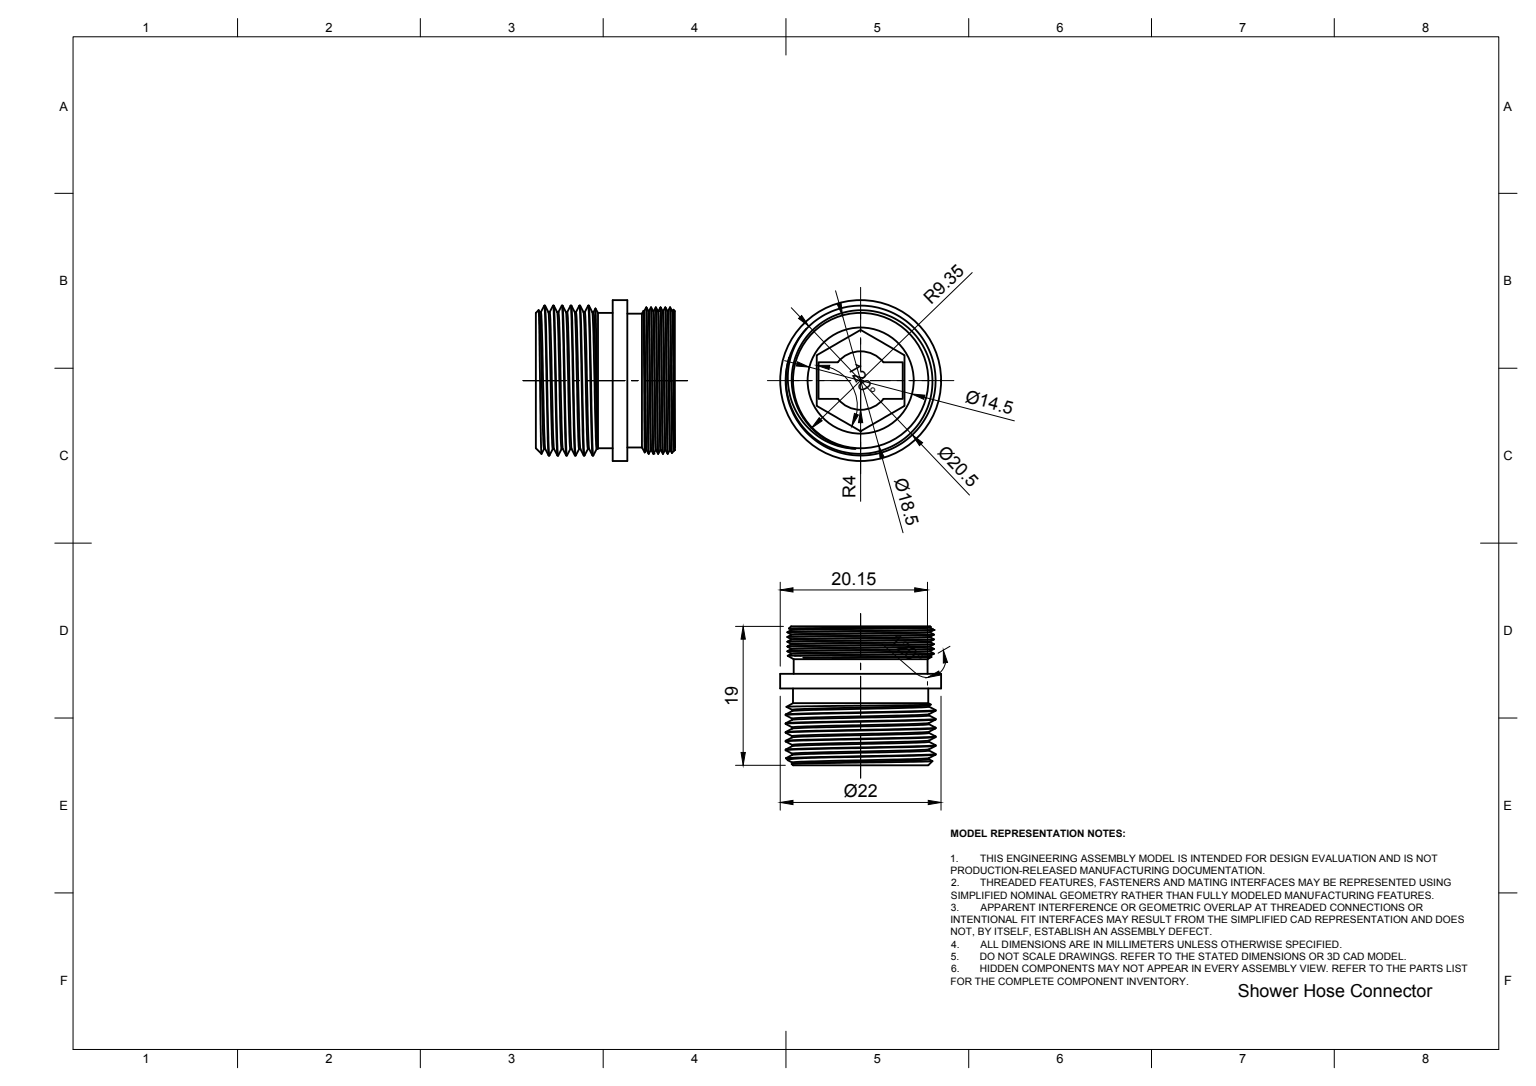
ISO-10303-21;
HEADER;
/* Generated by software containing ST-Developer
 * from STEP Tools, Inc. (www.steptools.com) 
 */

FILE_DESCRIPTION(
/* description */ ('STEP AP214'),
/* implementation_level */ '2;1');

FILE_NAME(
/* name */ 'Shower Hose Connector.step',
/* time_stamp */ '2026-10-05T23:18:41-07:00',
/* author */ (''),
/* organization */ (''),
/* preprocessor_version */ 'ST-DEVELOPER v20.2',
/* originating_system */ 'Autodesk Translation Framework v15.15.0.0',
/* authorisation */ '');

FILE_SCHEMA (('AUTOMOTIVE_DESIGN { 1 0 10303 214 3 1 1 }'));
ENDSEC;

DATA;
#10=MECHANICAL_DESIGN_GEOMETRIC_PRESENTATION_REPRESENTATION('',(#102),#221662);
#64=MANIFOLD_SOLID_BREP('Body1',#79324);
#76=SHAPE_REPRESENTATION_RELATIONSHIP('SRR','None',#221711,#89);
#89=ADVANCED_BREP_SHAPE_REPRESENTATION('',(#64),#221651);
#102=STYLED_ITEM('',(#221783),#64);
#179=B_SPLINE_SURFACE_WITH_KNOTS('',1,3,((#174040,#174041,#174042,#174043,
#174044,#174045,#174046,#174047,#174048,#174049,#174050,#174051,#174052,
#174053,#174054,#174055,#174056,#174057,#174058,#174059,#174060,#174061,
#174062,#174063,#174064,#174065,#174066,#174067,#174068,#174069,#174070,
#174071,#174072,#174073,#174074,#174075,#174076,#174077,#174078,#174079,
#174080,#174081,#174082,#174083,#174084,#174085,#174086,#174087,#174088,
#174089,#174090,#174091,#174092,#174093,#174094,#174095,#174096,#174097,
#174098,#174099,#174100,#174101,#174102,#174103,#174104,#174105,#174106),
(#174107,#174108,#174109,#174110,#174111,#174112,#174113,#174114,#174115,
#174116,#174117,#174118,#174119,#174120,#174121,#174122,#174123,#174124,
#174125,#174126,#174127,#174128,#174129,#174130,#174131,#174132,#174133,
#174134,#174135,#174136,#174137,#174138,#174139,#174140,#174141,#174142,
#174143,#174144,#174145,#174146,#174147,#174148,#174149,#174150,#174151,
#174152,#174153,#174154,#174155,#174156,#174157,#174158,#174159,#174160,
#174161,#174162,#174163,#174164,#174165,#174166,#174167,#174168,#174169,
#174170,#174171,#174172,#174173)),.UNSPECIFIED.,.F.,.F.,.F.,(2,2),(4,1,
1,1,1,1,1,1,1,1,1,1,1,1,1,1,1,1,1,1,1,1,1,1,1,1,1,1,1,1,1,1,1,1,1,1,1,1,
1,1,1,1,1,1,1,1,1,1,1,1,1,1,1,1,1,1,1,1,1,1,1,1,1,1,4),(0.,1.),(0.,0.0157026587679609,
0.0314053175359218,0.0471079763038827,0.0628106350718436,0.0785132938398045,
0.0942159526077654,0.109918611375726,0.125621270143687,0.141323928911648,
0.157026587679609,0.17272924644757,0.188431905215531,0.204134563983492,
0.219837222751453,0.235539881519413,0.251242540287374,0.266945199055335,
0.282647857823296,0.298350516591257,0.314053175359218,0.329755834127179,
0.34545849289514,0.361161151663101,0.376863810431061,0.392566469199022,
0.408269127966983,0.423971786734944,0.439674445502905,0.455377104270866,
0.471079763038827,0.486782421806788,0.502485080574749,0.518187739342709,
0.53389039811067,0.549593056878631,0.565295715646592,0.580998374414553,
0.596701033182514,0.612403691950475,0.628106350718436,0.643809009486397,
0.659511668254358,0.675214327022318,0.690916985790279,0.70661964455824,
0.722322303326201,0.738024962094162,0.753727620862123,0.769430279630084,
0.785132938398045,0.800835597166006,0.816538255933966,0.832240914701927,
0.847943573469888,0.863646232237849,0.87934889100581,0.895051549773771,
0.910754208541732,0.926456867309693,0.942159526077654,0.957862184845615,
0.973564843613575,0.989267502381536,1.),.UNSPECIFIED.);
#180=B_SPLINE_SURFACE_WITH_KNOTS('',1,3,((#174174,#174175,#174176,#174177,
#174178,#174179,#174180,#174181,#174182,#174183,#174184,#174185,#174186,
#174187,#174188,#174189,#174190,#174191,#174192,#174193,#174194,#174195,
#174196,#174197,#174198,#174199,#174200,#174201,#174202,#174203,#174204,
#174205,#174206,#174207,#174208,#174209,#174210,#174211,#174212,#174213,
#174214,#174215,#174216,#174217,#174218,#174219,#174220,#174221,#174222,
#174223,#174224,#174225,#174226,#174227,#174228,#174229,#174230,#174231,
#174232,#174233,#174234,#174235,#174236,#174237,#174238,#174239,#174240),
(#174241,#174242,#174243,#174244,#174245,#174246,#174247,#174248,#174249,
#174250,#174251,#174252,#174253,#174254,#174255,#174256,#174257,#174258,
#174259,#174260,#174261,#174262,#174263,#174264,#174265,#174266,#174267,
#174268,#174269,#174270,#174271,#174272,#174273,#174274,#174275,#174276,
#174277,#174278,#174279,#174280,#174281,#174282,#174283,#174284,#174285,
#174286,#174287,#174288,#174289,#174290,#174291,#174292,#174293,#174294,
#174295,#174296,#174297,#174298,#174299,#174300,#174301,#174302,#174303,
#174304,#174305,#174306,#174307)),.UNSPECIFIED.,.F.,.F.,.F.,(2,2),(4,1,
1,1,1,1,1,1,1,1,1,1,1,1,1,1,1,1,1,1,1,1,1,1,1,1,1,1,1,1,1,1,1,1,1,1,1,1,
1,1,1,1,1,1,1,1,1,1,1,1,1,1,1,1,1,1,1,1,1,1,1,1,1,1,4),(0.,1.),(0.,0.0157026587679609,
0.0314053175359218,0.0471079763038827,0.0628106350718436,0.0785132938398045,
0.0942159526077654,0.109918611375726,0.125621270143687,0.141323928911648,
0.157026587679609,0.17272924644757,0.188431905215531,0.204134563983492,
0.219837222751453,0.235539881519413,0.251242540287374,0.266945199055335,
0.282647857823296,0.298350516591257,0.314053175359218,0.329755834127179,
0.34545849289514,0.361161151663101,0.376863810431061,0.392566469199022,
0.408269127966983,0.423971786734944,0.439674445502905,0.455377104270866,
0.471079763038827,0.486782421806788,0.502485080574749,0.518187739342709,
0.53389039811067,0.549593056878631,0.565295715646592,0.580998374414553,
0.596701033182514,0.612403691950475,0.628106350718436,0.643809009486397,
0.659511668254358,0.675214327022318,0.690916985790279,0.70661964455824,
0.722322303326201,0.738024962094162,0.753727620862123,0.769430279630084,
0.785132938398045,0.800835597166006,0.816538255933966,0.832240914701927,
0.847943573469888,0.863646232237849,0.87934889100581,0.895051549773771,
0.910754208541732,0.926456867309693,0.942159526077654,0.957862184845615,
0.973564843613575,0.989267502381536,1.),.UNSPECIFIED.);
#181=B_SPLINE_SURFACE_WITH_KNOTS('',1,3,((#174308,#174309,#174310,#174311,
#174312,#174313,#174314,#174315,#174316,#174317,#174318,#174319,#174320,
#174321,#174322,#174323,#174324,#174325,#174326,#174327,#174328,#174329,
#174330,#174331,#174332,#174333,#174334,#174335,#174336,#174337,#174338,
#174339,#174340,#174341,#174342,#174343,#174344,#174345,#174346,#174347,
#174348,#174349,#174350,#174351,#174352,#174353,#174354,#174355,#174356,
#174357,#174358,#174359,#174360,#174361,#174362,#174363,#174364,#174365,
#174366,#174367,#174368,#174369,#174370,#174371,#174372,#174373,#174374,
#174375,#174376,#174377,#174378,#174379,#174380,#174381,#174382,#174383,
#174384),(#174385,#174386,#174387,#174388,#174389,#174390,#174391,#174392,
#174393,#174394,#174395,#174396,#174397,#174398,#174399,#174400,#174401,
#174402,#174403,#174404,#174405,#174406,#174407,#174408,#174409,#174410,
#174411,#174412,#174413,#174414,#174415,#174416,#174417,#174418,#174419,
#174420,#174421,#174422,#174423,#174424,#174425,#174426,#174427,#174428,
#174429,#174430,#174431,#174432,#174433,#174434,#174435,#174436,#174437,
#174438,#174439,#174440,#174441,#174442,#174443,#174444,#174445,#174446,
#174447,#174448,#174449,#174450,#174451,#174452,#174453,#174454,#174455,
#174456,#174457,#174458,#174459,#174460,#174461)),.UNSPECIFIED.,.F.,.F.,
 .F.,(2,2),(4,1,1,1,1,1,1,1,1,1,1,1,1,1,1,1,1,1,1,1,1,1,1,1,1,1,1,1,1,1,
1,1,1,1,1,1,1,1,1,1,1,1,1,1,1,1,1,1,1,1,1,1,1,1,1,1,1,1,1,1,1,1,1,1,1,1,
1,1,1,1,1,1,1,1,4),(0.,1.),(0.,0.0135337770704249,0.0270675541408498,0.0406013312112747,
0.0541351082816996,0.0676688853521246,0.0812026624225494,0.0947364394929744,
0.108270216563399,0.121803993633824,0.135337770704249,0.148871547774674,
0.162405324845099,0.175939101915524,0.189472878985949,0.203006656056374,
0.216540433126799,0.230074210197223,0.243607987267648,0.257141764338073,
0.270675541408498,0.284209318478923,0.297743095549348,0.311276872619773,
0.324810649690198,0.338344426760623,0.351878203831048,0.365411980901473,
0.378945757971897,0.392479535042322,0.406013312112747,0.419547089183172,
0.433080866253597,0.446614643324022,0.460148420394447,0.473682197464872,
0.487215974535297,0.500749751605722,0.514283528676147,0.527817305746571,
0.541351082816996,0.554884859887421,0.568418636957846,0.581952414028271,
0.595486191098696,0.609019968169121,0.622553745239546,0.636087522309971,
0.649621299380396,0.663155076450821,0.676688853521245,0.69022263059167,
0.703756407662095,0.71729018473252,0.730823961802945,0.74435773887337,0.757891515943795,
0.77142529301422,0.784959070084645,0.79849284715507,0.812026624225495,0.825560401295919,
0.839094178366344,0.852627955436769,0.866161732507194,0.879695509577619,
0.893229286648044,0.906763063718469,0.920296840788894,0.933830617859319,
0.947364394929744,0.960898172000169,0.974431949070593,0.987965726141018,
1.),.UNSPECIFIED.);
#182=B_SPLINE_SURFACE_WITH_KNOTS('',1,3,((#174462,#174463,#174464,#174465,
#174466,#174467,#174468,#174469,#174470,#174471,#174472,#174473,#174474,
#174475,#174476,#174477,#174478,#174479,#174480,#174481,#174482,#174483,
#174484,#174485,#174486,#174487,#174488,#174489,#174490,#174491,#174492,
#174493,#174494,#174495,#174496,#174497,#174498,#174499,#174500,#174501,
#174502,#174503,#174504,#174505,#174506,#174507,#174508,#174509,#174510,
#174511,#174512,#174513,#174514,#174515,#174516,#174517,#174518,#174519,
#174520,#174521,#174522,#174523,#174524,#174525,#174526,#174527,#174528,
#174529,#174530,#174531,#174532,#174533,#174534,#174535,#174536,#174537,
#174538),(#174539,#174540,#174541,#174542,#174543,#174544,#174545,#174546,
#174547,#174548,#174549,#174550,#174551,#174552,#174553,#174554,#174555,
#174556,#174557,#174558,#174559,#174560,#174561,#174562,#174563,#174564,
#174565,#174566,#174567,#174568,#174569,#174570,#174571,#174572,#174573,
#174574,#174575,#174576,#174577,#174578,#174579,#174580,#174581,#174582,
#174583,#174584,#174585,#174586,#174587,#174588,#174589,#174590,#174591,
#174592,#174593,#174594,#174595,#174596,#174597,#174598,#174599,#174600,
#174601,#174602,#174603,#174604,#174605,#174606,#174607,#174608,#174609,
#174610,#174611,#174612,#174613,#174614,#174615)),.UNSPECIFIED.,.F.,.F.,
 .F.,(2,2),(4,1,1,1,1,1,1,1,1,1,1,1,1,1,1,1,1,1,1,1,1,1,1,1,1,1,1,1,1,1,
1,1,1,1,1,1,1,1,1,1,1,1,1,1,1,1,1,1,1,1,1,1,1,1,1,1,1,1,1,1,1,1,1,1,1,1,
1,1,1,1,1,1,1,1,4),(0.,1.),(0.,0.0135337770704249,0.0270675541408498,0.0406013312112747,
0.0541351082816996,0.0676688853521246,0.0812026624225494,0.0947364394929744,
0.108270216563399,0.121803993633824,0.135337770704249,0.148871547774674,
0.162405324845099,0.175939101915524,0.189472878985949,0.203006656056374,
0.216540433126799,0.230074210197223,0.243607987267648,0.257141764338073,
0.270675541408498,0.284209318478923,0.297743095549348,0.311276872619773,
0.324810649690198,0.338344426760623,0.351878203831048,0.365411980901473,
0.378945757971897,0.392479535042322,0.406013312112747,0.419547089183172,
0.433080866253597,0.446614643324022,0.460148420394447,0.473682197464872,
0.487215974535297,0.500749751605722,0.514283528676147,0.527817305746571,
0.541351082816996,0.554884859887421,0.568418636957846,0.581952414028271,
0.595486191098696,0.609019968169121,0.622553745239546,0.636087522309971,
0.649621299380396,0.663155076450821,0.676688853521245,0.69022263059167,
0.703756407662095,0.71729018473252,0.730823961802945,0.74435773887337,0.757891515943795,
0.77142529301422,0.784959070084645,0.79849284715507,0.812026624225495,0.825560401295919,
0.839094178366344,0.852627955436769,0.866161732507194,0.879695509577619,
0.893229286648044,0.906763063718469,0.920296840788894,0.933830617859319,
0.947364394929744,0.960898172000169,0.974431949070593,0.987965726141018,
1.),.UNSPECIFIED.);
#275=FACE_BOUND('',#24701,.T.);
#276=FACE_BOUND('',#24703,.T.);
#277=FACE_BOUND('',#24705,.T.);
#278=FACE_BOUND('',#24713,.T.);
#279=FACE_BOUND('',#24715,.T.);
#280=FACE_BOUND('',#24717,.T.);
#281=FACE_BOUND('',#24719,.T.);
#1770=(
BOUNDED_CURVE()
B_SPLINE_CURVE(2,(#173205,#173206,#173207),.UNSPECIFIED.,.F.,.F.)
B_SPLINE_CURVE_WITH_KNOTS((3,3),(-1.84750056124993,-0.734340623816359),
 .UNSPECIFIED.)
CURVE()
GEOMETRIC_REPRESENTATION_ITEM()
RATIONAL_B_SPLINE_CURVE((1.51230430780121,1.74625859842863,1.51230430780121))
REPRESENTATION_ITEM('')
);
#1771=(
BOUNDED_CURVE()
B_SPLINE_CURVE(2,(#173209,#173210,#173211),.UNSPECIFIED.,.F.,.F.)
B_SPLINE_CURVE_WITH_KNOTS((3,3),(-1.84750056124992,-0.734340623816352),
 .UNSPECIFIED.)
CURVE()
GEOMETRIC_REPRESENTATION_ITEM()
RATIONAL_B_SPLINE_CURVE((1.51230430780122,1.74625859842863,1.51230430780121))
REPRESENTATION_ITEM('')
);
#1772=(
BOUNDED_CURVE()
B_SPLINE_CURVE(2,(#173213,#173214,#173215),.UNSPECIFIED.,.F.,.F.)
B_SPLINE_CURVE_WITH_KNOTS((3,3),(-1.84750056124992,-0.734340623816351),
 .UNSPECIFIED.)
CURVE()
GEOMETRIC_REPRESENTATION_ITEM()
RATIONAL_B_SPLINE_CURVE((1.51230430780122,1.74625859842864,1.51230430780121))
REPRESENTATION_ITEM('')
);
#1773=(
BOUNDED_CURVE()
B_SPLINE_CURVE(2,(#173220,#173221,#173222),.UNSPECIFIED.,.F.,.F.)
B_SPLINE_CURVE_WITH_KNOTS((3,3),(0.734340623816355,1.8475005612499),
 .UNSPECIFIED.)
CURVE()
GEOMETRIC_REPRESENTATION_ITEM()
RATIONAL_B_SPLINE_CURVE((1.5123043078012,1.7462585984286,1.5123043078012))
REPRESENTATION_ITEM('')
);
#1774=(
BOUNDED_CURVE()
B_SPLINE_CURVE(2,(#173224,#173225,#173226),.UNSPECIFIED.,.F.,.F.)
B_SPLINE_CURVE_WITH_KNOTS((3,3),(0.734340623816354,1.84750056124992),
 .UNSPECIFIED.)
CURVE()
GEOMETRIC_REPRESENTATION_ITEM()
RATIONAL_B_SPLINE_CURVE((1.51230430780121,1.74625859842862,1.51230430780121))
REPRESENTATION_ITEM('')
);
#1775=(
BOUNDED_CURVE()
B_SPLINE_CURVE(2,(#173227,#173228,#173229),.UNSPECIFIED.,.F.,.F.)
B_SPLINE_CURVE_WITH_KNOTS((3,3),(0.734340623816358,1.84750056124993),
 .UNSPECIFIED.)
CURVE()
GEOMETRIC_REPRESENTATION_ITEM()
RATIONAL_B_SPLINE_CURVE((1.51230430780122,1.74625859842864,1.51230430780122))
REPRESENTATION_ITEM('')
);
#1886=TOROIDAL_SURFACE('',#80583,6.75,0.25);
#1887=TOROIDAL_SURFACE('',#80586,8.25,0.5);
#1933=CONICAL_SURFACE('',#80540,9.49999999999999,0.7853981625);
#1934=CONICAL_SURFACE('',#80555,7.25,1.04719755);
#1935=CONICAL_SURFACE('',#80571,10.25,1.04719755);
#1936=CONICAL_SURFACE('',#80573,9.99999999999999,1.04719755);
#1937=CONICAL_SURFACE('',#80592,9.49999999999999,0.7853981625);
#1938=CONICAL_SURFACE('',#80594,10.25,0.7853981625);
#2170=CYLINDRICAL_SURFACE('',#80523,9.35);
#2171=CYLINDRICAL_SURFACE('',#80525,9.35);
#2172=CYLINDRICAL_SURFACE('',#80526,9.35);
#2173=CYLINDRICAL_SURFACE('',#80527,9.35);
#2174=CYLINDRICAL_SURFACE('',#80528,9.35);
#2175=CYLINDRICAL_SURFACE('',#80529,9.35);
#2176=CYLINDRICAL_SURFACE('',#80530,9.35);
#2177=CYLINDRICAL_SURFACE('',#80532,9.50000000000001);
#2178=CYLINDRICAL_SURFACE('',#80534,9.50000000000001);
#2179=CYLINDRICAL_SURFACE('',#80535,9.50000000000001);
#2180=CYLINDRICAL_SURFACE('',#80536,9.50000000000001);
#2181=CYLINDRICAL_SURFACE('',#80537,9.50000000000001);
#2182=CYLINDRICAL_SURFACE('',#80538,9.50000000000001);
#2183=CYLINDRICAL_SURFACE('',#80539,9.50000000000001);
#2184=CYLINDRICAL_SURFACE('',#80542,10.);
#2185=CYLINDRICAL_SURFACE('',#80544,10.);
#2186=CYLINDRICAL_SURFACE('',#80545,10.);
#2187=CYLINDRICAL_SURFACE('',#80546,10.);
#2188=CYLINDRICAL_SURFACE('',#80547,10.);
#2189=CYLINDRICAL_SURFACE('',#80548,10.25);
#2190=CYLINDRICAL_SURFACE('',#80550,10.25);
#2191=CYLINDRICAL_SURFACE('',#80551,10.25);
#2192=CYLINDRICAL_SURFACE('',#80552,10.25);
#2193=CYLINDRICAL_SURFACE('',#80553,10.25);
#2194=CYLINDRICAL_SURFACE('',#80554,10.25);
#2195=CYLINDRICAL_SURFACE('',#80557,10.25);
#2196=CYLINDRICAL_SURFACE('',#80559,9.25);
#2197=CYLINDRICAL_SURFACE('',#80563,11.);
#2198=CYLINDRICAL_SURFACE('',#80566,9.15);
#2199=CYLINDRICAL_SURFACE('',#80569,10.);
#2200=CYLINDRICAL_SURFACE('',#80576,7.75);
#2201=CYLINDRICAL_SURFACE('',#80580,6.5);
#2202=CYLINDRICAL_SURFACE('',#80589,4.);
#2203=CYLINDRICAL_SURFACE('',#80596,9.50000000000001);
#2204=CYLINDRICAL_SURFACE('',#80597,9.35);
#2205=CYLINDRICAL_SURFACE('',#80601,4.);
#3041=LINE('',#161941,#10108);
#3042=LINE('',#162330,#10109);
#3043=LINE('',#162956,#10110);
#3044=LINE('',#163166,#10111);
#3045=LINE('',#163572,#10112);
#3046=LINE('',#163993,#10113);
#3047=LINE('',#164421,#10114);
#3048=LINE('',#164833,#10115);
#3049=LINE('',#165106,#10116);
#3050=LINE('',#165636,#10117);
#3051=LINE('',#166150,#10118);
#3052=LINE('',#166686,#10119);
#3053=LINE('',#167210,#10120);
#3054=LINE('',#167730,#10121);
#3055=LINE('',#168256,#10122);
#3056=LINE('',#168283,#10123);
#3057=LINE('',#168630,#10124);
#3058=LINE('',#169158,#10125);
#3059=LINE('',#169674,#10126);
#3060=LINE('',#170192,#10127);
#3061=LINE('',#170718,#10128);
#3062=LINE('',#171017,#10129);
#3063=LINE('',#171447,#10130);
#3064=LINE('',#171891,#10131);
#3065=LINE('',#172549,#10132);
#3066=LINE('',#172769,#10133);
#3067=LINE('',#173217,#10134);
#3068=LINE('',#173296,#10135);
#3069=LINE('',#173304,#10136);
#3070=LINE('',#173310,#10137);
#3071=LINE('',#173726,#10138);
#3072=LINE('',#173793,#10139);
#3073=LINE('',#173799,#10140);
#3074=LINE('',#173806,#10141);
#3075=LINE('',#173821,#10142);
#3076=LINE('',#173824,#10143);
#3077=LINE('',#173948,#10144);
#3078=LINE('',#174618,#10145);
#3079=LINE('',#174620,#10146);
#3080=LINE('',#174621,#10147);
#3081=LINE('',#174624,#10148);
#3082=LINE('',#174626,#10149);
#3083=LINE('',#174627,#10150);
#3084=LINE('',#174630,#10151);
#3085=LINE('',#174632,#10152);
#3086=LINE('',#174633,#10153);
#3087=LINE('',#174638,#10154);
#3088=LINE('',#174642,#10155);
#3089=LINE('',#174644,#10156);
#3090=LINE('',#174645,#10157);
#3091=LINE('',#174648,#10158);
#3092=LINE('',#174650,#10159);
#3093=LINE('',#174651,#10160);
#3094=LINE('',#174653,#10161);
#3095=LINE('',#174654,#10162);
#3096=LINE('',#174660,#10163);
#3097=LINE('',#174662,#10164);
#3098=LINE('',#174664,#10165);
#3099=LINE('',#174666,#10166);
#3100=LINE('',#174668,#10167);
#3101=LINE('',#174669,#10168);
#3102=LINE('',#174671,#10169);
#3103=LINE('',#174672,#10170);
#3104=LINE('',#174674,#10171);
#3105=LINE('',#174676,#10172);
#3106=LINE('',#174678,#10173);
#3107=LINE('',#174680,#10174);
#10108=VECTOR('',#88588,9.35000000000001);
#10109=VECTOR('',#88593,9.35000000000001);
#10110=VECTOR('',#88596,9.35000000000001);
#10111=VECTOR('',#88599,9.35000000000001);
#10112=VECTOR('',#88602,9.35000000000001);
#10113=VECTOR('',#88605,9.35000000000001);
#10114=VECTOR('',#88608,9.35000000000001);
#10115=VECTOR('',#88613,9.50000000000001);
#10116=VECTOR('',#88618,9.50000000000001);
#10117=VECTOR('',#88621,9.50000000000001);
#10118=VECTOR('',#88624,9.50000000000001);
#10119=VECTOR('',#88627,9.50000000000001);
#10120=VECTOR('',#88630,9.50000000000001);
#10121=VECTOR('',#88633,9.50000000000001);
#10122=VECTOR('',#88636,9.5);
#10123=VECTOR('',#88641,10.);
#10124=VECTOR('',#88646,10.);
#10125=VECTOR('',#88649,10.);
#10126=VECTOR('',#88652,10.);
#10127=VECTOR('',#88655,10.);
#10128=VECTOR('',#88658,10.25);
#10129=VECTOR('',#88663,10.25);
#10130=VECTOR('',#88666,10.25);
#10131=VECTOR('',#88669,10.25);
#10132=VECTOR('',#88672,10.25);
#10133=VECTOR('',#88675,10.25);
#10134=VECTOR('',#88678,7.25);
#10135=VECTOR('',#88689,9.25000000000001);
#10136=VECTOR('',#88698,11.);
#10137=VECTOR('',#88705,9.15);
#10138=VECTOR('',#88716,10.25);
#10139=VECTOR('',#88723,9.99999999999999);
#10140=VECTOR('',#88728,7.75);
#10141=VECTOR('',#88737,6.5);
#10142=VECTOR('',#88756,1000.);
#10143=VECTOR('',#88759,1000.);
#10144=VECTOR('',#88766,10.25);
#10145=VECTOR('',#88775,1000.);
#10146=VECTOR('',#88776,1000.);
#10147=VECTOR('',#88777,1000.);
#10148=VECTOR('',#88780,1000.);
#10149=VECTOR('',#88781,1000.);
#10150=VECTOR('',#88782,1000.);
#10151=VECTOR('',#88785,1000.);
#10152=VECTOR('',#88786,1000.);
#10153=VECTOR('',#88787,1000.);
#10154=VECTOR('',#88792,1000.);
#10155=VECTOR('',#88797,1000.);
#10156=VECTOR('',#88798,1000.);
#10157=VECTOR('',#88799,1000.);
#10158=VECTOR('',#88802,1000.);
#10159=VECTOR('',#88803,1000.);
#10160=VECTOR('',#88804,1000.);
#10161=VECTOR('',#88807,1000.);
#10162=VECTOR('',#88808,1000.);
#10163=VECTOR('',#88815,1000.);
#10164=VECTOR('',#88816,1000.);
#10165=VECTOR('',#88817,1000.);
#10166=VECTOR('',#88818,1000.);
#10167=VECTOR('',#88819,1000.);
#10168=VECTOR('',#88820,1000.);
#10169=VECTOR('',#88823,1000.);
#10170=VECTOR('',#88824,1000.);
#10171=VECTOR('',#88827,1000.);
#10172=VECTOR('',#88830,1000.);
#10173=VECTOR('',#88833,1000.);
#10174=VECTOR('',#88836,1000.);
#16943=PLANE('',#80598);
#16944=PLANE('',#80599);
#16945=PLANE('',#80600);
#16946=PLANE('',#80604);
#16947=PLANE('',#80605);
#16948=PLANE('',#80606);
#16949=PLANE('',#80607);
#16950=PLANE('',#80608);
#16951=PLANE('',#80609);
#16952=PLANE('',#80610);
#16953=PLANE('',#80611);
#16954=PLANE('',#80612);
#16955=PLANE('',#80613);
#16956=PLANE('',#80614);
#16957=PLANE('',#80615);
#16958=PLANE('',#80616);
#16959=PLANE('',#80617);
#16960=PLANE('',#80618);
#16961=PLANE('',#80619);
#20601=FACE_OUTER_BOUND('',#24646,.T.);
#20602=FACE_OUTER_BOUND('',#24647,.T.);
#20603=FACE_OUTER_BOUND('',#24648,.T.);
#20604=FACE_OUTER_BOUND('',#24649,.T.);
#20605=FACE_OUTER_BOUND('',#24650,.T.);
#20606=FACE_OUTER_BOUND('',#24651,.T.);
#20607=FACE_OUTER_BOUND('',#24652,.T.);
#20608=FACE_OUTER_BOUND('',#24653,.T.);
#20609=FACE_OUTER_BOUND('',#24654,.T.);
#20610=FACE_OUTER_BOUND('',#24655,.T.);
#20611=FACE_OUTER_BOUND('',#24656,.T.);
#20612=FACE_OUTER_BOUND('',#24657,.T.);
#20613=FACE_OUTER_BOUND('',#24658,.T.);
#20614=FACE_OUTER_BOUND('',#24659,.T.);
#20615=FACE_OUTER_BOUND('',#24660,.T.);
#20616=FACE_OUTER_BOUND('',#24661,.T.);
#20617=FACE_OUTER_BOUND('',#24662,.T.);
#20618=FACE_OUTER_BOUND('',#24663,.T.);
#20619=FACE_OUTER_BOUND('',#24664,.T.);
#20620=FACE_OUTER_BOUND('',#24665,.T.);
#20621=FACE_OUTER_BOUND('',#24666,.T.);
#20622=FACE_OUTER_BOUND('',#24667,.T.);
#20623=FACE_OUTER_BOUND('',#24668,.T.);
#20624=FACE_OUTER_BOUND('',#24669,.T.);
#20625=FACE_OUTER_BOUND('',#24670,.T.);
#20626=FACE_OUTER_BOUND('',#24671,.T.);
#20627=FACE_OUTER_BOUND('',#24672,.T.);
#20628=FACE_OUTER_BOUND('',#24673,.T.);
#20629=FACE_OUTER_BOUND('',#24674,.T.);
#20630=FACE_OUTER_BOUND('',#24675,.T.);
#20631=FACE_OUTER_BOUND('',#24676,.T.);
#20632=FACE_OUTER_BOUND('',#24677,.T.);
#20633=FACE_OUTER_BOUND('',#24678,.T.);
#20634=FACE_OUTER_BOUND('',#24679,.T.);
#20635=FACE_OUTER_BOUND('',#24680,.T.);
#20636=FACE_OUTER_BOUND('',#24681,.T.);
#20637=FACE_OUTER_BOUND('',#24682,.T.);
#20638=FACE_OUTER_BOUND('',#24683,.T.);
#20639=FACE_OUTER_BOUND('',#24684,.T.);
#20640=FACE_OUTER_BOUND('',#24685,.T.);
#20641=FACE_OUTER_BOUND('',#24686,.T.);
#20642=FACE_OUTER_BOUND('',#24687,.T.);
#20643=FACE_OUTER_BOUND('',#24688,.T.);
#20644=FACE_OUTER_BOUND('',#24689,.T.);
#20645=FACE_OUTER_BOUND('',#24690,.T.);
#20646=FACE_OUTER_BOUND('',#24691,.T.);
#20647=FACE_OUTER_BOUND('',#24692,.T.);
#20648=FACE_OUTER_BOUND('',#24693,.T.);
#20649=FACE_OUTER_BOUND('',#24694,.T.);
#20650=FACE_OUTER_BOUND('',#24695,.T.);
#20651=FACE_OUTER_BOUND('',#24696,.T.);
#20652=FACE_OUTER_BOUND('',#24697,.T.);
#20653=FACE_OUTER_BOUND('',#24698,.T.);
#20654=FACE_OUTER_BOUND('',#24699,.T.);
#20655=FACE_OUTER_BOUND('',#24700,.T.);
#20656=FACE_OUTER_BOUND('',#24702,.T.);
#20657=FACE_OUTER_BOUND('',#24704,.T.);
#20658=FACE_OUTER_BOUND('',#24706,.T.);
#20659=FACE_OUTER_BOUND('',#24707,.T.);
#20660=FACE_OUTER_BOUND('',#24708,.T.);
#20661=FACE_OUTER_BOUND('',#24709,.T.);
#20662=FACE_OUTER_BOUND('',#24710,.T.);
#20663=FACE_OUTER_BOUND('',#24711,.T.);
#20664=FACE_OUTER_BOUND('',#24712,.T.);
#20665=FACE_OUTER_BOUND('',#24714,.T.);
#20666=FACE_OUTER_BOUND('',#24716,.T.);
#20667=FACE_OUTER_BOUND('',#24718,.T.);
#24646=EDGE_LOOP('',(#55947,#55948,#55949,#55950));
#24647=EDGE_LOOP('',(#55951,#55952,#55953,#55954));
#24648=EDGE_LOOP('',(#55955,#55956,#55957,#55958));
#24649=EDGE_LOOP('',(#55959,#55960,#55961,#55962));
#24650=EDGE_LOOP('',(#55963,#55964,#55965,#55966,#55967));
#24651=EDGE_LOOP('',(#55968,#55969,#55970,#55971));
#24652=EDGE_LOOP('',(#55972,#55973,#55974,#55975,#55976));
#24653=EDGE_LOOP('',(#55977,#55978,#55979,#55980));
#24654=EDGE_LOOP('',(#55981,#55982,#55983,#55984));
#24655=EDGE_LOOP('',(#55985,#55986,#55987,#55988));
#24656=EDGE_LOOP('',(#55989,#55990,#55991,#55992,#55993,#55994));
#24657=EDGE_LOOP('',(#55995,#55996,#55997,#55998));
#24658=EDGE_LOOP('',(#55999,#56000,#56001,#56002));
#24659=EDGE_LOOP('',(#56003,#56004,#56005,#56006));
#24660=EDGE_LOOP('',(#56007,#56008,#56009));
#24661=EDGE_LOOP('',(#56010,#56011,#56012,#56013));
#24662=EDGE_LOOP('',(#56014,#56015,#56016,#56017));
#24663=EDGE_LOOP('',(#56018,#56019,#56020,#56021));
#24664=EDGE_LOOP('',(#56022,#56023,#56024,#56025));
#24665=EDGE_LOOP('',(#56026,#56027,#56028,#56029));
#24666=EDGE_LOOP('',(#56030,#56031,#56032,#56033));
#24667=EDGE_LOOP('',(#56034,#56035,#56036,#56037));
#24668=EDGE_LOOP('',(#56038,#56039,#56040,#56041));
#24669=EDGE_LOOP('',(#56042,#56043,#56044,#56045));
#24670=EDGE_LOOP('',(#56046,#56047,#56048,#56049));
#24671=EDGE_LOOP('',(#56050,#56051,#56052,#56053));
#24672=EDGE_LOOP('',(#56054,#56055,#56056,#56057,#56058,#56059,#56060,#56061,
#56062));
#24673=EDGE_LOOP('',(#56063,#56064,#56065,#56066));
#24674=EDGE_LOOP('',(#56067,#56068,#56069,#56070,#56071));
#24675=EDGE_LOOP('',(#56072,#56073,#56074,#56075));
#24676=EDGE_LOOP('',(#56076,#56077,#56078,#56079));
#24677=EDGE_LOOP('',(#56080,#56081,#56082,#56083));
#24678=EDGE_LOOP('',(#56084,#56085,#56086,#56087,#56088,#56089,#56090,#56091,
#56092,#56093));
#24679=EDGE_LOOP('',(#56094,#56095,#56096,#56097,#56098,#56099,#56100,#56101));
#24680=EDGE_LOOP('',(#56102,#56103,#56104,#56105,#56106));
#24681=EDGE_LOOP('',(#56107,#56108,#56109,#56110));
#24682=EDGE_LOOP('',(#56111,#56112,#56113,#56114));
#24683=EDGE_LOOP('',(#56115,#56116,#56117,#56118,#56119));
#24684=EDGE_LOOP('',(#56120,#56121,#56122,#56123));
#24685=EDGE_LOOP('',(#56124,#56125,#56126,#56127,#56128));
#24686=EDGE_LOOP('',(#56129,#56130,#56131,#56132,#56133,#56134,#56135,#56136));
#24687=EDGE_LOOP('',(#56137,#56138,#56139,#56140));
#24688=EDGE_LOOP('',(#56141,#56142,#56143));
#24689=EDGE_LOOP('',(#56144,#56145,#56146,#56147,#56148,#56149,#56150,#56151,
#56152,#56153,#56154,#56155,#56156,#56157,#56158,#56159,#56160));
#24690=EDGE_LOOP('',(#56161,#56162,#56163,#56164,#56165,#56166,#56167,#56168,
#56169,#56170,#56171,#56172,#56173,#56174,#56175,#56176,#56177,#56178,#56179));
#24691=EDGE_LOOP('',(#56180,#56181,#56182,#56183,#56184,#56185,#56186,#56187,
#56188,#56189,#56190,#56191,#56192,#56193,#56194,#56195,#56196,#56197));
#24692=EDGE_LOOP('',(#56198,#56199,#56200,#56201,#56202,#56203,#56204,#56205,
#56206,#56207,#56208,#56209,#56210,#56211,#56212,#56213,#56214,#56215));
#24693=EDGE_LOOP('',(#56216,#56217,#56218,#56219));
#24694=EDGE_LOOP('',(#56220,#56221,#56222,#56223));
#24695=EDGE_LOOP('',(#56224,#56225,#56226,#56227));
#24696=EDGE_LOOP('',(#56228,#56229,#56230,#56231));
#24697=EDGE_LOOP('',(#56232,#56233,#56234,#56235));
#24698=EDGE_LOOP('',(#56236,#56237,#56238,#56239));
#24699=EDGE_LOOP('',(#56240,#56241,#56242,#56243));
#24700=EDGE_LOOP('',(#56244));
#24701=EDGE_LOOP('',(#56245,#56246,#56247,#56248,#56249,#56250,#56251,#56252));
#24702=EDGE_LOOP('',(#56253));
#24703=EDGE_LOOP('',(#56254));
#24704=EDGE_LOOP('',(#56255,#56256,#56257,#56258,#56259,#56260));
#24705=EDGE_LOOP('',(#56261,#56262,#56263,#56264,#56265,#56266,#56267,#56268));
#24706=EDGE_LOOP('',(#56269,#56270,#56271,#56272));
#24707=EDGE_LOOP('',(#56273,#56274,#56275,#56276));
#24708=EDGE_LOOP('',(#56277,#56278,#56279,#56280));
#24709=EDGE_LOOP('',(#56281,#56282,#56283,#56284));
#24710=EDGE_LOOP('',(#56285,#56286,#56287,#56288));
#24711=EDGE_LOOP('',(#56289,#56290,#56291,#56292));
#24712=EDGE_LOOP('',(#56293,#56294,#56295));
#24713=EDGE_LOOP('',(#56296));
#24714=EDGE_LOOP('',(#56297));
#24715=EDGE_LOOP('',(#56298));
#24716=EDGE_LOOP('',(#56299));
#24717=EDGE_LOOP('',(#56300));
#24718=EDGE_LOOP('',(#56301));
#24719=EDGE_LOOP('',(#56302));
#30123=B_SPLINE_CURVE_WITH_KNOTS('',3,(#161943,#161944,#161945,#161946,
#161947,#161948,#161949,#161950,#161951,#161952,#161953,#161954,#161955,
#161956,#161957,#161958,#161959,#161960,#161961,#161962,#161963,#161964,
#161965,#161966,#161967,#161968,#161969,#161970,#161971,#161972,#161973,
#161974,#161975,#161976,#161977,#161978,#161979,#161980,#161981,#161982,
#161983,#161984,#161985,#161986,#161987,#161988,#161989,#161990,#161991,
#161992,#161993,#161994,#161995,#161996,#161997,#161998,#161999,#162000,
#162001,#162002,#162003,#162004,#162005,#162006,#162007,#162008,#162009,
#162010,#162011,#162012,#162013,#162014,#162015,#162016,#162017,#162018,
#162019,#162020,#162021,#162022,#162023,#162024,#162025,#162026,#162027,
#162028,#162029,#162030,#162031,#162032,#162033,#162034,#162035,#162036,
#162037,#162038,#162039,#162040,#162041,#162042,#162043,#162044,#162045,
#162046,#162047,#162048,#162049,#162050,#162051,#162052,#162053,#162054,
#162055,#162056,#162057,#162058,#162059,#162060,#162061,#162062,#162063,
#162064,#162065,#162066,#162067,#162068,#162069,#162070,#162071,#162072,
#162073,#162074,#162075,#162076,#162077,#162078,#162079,#162080,#162081,
#162082,#162083,#162084,#162085,#162086,#162087,#162088,#162089,#162090,
#162091,#162092,#162093,#162094,#162095,#162096,#162097,#162098,#162099,
#162100,#162101,#162102,#162103,#162104,#162105,#162106,#162107,#162108,
#162109,#162110,#162111,#162112,#162113,#162114,#162115,#162116,#162117,
#162118,#162119,#162120,#162121,#162122,#162123,#162124,#162125,#162126,
#162127,#162128,#162129,#162130,#162131,#162132,#162133,#162134,#162135,
#162136,#162137,#162138,#162139,#162140,#162141,#162142,#162143,#162144),
 .UNSPECIFIED.,.F.,.F.,(4,2,2,2,2,2,2,2,2,2,2,2,2,2,2,2,2,2,2,2,2,2,2,2,
2,2,2,2,2,2,2,2,2,2,2,2,2,2,2,2,2,2,2,2,2,2,2,2,2,2,2,2,2,2,2,2,2,2,2,2,
2,2,2,2,2,2,2,2,2,2,2,2,2,2,2,2,2,2,2,2,2,2,2,2,2,2,2,2,2,2,2,2,2,2,2,2,
2,2,2,2,4),(-5.80673691874591,-5.80311558456603,-5.78521951548741,-5.74936542742757,
-5.69789658982925,-5.55469108508799,-5.47835921867039,-5.44224050505522,
-5.41337094993437,-5.37911111324198,-5.30769462254877,-5.19011243008685,
-5.1078364512622,-5.08324731886244,-5.06654399501397,-5.04601596685676,
-4.99854432371449,-4.91830532015885,-4.78499374848092,-4.74318259301805,
-4.71370033935409,-4.6823336174823,-4.6296968329514,-4.56208732768372,-4.47613359739696,
-4.38165464089175,-4.35365106186554,-4.33726741584425,-4.32077052078011,
-4.29220578521379,-4.19215569564271,-4.02482294360284,-3.9823839054569,
-3.9530819167607,-3.92201642443015,-3.8707363199192,-3.83543283172867,-3.71055225609258,
-3.63739932108507,-3.61332061828525,-3.59666780468482,-3.57581690019977,
-3.52601539924736,-3.4385685991293,-3.31662702727645,-3.27439545448113,
-3.24514210062318,-3.21398488565512,-3.16251724931886,-3.06903864772341,
-2.91054203146376,-2.88348211392876,-2.86728626244473,-2.85057629001149,
-2.82094837620054,-2.7817347539378,-2.67149231740343,-2.54909724995236,
-2.50941118672945,-2.48021170712932,-2.4480865615984,-2.39060713882964,
-2.31115601623141,-2.17122053541862,-2.14565849354444,-2.12883882530887,
-2.10884676183292,-2.06498560927209,-1.99486879103477,-1.8440265326523,
-1.80321525945184,-1.77387759557024,-1.74217324047111,-1.68763358136074,
-1.6163625826057,-1.51764607929113,-1.4347617200489,-1.4110028515639,-1.39555525777792,
-1.37784773159648,-1.34302416000173,-1.29369949695151,-1.19799736808929,
-1.07974823682673,-1.04009726750669,-1.01090298265717,-0.978763975383292,
-0.921197537526748,-0.841549942479151,-0.701890581981484,-0.676365628406667,
-0.659551239060342,-0.639541471368818,-0.595562919387754,-0.525133199857429,
-0.374882540968986,-0.334029316432046,-0.304686498507445,-0.272998728748237,
-0.218549124060644,-1.00000001435063E-6),.UNSPECIFIED.);
#30124=B_SPLINE_CURVE_WITH_KNOTS('',3,(#162147,#162148,#162149,#162150,
#162151,#162152,#162153,#162154,#162155,#162156,#162157,#162158,#162159,
#162160,#162161,#162162,#162163,#162164,#162165,#162166,#162167,#162168,
#162169,#162170,#162171,#162172,#162173,#162174,#162175,#162176,#162177,
#162178,#162179,#162180,#162181,#162182,#162183,#162184,#162185,#162186,
#162187,#162188,#162189,#162190,#162191,#162192,#162193,#162194,#162195,
#162196,#162197,#162198,#162199,#162200,#162201,#162202,#162203,#162204,
#162205,#162206,#162207,#162208,#162209,#162210,#162211,#162212,#162213,
#162214,#162215,#162216,#162217,#162218,#162219,#162220,#162221,#162222,
#162223,#162224,#162225,#162226,#162227,#162228,#162229,#162230,#162231,
#162232,#162233,#162234,#162235,#162236,#162237,#162238,#162239,#162240,
#162241,#162242,#162243,#162244,#162245,#162246,#162247,#162248,#162249,
#162250,#162251,#162252,#162253,#162254,#162255,#162256,#162257,#162258,
#162259,#162260,#162261,#162262,#162263,#162264,#162265,#162266,#162267,
#162268,#162269,#162270,#162271,#162272,#162273,#162274,#162275,#162276,
#162277,#162278,#162279,#162280,#162281,#162282,#162283,#162284,#162285,
#162286,#162287,#162288,#162289,#162290,#162291,#162292,#162293,#162294,
#162295,#162296,#162297,#162298,#162299,#162300,#162301,#162302,#162303,
#162304,#162305,#162306,#162307,#162308,#162309,#162310,#162311,#162312,
#162313,#162314,#162315,#162316,#162317,#162318,#162319,#162320,#162321,
#162322,#162323,#162324,#162325,#162326),.UNSPECIFIED.,.F.,.F.,(4,2,2,2,
2,2,2,2,2,2,2,2,2,2,2,2,2,2,2,2,2,2,2,2,2,2,2,2,2,2,2,2,2,2,2,2,2,2,2,2,
2,2,2,2,2,2,2,2,2,2,2,2,2,2,2,2,2,2,2,2,2,2,2,2,2,2,2,2,2,2,2,2,2,2,2,2,
2,2,2,2,2,2,2,2,2,2,2,2,2,4),(-28.462078608473,-28.3866548311619,-28.3415640456688,
-28.3139836013474,-28.2851402865027,-28.2498725241615,-28.1727391509134,
-28.0276202040923,-27.9762895199563,-27.9405029136976,-27.9226205962435,
-27.9070576963559,-27.8835404957315,-27.799784969196,-27.7010835025185,
-27.6300241283045,-27.5755935925949,-27.5439101464897,-27.5145673445461,
-27.4737074668686,-27.3235559695455,-27.2530676138123,-27.2090677021112,
-27.1890551445635,-27.1722423347026,-27.1467255074532,-27.0071246534371,
-26.9274530031814,-26.8698765206144,-26.8377367496269,-26.8085440961376,
-26.7688990369699,-26.6510052576259,-26.5570035453015,-26.5064981574161,
-26.4711052813981,-26.4532940091875,-26.4378833110121,-26.4143654381337,
-26.3306061123437,-26.2319014706414,-26.1608403040848,-26.1064082708122,
-26.0747238510428,-26.045380088863,-26.0045187746979,-25.85436419259,-25.7838726296274,
-25.7398709498093,-25.7198576946395,-25.7030443585834,-25.6775268190117,
-25.5379220805613,-25.4582473970294,-25.4006688534241,-25.3685280144069,
-25.3393344329808,-25.2996881799948,-25.1817954462825,-25.0878143825943,
-25.0372910199182,-25.0018891637963,-24.9840758916647,-24.9686651747599,
-24.9451497507252,-24.8613357356013,-24.7626277773463,-24.6915881953645,
-24.6371666422563,-24.6054833705243,-24.5761378290026,-24.535269208448,
-24.3851947435507,-24.3146549163278,-24.2706345365833,-24.2506179801848,
-24.2338047935297,-24.2082916912617,-24.0687112068533,-23.9890112592286,
-23.931420751605,-23.8992771939593,-23.8700831671917,-23.8304394951872,
-23.7127704669023,-23.6199974742871,-23.5686447890576,-23.5328466286805,
-23.5149611243724,-23.511361333244),.UNSPECIFIED.);
#30125=B_SPLINE_CURVE_WITH_KNOTS('',3,(#162331,#162332,#162333,#162334,
#162335,#162336,#162337,#162338,#162339,#162340,#162341,#162342,#162343,
#162344,#162345,#162346,#162347,#162348,#162349,#162350,#162351,#162352,
#162353,#162354,#162355,#162356,#162357,#162358,#162359,#162360,#162361,
#162362,#162363,#162364,#162365,#162366,#162367,#162368,#162369,#162370,
#162371,#162372,#162373,#162374,#162375,#162376,#162377,#162378,#162379,
#162380,#162381,#162382,#162383,#162384,#162385,#162386,#162387,#162388,
#162389,#162390,#162391,#162392,#162393,#162394,#162395,#162396,#162397,
#162398,#162399,#162400,#162401,#162402,#162403,#162404,#162405,#162406,
#162407,#162408,#162409,#162410,#162411,#162412,#162413,#162414,#162415,
#162416,#162417,#162418,#162419,#162420,#162421,#162422,#162423,#162424,
#162425,#162426,#162427,#162428,#162429,#162430,#162431,#162432,#162433,
#162434,#162435,#162436,#162437,#162438,#162439,#162440,#162441,#162442,
#162443,#162444,#162445,#162446,#162447,#162448,#162449,#162450,#162451,
#162452,#162453,#162454,#162455,#162456,#162457,#162458,#162459,#162460,
#162461,#162462,#162463,#162464,#162465,#162466,#162467,#162468,#162469,
#162470,#162471,#162472,#162473,#162474,#162475,#162476,#162477,#162478,
#162479,#162480,#162481,#162482,#162483,#162484,#162485,#162486,#162487,
#162488,#162489,#162490,#162491,#162492,#162493,#162494,#162495,#162496,
#162497,#162498,#162499,#162500,#162501,#162502,#162503,#162504,#162505,
#162506,#162507,#162508,#162509,#162510,#162511,#162512,#162513,#162514,
#162515,#162516,#162517,#162518,#162519,#162520,#162521,#162522,#162523,
#162524,#162525,#162526,#162527,#162528,#162529,#162530,#162531,#162532,
#162533,#162534,#162535,#162536,#162537,#162538),.UNSPECIFIED.,.F.,.F.,
(4,2,2,2,2,2,2,2,2,2,2,2,2,2,2,2,2,2,2,2,2,2,2,2,2,2,2,2,2,2,2,2,2,2,2,
2,2,2,2,2,2,2,2,2,2,2,2,2,2,2,2,2,2,2,2,2,2,2,2,2,2,2,2,2,2,2,2,2,2,2,2,
2,2,2,2,2,2,2,2,2,2,2,2,2,2,2,2,2,2,2,2,2,2,2,2,2,2,2,2,2,2,2,2,4),(-11.684044174322,
-11.6723367729996,-11.6578121804501,-11.6213110169713,-11.4659961518821,
-11.3949588913602,-11.3405391976892,-11.3088570747923,-11.2795126353998,
-11.2386456144045,-11.0885755866662,-11.0180390006996,-10.9740204899463,
-10.9540047134165,-10.9371921425277,-10.9116799180412,-10.772104244175,
-10.6924075600857,-10.6348193273248,-10.602676986944,-10.5734840389483,
-10.5338417896757,-10.416174179528,-10.3233755606539,-10.2720432235089,
-10.2362551585611,-10.2183719028399,-10.2028080433849,-10.1792891894372,
-10.0955321491061,-9.99682485798081,-9.92575976392989,-9.87132523251124,
-9.8396397759129,-9.81029529297017,-9.76943338184275,-9.61926762710395,
-9.54877801758719,-9.50477660009966,-9.48476302813906,-9.46794918087568,
-9.44243051234741,-9.30281954225911,-9.22314464713178,-9.16556541387518,
-9.13342385207994,-9.10422944144975,-9.064581790491,-8.94666604649448,-8.85258545643525,
-8.80212773470256,-8.76675706925275,-8.74894916912009,-8.73353607961527,
-8.71000687037493,-8.62634021065093,-8.52762996553284,-8.4565241472155,
-8.40206817624361,-8.37037821353963,-8.34103413103857,-8.30018054264639,
-8.14987483177597,-8.07945594751373,-8.03548056449599,-8.01547057214582,
-7.99865508565373,-7.9731272329097,-7.83346309061008,-7.75382343831422,
-7.69625920008055,-7.6641194132818,-7.6349232418721,-7.59526788858234,-7.47694539865929,
-7.36353796539349,-7.32380079443192,-7.29388946418653,-7.27712283294249,
-7.26097107435698,-7.23413817200323,-7.07433090077473,-6.98158545707883,
-6.93020696410078,-6.89906512256474,-6.86980261427119,-6.82751420994756,
-6.70813042045763,-6.61894713689106,-6.56861078422214,-6.54768760660895,
-6.53104358260768,-6.50707032200526,-6.42785900488293,-6.30717218959642,
-6.27246012230937,-6.2217530119573,-6.19078642066411,-6.16142784615645,
-6.11862909549268,-5.93063288332504,-5.84217227257886,-5.81867682705061,
-5.80673691874591),.UNSPECIFIED.);
#30126=B_SPLINE_CURVE_WITH_KNOTS('',3,(#162539,#162540,#162541,#162542,
#162543,#162544,#162545,#162546,#162547,#162548,#162549,#162550,#162551,
#162552,#162553,#162554,#162555,#162556,#162557,#162558,#162559,#162560,
#162561,#162562,#162563,#162564,#162565,#162566,#162567,#162568,#162569,
#162570,#162571,#162572,#162573,#162574,#162575,#162576,#162577,#162578,
#162579,#162580,#162581,#162582,#162583,#162584,#162585,#162586,#162587,
#162588,#162589,#162590,#162591,#162592,#162593,#162594,#162595,#162596,
#162597,#162598,#162599,#162600,#162601,#162602,#162603,#162604,#162605,
#162606,#162607,#162608,#162609,#162610,#162611,#162612,#162613,#162614,
#162615,#162616,#162617,#162618,#162619,#162620,#162621,#162622,#162623,
#162624,#162625,#162626,#162627,#162628,#162629,#162630,#162631,#162632,
#162633,#162634,#162635,#162636,#162637,#162638,#162639,#162640,#162641,
#162642,#162643,#162644,#162645,#162646,#162647,#162648,#162649,#162650,
#162651,#162652,#162653,#162654,#162655,#162656,#162657,#162658,#162659,
#162660,#162661,#162662,#162663,#162664,#162665,#162666,#162667,#162668,
#162669,#162670,#162671,#162672,#162673,#162674,#162675,#162676,#162677,
#162678,#162679,#162680,#162681,#162682,#162683,#162684,#162685,#162686,
#162687,#162688,#162689,#162690,#162691,#162692,#162693,#162694,#162695,
#162696,#162697,#162698,#162699,#162700,#162701,#162702,#162703,#162704,
#162705,#162706,#162707,#162708,#162709,#162710,#162711,#162712,#162713,
#162714,#162715,#162716,#162717,#162718,#162719,#162720,#162721,#162722,
#162723,#162724,#162725,#162726,#162727,#162728,#162729,#162730,#162731,
#162732,#162733,#162734,#162735,#162736,#162737,#162738,#162739,#162740,
#162741,#162742,#162743,#162744),.UNSPECIFIED.,.F.,.F.,(4,2,2,2,2,2,2,2,
2,2,2,2,2,2,2,2,2,2,2,2,2,2,2,2,2,2,2,2,2,2,2,2,2,2,2,2,2,2,2,2,2,2,2,2,
2,2,2,2,2,2,2,2,2,2,2,2,2,2,2,2,2,2,2,2,2,2,2,2,2,2,2,2,2,2,2,2,2,2,2,2,
2,2,2,2,2,2,2,2,2,2,2,2,2,2,2,2,2,2,2,2,2,2,4),(-23.511361333244,-23.4993972146998,
-23.4758809979245,-23.3920650137635,-23.2933538790571,-23.222311663882,
-23.1678881812097,-23.1362038578463,-23.1068573834604,-23.0659875336822,
-22.9159070008107,-22.8453655716136,-22.8013440258702,-22.7813268635726,
-22.7645131254748,-22.7389991251823,-22.5994137366634,-22.5197115478179,
-22.4621193305488,-22.4299747619663,-22.4007797880389,-22.3611347842271,
-22.2434587686312,-22.1506513293291,-22.0993169410328,-22.0635271110743,
-22.0456427443577,-22.0300777615743,-22.0065569877358,-21.9227978044795,
-21.8240836745711,-21.7530120351075,-21.6985728996921,-21.6668850982125,
-21.6375386358784,-21.5966742949601,-21.4464924060745,-21.3760009976888,
-21.3319976895833,-21.3119829078351,-21.2951678475892,-21.2696470548108,
-21.1300244121076,-21.0503455467186,-20.9927630125642,-20.9606193364621,
-20.9314228664848,-20.8917722001421,-20.7738322732462,-20.6796670929825,
-20.629259794319,-20.593912562184,-20.5761081420522,-20.5606923997099,-20.5371509363203,
-20.4535496666785,-20.3548327100082,-20.2836961859723,-20.2292232392401,
-20.1975287401617,-20.1681835203225,-20.1273335473972,-19.9769278678421,
-19.906552344578,-19.862592066368,-19.8425834801576,-19.8257660978533,-19.8002309315131,
-19.6605226063899,-19.5809037486191,-19.5233472487528,-19.4912071878676,
-19.46200841687,-19.4223458305632,-19.2344315517932,-19.1392170953403,-19.1154216534419,
-19.0998135406436,-19.0820475230388,-19.046913153152,-18.9069936528118,
-18.8239247364213,-18.7636645823629,-18.730965971671,-18.7019078955318,
-18.6640356065842,-18.5570298547274,-18.4687890467565,-18.4216257184478,
-18.3876755479274,-18.3693757380058,-18.3538804018095,-18.3259541867317,
-18.1495305957111,-18.0659447479598,-18.030177836169,-18.0013209655792,
-17.9667538391989,-17.8946472335103,-17.7511154568425,-17.6684221208536,
-17.6452400522391,-17.6336516764103),.UNSPECIFIED.);
#30127=B_SPLINE_CURVE_WITH_KNOTS('',3,(#162747,#162748,#162749,#162750,
#162751,#162752,#162753,#162754,#162755,#162756,#162757,#162758,#162759,
#162760,#162761,#162762,#162763,#162764,#162765,#162766,#162767,#162768,
#162769,#162770,#162771,#162772,#162773,#162774,#162775,#162776,#162777,
#162778,#162779,#162780,#162781,#162782,#162783,#162784,#162785,#162786,
#162787,#162788,#162789,#162790,#162791,#162792,#162793,#162794,#162795,
#162796,#162797,#162798,#162799,#162800,#162801,#162802,#162803,#162804,
#162805,#162806,#162807,#162808,#162809,#162810,#162811,#162812,#162813,
#162814,#162815,#162816,#162817,#162818,#162819,#162820,#162821,#162822,
#162823,#162824,#162825,#162826,#162827,#162828,#162829,#162830,#162831,
#162832,#162833,#162834,#162835,#162836,#162837,#162838,#162839,#162840,
#162841,#162842,#162843,#162844,#162845,#162846,#162847,#162848,#162849,
#162850,#162851,#162852,#162853,#162854,#162855,#162856,#162857,#162858,
#162859,#162860,#162861,#162862,#162863,#162864,#162865,#162866,#162867,
#162868,#162869,#162870,#162871,#162872,#162873,#162874,#162875,#162876,
#162877,#162878,#162879,#162880,#162881,#162882,#162883,#162884,#162885,
#162886,#162887,#162888,#162889,#162890,#162891,#162892,#162893,#162894,
#162895,#162896,#162897,#162898,#162899,#162900,#162901,#162902,#162903,
#162904,#162905,#162906,#162907,#162908,#162909,#162910,#162911,#162912,
#162913,#162914,#162915,#162916,#162917,#162918,#162919,#162920,#162921,
#162922,#162923,#162924,#162925,#162926,#162927,#162928,#162929,#162930,
#162931,#162932,#162933,#162934,#162935,#162936,#162937,#162938,#162939,
#162940,#162941,#162942,#162943,#162944,#162945,#162946,#162947,#162948,
#162949,#162950,#162951,#162952,#162953,#162954),.UNSPECIFIED.,.F.,.F.,
(4,2,2,2,2,2,2,2,2,2,2,2,2,2,2,2,2,2,2,2,2,2,2,2,2,2,2,2,2,2,2,2,2,2,2,
2,2,2,2,2,2,2,2,2,2,2,2,2,2,2,2,2,2,2,2,2,2,2,2,2,2,2,2,2,2,2,2,2,2,2,2,
2,2,2,2,2,2,2,2,2,2,2,2,2,2,2,2,2,2,2,2,2,2,2,2,2,2,2,2,2,2,2,2,4),(-17.6336516764103,
-17.6297243330596,-17.6116808244776,-17.5750059161433,-17.4367864941327,
-17.3541262239905,-17.2940543692883,-17.2613882223578,-17.2323243674471,
-17.1943943599489,-17.0846814014701,-16.9816201130654,-16.927367862535,
-16.9059448670352,-16.8893486613693,-16.8660531557983,-16.7953573344822,
-16.7864150354094,-16.6649414585775,-16.630115600003,-16.5792969587153,
-16.5483100156811,-16.5189610220922,-16.4762299426034,-16.3119485845575,
-16.2098416083641,-16.1810552057561,-16.1645128975227,-16.1481695117954,
-16.1203707252606,-15.9660810541342,-15.8691700519801,-15.8180199551347,
-15.7869176839933,-15.7576318254445,-15.7151968440132,-15.6025722476219,
-15.5087784758488,-15.4570725237245,-15.4359686611406,-15.419344216166,
-15.3956253670958,-15.3202983293306,-15.1964086399864,-15.1612416528181,
-15.1100918324008,-15.0790470775991,-15.0497297623631,-15.0072044449991,
-14.8406561679522,-14.7400623849715,-14.7114372462249,-14.6949272684309,
-14.6805627321891,-14.654893180657,-14.50694225317,-14.3855500321139,-14.3415261726698,
-14.3116722146673,-14.2809387669368,-14.2315816356588,-14.1688167976056,
-14.0691049340051,-13.9938446919914,-13.9701305813156,-13.9535065294856,
-13.9323991956418,-13.880665938317,-13.7867761558958,-13.6743063607204,
-13.631870689576,-13.6025846942315,-13.5714824819395,-13.5203332368778,
-13.4233565715843,-13.2691331244168,-13.2413190829432,-13.2249726282854,
-13.2084334966322,-13.1796632703288,-13.077707529614,-12.9132272038271,
-12.8705149485744,-12.8411688075139,-12.8101764854403,-12.7593277508794,
-12.7244708632311,-12.6027868669078,-12.5586556269274,-12.5149929475945,
-12.4950303927588,-12.4782009101954,-12.4525739862569,-12.4208646084837,
-12.3484411713795,-12.2017213702071,-12.1606457739916,-12.1312685777191,
-12.099653925335,-12.0456331388895,-11.8143378152777,-11.7775768940125,
-11.7595172858016,-11.7555598459133),.UNSPECIFIED.);
#30128=B_SPLINE_CURVE_WITH_KNOTS('',3,(#162957,#162958,#162959,#162960,
#162961,#162962,#162963,#162964,#162965,#162966,#162967,#162968,#162969,
#162970,#162971,#162972,#162973,#162974,#162975,#162976,#162977,#162978,
#162979,#162980,#162981,#162982,#162983,#162984,#162985,#162986,#162987,
#162988,#162989,#162990,#162991,#162992,#162993,#162994,#162995,#162996,
#162997,#162998,#162999,#163000,#163001,#163002,#163003,#163004,#163005,
#163006,#163007,#163008,#163009,#163010,#163011,#163012,#163013,#163014,
#163015,#163016,#163017,#163018,#163019,#163020,#163021,#163022,#163023,
#163024,#163025,#163026,#163027,#163028,#163029,#163030,#163031,#163032,
#163033,#163034,#163035,#163036,#163037,#163038,#163039,#163040,#163041,
#163042,#163043,#163044,#163045,#163046,#163047,#163048,#163049,#163050,
#163051,#163052,#163053,#163054,#163055,#163056,#163057,#163058,#163059,
#163060,#163061,#163062,#163063,#163064,#163065,#163066,#163067,#163068,
#163069,#163070,#163071,#163072,#163073,#163074,#163075,#163076,#163077,
#163078,#163079,#163080,#163081,#163082,#163083,#163084,#163085,#163086,
#163087,#163088,#163089,#163090,#163091,#163092,#163093,#163094,#163095,
#163096,#163097,#163098,#163099,#163100,#163101,#163102,#163103,#163104,
#163105,#163106,#163107,#163108,#163109,#163110,#163111,#163112,#163113,
#163114,#163115,#163116,#163117,#163118,#163119,#163120,#163121,#163122,
#163123,#163124,#163125,#163126,#163127,#163128,#163129,#163130,#163131,
#163132,#163133,#163134,#163135,#163136,#163137,#163138,#163139,#163140,
#163141,#163142,#163143,#163144,#163145,#163146,#163147,#163148,#163149,
#163150,#163151,#163152,#163153,#163154,#163155,#163156,#163157,#163158,
#163159,#163160,#163161,#163162),.UNSPECIFIED.,.F.,.F.,(4,2,2,2,2,2,2,2,
2,2,2,2,2,2,2,2,2,2,2,2,2,2,2,2,2,2,2,2,2,2,2,2,2,2,2,2,2,2,2,2,2,2,2,2,
2,2,2,2,2,2,2,2,2,2,2,2,2,2,2,2,2,2,2,2,2,2,2,2,2,2,2,2,2,2,2,2,2,2,2,2,
2,2,2,2,2,2,2,2,2,2,2,2,2,2,2,2,2,2,2,2,2,2,4),(-5.87747899666309,-5.87157346505971,
-5.85248314543527,-5.80954203483998,-5.7417957919028,-5.5608213270671,-5.5201349499391,
-5.49079992027863,-5.45907652088146,-5.40398214713538,-5.32972990832103,
-5.18388223059086,-5.15664816033201,-5.13974869721203,-5.12056346370538,
-5.08166576675479,-4.96471618283776,-4.84727000182852,-4.80935360609149,
-4.78029242579081,-4.74762140467953,-4.68751512230553,-4.60477716464133,
-4.46624328632409,-4.42985298043581,-4.4118607071297,-4.39633043336306,
-4.37304374410558,-4.28852092165992,-4.14412811602476,-4.0740255911769,
-4.03975577928991,-4.01116499979379,-3.97519554604315,-3.8897194987258,
-3.78910941156182,-3.70831001718957,-3.68410127974098,-3.66743607545008,
-3.64666970556103,-3.59749286246434,-3.51203828177267,-3.38728278927883,
-3.34503190946236,-3.31577494615111,-3.28462199156079,-3.23318206344992,
-3.14058837404119,-2.98069440326973,-2.95387314181897,-2.937723617619,-2.92095388779108,
-2.89102741751659,-2.85126289552927,-2.73768112991984,-2.61959869869359,
-2.5799480763157,-2.55075237876615,-2.51861023214061,-2.46103313057068,
-2.38136459778146,-2.24171758855171,-2.2161946518779,-2.19937971442438,
-2.17936694154875,-2.1353740560491,-2.06490903203982,-1.91470678954435,
-1.87384699542792,-1.84450183315419,-1.81281363412142,-1.75836912301625,
-1.68728513927099,-1.58856462092969,-1.50482238591236,-1.48129984342857,
-1.46573494246526,-1.44785213223697,-1.41206920115665,-1.36074929016381,
-1.26793889032233,-1.15027252609476,-1.11062990544292,-1.08143591754672,
-1.04929168040641,-0.99169818777239,-0.911991451022073,-0.772399803164502,
-0.746886891767463,-0.730073653166686,-0.710056749975434,-0.666034554412352,
-0.595490216808555,-0.445442481013401,-0.404573231916604,-0.375227423474463,
-0.343543965431134,-0.289122676732243,-0.21808301763149,-0.0627325530217655,
-0.02623614266319,-0.0117124008606042,-1.00000000102796E-6),
 .UNSPECIFIED.);
#30129=B_SPLINE_CURVE_WITH_KNOTS('',3,(#163167,#163168,#163169,#163170,
#163171,#163172,#163173,#163174,#163175,#163176,#163177,#163178,#163179,
#163180,#163181,#163182,#163183,#163184,#163185,#163186,#163187,#163188,
#163189,#163190,#163191,#163192,#163193,#163194,#163195,#163196,#163197,
#163198,#163199,#163200,#163201,#163202,#163203,#163204,#163205,#163206,
#163207,#163208,#163209,#163210,#163211,#163212,#163213,#163214,#163215,
#163216,#163217,#163218,#163219,#163220,#163221,#163222,#163223,#163224,
#163225,#163226,#163227,#163228,#163229,#163230,#163231,#163232,#163233,
#163234,#163235,#163236,#163237,#163238,#163239,#163240,#163241,#163242,
#163243,#163244,#163245,#163246,#163247,#163248,#163249,#163250,#163251,
#163252,#163253,#163254,#163255,#163256,#163257,#163258,#163259,#163260,
#163261,#163262,#163263,#163264,#163265,#163266,#163267,#163268,#163269,
#163270,#163271,#163272,#163273,#163274,#163275,#163276,#163277,#163278,
#163279,#163280,#163281,#163282,#163283,#163284,#163285,#163286,#163287,
#163288,#163289,#163290,#163291,#163292,#163293,#163294,#163295,#163296,
#163297,#163298,#163299,#163300,#163301,#163302,#163303,#163304,#163305,
#163306,#163307,#163308,#163309,#163310,#163311,#163312,#163313,#163314,
#163315,#163316,#163317,#163318,#163319,#163320,#163321,#163322,#163323,
#163324,#163325,#163326,#163327,#163328,#163329,#163330,#163331,#163332,
#163333,#163334,#163335,#163336,#163337,#163338,#163339,#163340,#163341,
#163342,#163343,#163344,#163345,#163346,#163347,#163348,#163349,#163350,
#163351,#163352,#163353,#163354,#163355,#163356,#163357,#163358,#163359,
#163360,#163361,#163362),.UNSPECIFIED.,.F.,.F.,(4,2,2,2,2,2,2,2,2,2,2,2,
2,2,2,2,2,2,2,2,2,2,2,2,2,2,2,2,2,2,2,2,2,2,2,2,2,2,2,2,2,2,2,2,2,2,2,2,
2,2,2,2,2,2,2,2,2,2,2,2,2,2,2,2,2,2,2,2,2,2,2,2,2,2,2,2,2,2,2,2,2,2,2,2,
2,2,2,2,2,2,2,2,2,2,2,2,2,4),(-11.7554193354896,-11.7397043632071,-11.7123004815342,
-11.6224226329561,-11.4373214846833,-11.3972516385993,-11.3680038502512,
-11.3360446056121,-11.2795437262896,-11.2022552555165,-11.0575886767294,
-11.0324815767214,-11.015720652302,-10.9954932470459,-10.950073918821,-10.8757255179483,
-10.7323508256304,-10.6911203504236,-10.6617252978838,-10.6301725220565,
-10.5764779266283,-10.3341276308243,-10.3038299096669,-10.2869872280702,
-10.2708941245356,-10.2443610789862,-10.1377258901351,-9.9739783796236,
-9.9312112972648,-9.90185904001811,-9.87088633993241,-9.82013679359398,
-9.78537996755567,-9.66438133917026,-9.58618606974665,-9.5619483554948,
-9.54528130209995,-9.52453598057058,-9.47550615798171,-9.39050927554147,
-9.26523325924768,-9.22293054516803,-9.19366725491827,-9.16253205978628,
-9.11118379427364,-8.86425618552492,-8.83412626996381,-8.81731620087078,
-8.80119737244526,-8.77453432150838,-8.66029891333827,-8.50548966811694,
-8.46221896920077,-8.43278589735234,-8.40194360743511,-8.35195177820095,
-8.28797649513853,-8.1881217207662,-8.11486396452449,-8.09140312005425,
-8.07479768206906,-8.0535049396504,-8.00030373832085,-7.90117681883251,
-7.78622750901807,-7.74828129370964,-7.71921680515702,-7.68656181833748,
-7.62654998195761,-7.54401711520464,-7.4063189996342,-7.36915394529351,
-7.3510242746613,-7.33553417289989,-7.31253040254177,-7.23269484403501,
-7.09052336097322,-7.01526138710406,-6.98024657890108,-6.9513993988035,
-6.91612418334169,-6.83681859754211,-6.68649309196766,-6.64000070015146,
-6.61881803077876,-6.60387345672411,-6.58153213344665,-6.51891702391052,
-6.37632972261265,-6.30508437756925,-6.27084803666434,-6.24197681600633,
-6.20582826182792,-6.12182666386515,-5.96475121216872,-5.90828696392928,
-5.88688495602323,-5.87747899666309),.UNSPECIFIED.);
#30130=B_SPLINE_CURVE_WITH_KNOTS('',3,(#163363,#163364,#163365,#163366,
#163367,#163368,#163369,#163370,#163371,#163372,#163373,#163374,#163375,
#163376,#163377,#163378,#163379,#163380,#163381,#163382,#163383,#163384,
#163385,#163386,#163387,#163388,#163389,#163390,#163391,#163392,#163393,
#163394,#163395,#163396,#163397,#163398,#163399,#163400,#163401,#163402,
#163403,#163404,#163405,#163406,#163407,#163408,#163409,#163410,#163411,
#163412,#163413,#163414,#163415,#163416,#163417,#163418,#163419,#163420,
#163421,#163422,#163423,#163424,#163425,#163426,#163427,#163428,#163429,
#163430,#163431,#163432,#163433,#163434,#163435,#163436,#163437,#163438,
#163439,#163440,#163441,#163442,#163443,#163444,#163445,#163446,#163447,
#163448,#163449,#163450,#163451,#163452,#163453,#163454,#163455,#163456,
#163457,#163458,#163459,#163460,#163461,#163462,#163463,#163464,#163465,
#163466,#163467,#163468,#163469,#163470,#163471,#163472,#163473,#163474,
#163475,#163476,#163477,#163478,#163479,#163480,#163481,#163482,#163483,
#163484,#163485,#163486,#163487,#163488,#163489,#163490,#163491,#163492,
#163493,#163494,#163495,#163496,#163497,#163498,#163499,#163500,#163501,
#163502,#163503,#163504,#163505,#163506,#163507,#163508,#163509,#163510,
#163511,#163512,#163513,#163514,#163515,#163516,#163517,#163518,#163519,
#163520,#163521,#163522,#163523,#163524,#163525,#163526,#163527,#163528,
#163529,#163530,#163531,#163532,#163533,#163534,#163535,#163536,#163537,
#163538,#163539,#163540,#163541,#163542,#163543,#163544,#163545,#163546,
#163547,#163548,#163549,#163550,#163551,#163552,#163553,#163554,#163555,
#163556,#163557,#163558,#163559,#163560,#163561,#163562,#163563,#163564,
#163565,#163566,#163567,#163568),.UNSPECIFIED.,.F.,.F.,(4,2,2,2,2,2,2,2,
2,2,2,2,2,2,2,2,2,2,2,2,2,2,2,2,2,2,2,2,2,2,2,2,2,2,2,2,2,2,2,2,2,2,2,2,
2,2,2,2,2,2,2,2,2,2,2,2,2,2,2,2,2,2,2,2,2,2,2,2,2,2,2,2,2,2,2,2,2,2,2,2,
2,2,2,2,2,2,2,2,2,2,2,2,2,2,2,2,2,2,2,2,2,2,4),(-11.7555598459133,-11.7440048067695,
-11.720851736883,-11.638659223459,-11.4953665694064,-11.4227083740445,-11.3880596555871,
-11.3592030410641,-11.3235236457627,-11.2407482262352,-11.0700802910848,
-11.0383780099431,-11.0205040090326,-11.0024721687282,-10.9699455702908,
-10.9256322936732,-10.7740119075505,-10.7099728002658,-10.6767884487821,
-10.6478103432566,-10.6101592509722,-10.5120284451198,-10.4250797153776,
-10.3301968685769,-10.3021758802065,-10.2857871637331,-10.2692906627363,
-10.2407356533069,-10.1407993755448,-9.97324266646984,-9.93081799300448,
-9.90151489474412,-9.87043899193725,-9.81911755145721,-9.78377384073625,
-9.65861981349754,-9.58575417153447,-9.56169656834753,-9.54504351230296,
-9.5241730780038,-9.47424208902618,-9.38638792719994,-9.26501304267273,
-9.22276472422519,-9.19350551792324,-9.16234684096919,-9.110888961732,-9.01770518171239,
-8.85868257304902,-8.8317053223883,-8.81552408718923,-8.79879050856922,
-8.76905203613641,-8.72963687788532,-8.61820280554415,-8.49733444467963,
-8.45764792686622,-8.42844487004975,-8.39631271403875,-8.3388109906517,
-8.25931711823037,-8.11940588144879,-8.09384484094786,-8.07702334324308,
-8.05702598803933,-8.01314304416159,-7.94297521434756,-7.79218740176557,
-7.75136442710309,-7.72202168256262,-7.69031479211883,-7.63577899031293,
-7.5645206967366,-7.46578969299074,-7.38269289579539,-7.35900554606823,
-7.34356717687921,-7.32582497937522,-7.29082160692587,-7.24112945306772,
-7.14593443646003,-7.02778013672203,-6.9881251327,-6.95892680798051,-6.92678233802362,
-6.86920288508827,-6.78953331989904,-6.64986690084062,-6.62434048946161,
-6.60752394225729,-6.58751010528971,-6.54351767881986,-6.4730578617152,
-6.32282194091014,-6.28196012859145,-6.25261265899417,-6.2209212087621,
-6.16646900481442,-6.09537301881674,-5.99664407705398,-5.91290865712216,
-5.88938277793605,-5.87740991053728),.UNSPECIFIED.);
#30131=B_SPLINE_CURVE_WITH_KNOTS('',3,(#163573,#163574,#163575,#163576,
#163577,#163578,#163579,#163580,#163581,#163582,#163583,#163584,#163585,
#163586,#163587,#163588,#163589,#163590,#163591,#163592,#163593,#163594,
#163595,#163596,#163597,#163598,#163599,#163600,#163601,#163602,#163603,
#163604,#163605,#163606,#163607,#163608,#163609,#163610,#163611,#163612,
#163613,#163614,#163615,#163616,#163617,#163618,#163619,#163620,#163621,
#163622,#163623,#163624,#163625,#163626,#163627,#163628,#163629,#163630,
#163631,#163632,#163633,#163634,#163635,#163636,#163637,#163638,#163639,
#163640,#163641,#163642,#163643,#163644,#163645,#163646,#163647,#163648,
#163649,#163650,#163651,#163652,#163653,#163654,#163655,#163656,#163657,
#163658,#163659,#163660,#163661,#163662,#163663,#163664,#163665,#163666,
#163667,#163668,#163669,#163670,#163671,#163672,#163673,#163674,#163675,
#163676,#163677,#163678,#163679,#163680,#163681,#163682,#163683,#163684,
#163685,#163686,#163687,#163688,#163689,#163690,#163691,#163692,#163693,
#163694,#163695,#163696,#163697,#163698,#163699,#163700,#163701,#163702,
#163703,#163704,#163705,#163706,#163707,#163708,#163709,#163710,#163711,
#163712,#163713,#163714,#163715,#163716,#163717,#163718,#163719,#163720,
#163721,#163722,#163723,#163724,#163725,#163726,#163727,#163728,#163729,
#163730,#163731,#163732,#163733,#163734,#163735,#163736,#163737,#163738,
#163739,#163740,#163741,#163742,#163743,#163744,#163745,#163746,#163747,
#163748,#163749,#163750,#163751,#163752,#163753,#163754,#163755,#163756,
#163757,#163758,#163759,#163760,#163761,#163762,#163763,#163764,#163765,
#163766,#163767,#163768,#163769,#163770,#163771,#163772),.UNSPECIFIED.,
 .F.,.F.,(4,2,2,2,2,2,2,2,2,2,2,2,2,2,2,2,2,2,2,2,2,2,2,2,2,2,2,2,2,2,2,
2,2,2,2,2,2,2,2,2,2,2,2,2,2,2,2,2,2,2,2,2,2,2,2,2,2,2,2,2,2,2,2,2,2,2,2,
2,2,2,2,2,2,2,2,2,2,2,2,2,2,2,2,2,2,2,2,2,2,2,2,2,2,2,2,2,2,2,2,4),(-17.6325413712744,
-17.6173187457267,-17.5904856539766,-17.4593952055629,-17.3626719016611,
-17.2965513353061,-17.2628975944784,-17.2339877545232,-17.1970562833595,
-17.1096153606531,-16.9866238803363,-16.9456921605042,-16.9149211009742,
-16.89722700416,-16.8790024480916,-16.8454419442937,-16.6774854446449,-16.5951359694173,
-16.5595115378792,-16.5306635546779,-16.4959833036162,-16.4230634716081,
-16.2799158071296,-16.1979903684606,-16.1748579249094,-16.159351597272,
-16.1412896347085,-16.1044983710977,-15.9664384603955,-15.8838265873493,
-15.8237812112649,-15.7911238400417,-15.762064995908,-15.7241374690325,
-15.6077611350589,-15.4903145511018,-15.4510846007422,-15.4318445322676,
-15.4149715433235,-15.387893779987,-15.2412814902409,-15.1673191911459,
-15.1123642372609,-15.0806678097385,-15.0513283384161,-15.0105871103192,
-14.8035043822286,-14.7516665127793,-14.7156392273614,-14.697713275884,
-14.6821643154854,-14.6587417864808,-14.5775135039217,-14.4344046562726,
-14.3622961518627,-14.3273191292728,-14.2984747582599,-14.2631678401768,
-14.1835735132702,-14.0317209167044,-13.9865811168811,-13.9656290196518,
-13.9489901467216,-13.925063527677,-13.8408484917158,-13.6623672802532,
-13.6250349005944,-13.5960376800389,-13.5630417581693,-13.5009852778125,
-13.4139140657653,-13.2642609992235,-13.2387213061367,-13.2243802532728,
-13.2078391596062,-13.1790510099162,-13.0769001636591,-12.9127536585608,
-12.8700218757182,-12.8406761560905,-12.8096957282282,-12.7588959517633,
-12.7240867360307,-12.6027175415787,-12.5250678189431,-12.5008241580527,
-12.484157186304,-12.4634173481096,-12.4144228007699,-12.3295333231515,
-12.2041551846857,-12.1618359118408,-12.1325711761753,-12.1014427265716,
-12.0501266293664,-11.9578768100303,-11.7971824674383,-11.770504412013,
-11.7559673807982,-11.7554193354896),.UNSPECIFIED.);
#30132=B_SPLINE_CURVE_WITH_KNOTS('',3,(#163774,#163775,#163776,#163777,
#163778,#163779,#163780,#163781,#163782,#163783,#163784,#163785,#163786,
#163787,#163788,#163789,#163790,#163791,#163792,#163793,#163794,#163795,
#163796,#163797,#163798,#163799,#163800,#163801,#163802,#163803,#163804,
#163805,#163806,#163807,#163808,#163809,#163810,#163811,#163812,#163813,
#163814,#163815,#163816,#163817,#163818,#163819,#163820,#163821,#163822,
#163823,#163824,#163825,#163826,#163827,#163828,#163829,#163830,#163831,
#163832,#163833,#163834,#163835,#163836,#163837,#163838,#163839,#163840,
#163841,#163842,#163843,#163844,#163845,#163846,#163847,#163848,#163849,
#163850,#163851,#163852,#163853,#163854,#163855,#163856,#163857,#163858,
#163859,#163860,#163861,#163862,#163863,#163864,#163865,#163866,#163867,
#163868,#163869,#163870,#163871,#163872,#163873,#163874,#163875,#163876,
#163877,#163878,#163879,#163880,#163881,#163882,#163883,#163884,#163885,
#163886,#163887,#163888,#163889,#163890,#163891,#163892,#163893,#163894,
#163895,#163896,#163897,#163898,#163899,#163900,#163901,#163902,#163903,
#163904,#163905,#163906,#163907,#163908,#163909,#163910,#163911,#163912,
#163913,#163914,#163915,#163916,#163917,#163918,#163919,#163920,#163921,
#163922,#163923,#163924,#163925,#163926,#163927,#163928,#163929,#163930,
#163931,#163932,#163933,#163934,#163935,#163936,#163937,#163938,#163939,
#163940,#163941,#163942,#163943,#163944,#163945,#163946,#163947,#163948,
#163949,#163950,#163951,#163952,#163953,#163954,#163955,#163956,#163957,
#163958,#163959,#163960,#163961,#163962,#163963,#163964,#163965,#163966,
#163967,#163968,#163969,#163970,#163971,#163972,#163973,#163974,#163975,
#163976,#163977,#163978,#163979,#163980,#163981,#163982,#163983,#163984,
#163985),.UNSPECIFIED.,.F.,.F.,(4,2,2,2,2,2,2,2,2,2,2,2,2,2,2,2,2,2,2,2,
2,2,2,2,2,2,2,2,2,2,2,2,2,2,2,2,2,2,2,2,2,2,2,2,2,2,2,2,2,2,2,2,2,2,2,2,
2,2,2,2,2,2,2,2,2,2,2,2,2,2,2,2,2,2,2,2,2,2,2,2,2,2,2,2,2,2,2,2,2,2,2,2,
2,2,2,2,2,2,2,2,2,2,2,2,2,4),(-5.87740991053728,-5.87381634389079,-5.85593259626545,
-5.82014988976725,-5.76883250195084,-5.67600323296091,-5.55832568302647,
-5.51867964714232,-5.4894831557696,-5.45733617317984,-5.39973779655696,
-5.32002434367809,-5.18042059592695,-5.1549054723282,-5.13809078986479,
-5.11807218524499,-5.07404630556962,-5.00349615672977,-4.8534351379586,
-4.812562417678,-4.78321409938624,-4.75152791616519,-4.69710190387738,-4.62605603914143,
-4.52732961968957,-4.44348970680189,-4.41997195299682,-4.4044070877698,
-4.38652049228867,-4.35072022791597,-4.29936522418603,-4.20660022685623,
-4.08893228353677,-4.04928748385735,-4.02009183715372,-3.98794572217029,
-3.93034870130074,-3.85063688066746,-3.71103790495148,-3.68552365771353,
-3.66870947346294,-3.64869136252443,-3.60466624131641,-3.53411678403665,
-3.38406246324267,-3.34319073573122,-3.31384322885109,-3.28215800891038,
-3.22773389296099,-3.15669072814478,-3.05796711401422,-2.97412817625273,
-2.95061115117794,-2.93519943267184,-2.91738499773655,-2.88198087389371,
-2.83145493570879,-2.73748120548732,-2.6195895690735,-2.57994205599912,
-2.55074675201768,-2.51860323799425,-2.46101795597002,-2.38133107091658,
-2.24170745971876,-2.21618866822998,-2.19937427274828,-2.17935940028968,
-2.13535287861461,-2.06485158880524,-1.91471635824081,-1.8738518013772,
-1.84450597083593,-1.81281948687812,-1.75838467887102,-1.68731964167472,
-1.58859899517801,-1.50481364012982,-1.48129449819807,-1.46573010873508,
-1.44784576290461,-1.41205434491034,-1.36071658586461,-1.26793430907094,
-1.15027077968689,-1.11062820157249,-1.08143421502927,-1.04928995090465,
-0.991696319260591,-0.911989278801862,-0.772397971886967,-0.746885124704753,
-0.730071892244856,-0.710054950998422,-0.666032522475088,-0.595487572620013,
-0.445440918675119,-0.404571584945724,-0.375225760690415,-0.343542325363129,
-0.289121185952612,-0.218081824129735,-0.0627285934085948,-0.0262342865270621,
-0.011711063373005,-1.00000000198032E-6),.UNSPECIFIED.);
#30133=B_SPLINE_CURVE_WITH_KNOTS('',3,(#163986,#163987,#163988,#163989),
 .UNSPECIFIED.,.F.,.F.,(4,4),(-12.3895192570164,-12.3895147069527),
 .UNSPECIFIED.);
#30134=B_SPLINE_CURVE_WITH_KNOTS('',3,(#163994,#163995,#163996,#163997,
#163998,#163999,#164000,#164001,#164002,#164003,#164004,#164005,#164006,
#164007,#164008,#164009,#164010,#164011,#164012,#164013,#164014,#164015,
#164016,#164017,#164018,#164019,#164020,#164021,#164022,#164023,#164024,
#164025,#164026,#164027,#164028,#164029,#164030,#164031,#164032,#164033,
#164034,#164035,#164036,#164037,#164038,#164039,#164040,#164041,#164042,
#164043,#164044,#164045,#164046,#164047,#164048,#164049,#164050,#164051,
#164052,#164053,#164054,#164055,#164056,#164057,#164058,#164059,#164060,
#164061,#164062,#164063,#164064,#164065,#164066,#164067,#164068,#164069,
#164070,#164071,#164072,#164073,#164074,#164075,#164076,#164077,#164078,
#164079,#164080,#164081,#164082,#164083,#164084,#164085,#164086,#164087,
#164088,#164089,#164090,#164091,#164092,#164093,#164094,#164095,#164096,
#164097,#164098,#164099,#164100,#164101,#164102,#164103,#164104,#164105,
#164106,#164107,#164108,#164109,#164110,#164111,#164112,#164113,#164114,
#164115,#164116,#164117,#164118,#164119,#164120,#164121,#164122,#164123,
#164124,#164125,#164126,#164127,#164128,#164129,#164130,#164131,#164132,
#164133,#164134,#164135,#164136,#164137,#164138,#164139,#164140,#164141,
#164142,#164143,#164144,#164145,#164146,#164147,#164148,#164149,#164150,
#164151,#164152,#164153,#164154,#164155,#164156,#164157,#164158,#164159,
#164160,#164161,#164162,#164163,#164164,#164165,#164166,#164167,#164168,
#164169,#164170,#164171,#164172,#164173,#164174,#164175,#164176,#164177,
#164178,#164179,#164180,#164181,#164182,#164183,#164184,#164185,#164186,
#164187,#164188,#164189,#164190,#164191,#164192,#164193,#164194,#164195,
#164196,#164197,#164198,#164199,#164200,#164201,#164202,#164203,#164204,
#164205),.UNSPECIFIED.,.F.,.F.,(4,2,2,2,2,2,2,2,2,2,2,2,2,2,2,2,2,2,2,2,
2,2,2,2,2,2,2,2,2,2,2,2,2,2,2,2,2,2,2,2,2,2,2,2,2,2,2,2,2,2,2,2,2,2,2,2,
2,2,2,2,2,2,2,2,2,2,2,2,2,2,2,2,2,2,2,2,2,2,2,2,2,2,2,2,2,2,2,2,2,2,2,2,
2,2,2,2,2,2,2,2,2,2,2,2,2,4),(-23.5087927899511,-23.4968313698322,-23.4733204154092,
-23.389522330444,-23.290833133669,-23.2198070544226,-23.1653958453539,-23.1337185956986,
-23.1043786318951,-23.0635177792145,-22.9134718397736,-22.8429454197137,
-22.7989334068048,-22.7789206549434,-22.7621106639869,-22.7366024110544,
-22.5970484570337,-22.5173636578392,-22.4597840963954,-22.4276466482817,
-22.3984581704448,-22.3588220335695,-22.2411753725644,-22.1484200315698,
-22.0970770954317,-22.0612857337457,-22.043403627955,-22.0278426792721,
-22.0043309391874,-21.9205308578202,-21.8218385050015,-21.7508098285477,
-21.6963967121042,-21.6647184193347,-21.6353775280291,-21.5945154493004,
-21.4444635489012,-21.3739355004649,-21.3299223152833,-21.3099089593149,
-21.2930984210289,-21.2675892800697,-21.1280304760964,-21.0483434323024,
-20.9907621643042,-20.958623710459,-20.9294342919689,-20.8897968349208,
-20.7721434073732,-20.6793555736253,-20.6280297185314,-20.5922461116202,
-20.5743650417727,-20.5588030561401,-20.5352869931688,-20.4515407559718,
-20.3528454009096,-20.2817886006594,-20.2273604978313,-20.195678845116,
-20.1663379205417,-20.1254810247372,-19.9753323695748,-19.9048518541056,
-19.8608559714563,-19.8408448522938,-19.8240330293425,-19.7985173807911,
-19.6589229238285,-19.5792579494841,-19.5216858060394,-19.4895481517101,
-19.4603572646099,-19.4207143584248,-19.302809919845,-19.2087262937014,
-19.1582846275073,-19.1229230165088,-19.1051181396125,-19.0897066218821,
-19.0661782991244,-18.9825364446692,-18.8838381644915,-18.8127353675039,
-18.7582831250707,-18.7265964880695,-18.6972561479971,-18.6564088951883,
-18.5061019142493,-18.4357020284634,-18.3917359069127,-18.3717289409319,
-18.3549153292737,-18.329389359514,-18.1897347780319,-18.1101103762315,
-18.0525556034341,-18.0204201202029,-17.9912273562865,-17.9515758407652,
-17.8332048197293,-17.7198606513816,-17.6801363305922,-17.650232961444,
-17.6334692206125,-17.6325413712744),.UNSPECIFIED.);
#30135=B_SPLINE_CURVE_WITH_KNOTS('',3,(#164206,#164207,#164208,#164209,
#164210,#164211,#164212,#164213,#164214,#164215,#164216,#164217,#164218,
#164219,#164220,#164221,#164222,#164223,#164224,#164225,#164226,#164227,
#164228,#164229,#164230,#164231,#164232,#164233,#164234,#164235,#164236,
#164237,#164238,#164239,#164240,#164241,#164242,#164243,#164244,#164245,
#164246,#164247,#164248,#164249,#164250,#164251,#164252,#164253,#164254,
#164255,#164256,#164257,#164258,#164259,#164260,#164261,#164262,#164263,
#164264,#164265,#164266,#164267,#164268,#164269,#164270,#164271,#164272,
#164273,#164274,#164275,#164276,#164277,#164278,#164279,#164280,#164281,
#164282,#164283,#164284,#164285,#164286,#164287,#164288,#164289,#164290,
#164291,#164292,#164293,#164294,#164295,#164296,#164297,#164298,#164299,
#164300,#164301,#164302,#164303,#164304,#164305,#164306,#164307,#164308,
#164309,#164310,#164311,#164312,#164313,#164314,#164315,#164316,#164317,
#164318,#164319,#164320,#164321,#164322,#164323,#164324,#164325,#164326,
#164327,#164328,#164329,#164330,#164331,#164332,#164333,#164334,#164335,
#164336,#164337,#164338,#164339,#164340,#164341,#164342,#164343,#164344,
#164345,#164346,#164347,#164348,#164349,#164350,#164351,#164352,#164353,
#164354,#164355,#164356,#164357,#164358,#164359,#164360,#164361,#164362,
#164363,#164364,#164365,#164366,#164367,#164368,#164369,#164370,#164371,
#164372,#164373,#164374,#164375,#164376,#164377,#164378,#164379,#164380,
#164381,#164382,#164383,#164384,#164385,#164386,#164387,#164388,#164389,
#164390,#164391,#164392,#164393,#164394,#164395,#164396,#164397,#164398,
#164399,#164400,#164401,#164402,#164403,#164404,#164405,#164406,#164407,
#164408,#164409,#164410,#164411,#164412,#164413,#164414,#164415,#164416,
#164417),.UNSPECIFIED.,.F.,.F.,(4,2,2,2,2,2,2,2,2,2,2,2,2,2,2,2,2,2,2,2,
2,2,2,2,2,2,2,2,2,2,2,2,2,2,2,2,2,2,2,2,2,2,2,2,2,2,2,2,2,2,2,2,2,2,2,2,
2,2,2,2,2,2,2,2,2,2,2,2,2,2,2,2,2,2,2,2,2,2,2,2,2,2,2,2,2,2,2,2,2,2,2,2,
2,2,2,2,2,2,2,2,2,2,2,2,2,4),(-12.3895147069527,-12.377807257671,-12.3632813542591,
-12.3267754286178,-12.1714619301749,-12.1004236322622,-12.0460030633795,
-12.014320365083,-11.9849753549371,-11.9441074748392,-11.7940357195205,
-11.7234971735021,-11.6794775922804,-11.6594613985178,-11.642648516205,
-11.6171358753871,-11.4775579155955,-11.397859412922,-11.3402699488588,
-11.3081269733203,-11.2789334750683,-11.2392905204773,-11.1216236031218,
-11.028852099042,-10.9775004647937,-10.9417030101661,-10.9238178400865,
-10.9082542111278,-10.8847384017566,-10.8009244242619,-10.702215098039,
-10.6311739600063,-10.5767513591747,-10.5450675955751,-10.5157216662698,
-10.4748526208287,-10.3247740369237,-10.2542343319478,-10.2102137547144,
-10.1901969838709,-10.1733835471008,-10.1478699644682,-10.0082868665789,
-9.92858634718545,-9.87099527794653,-9.83885131344926,-9.80965686943057,
-9.77001255569823,-9.65233662531578,-9.55951046683855,-9.50818996136906,
-9.4724069399824,-9.45452401270246,-9.4389589417329,-9.41543612792821,-9.33170680362448,
-9.23299455169726,-9.16191201462924,-9.10746762671221,-9.07577929839688,
-9.04643380002528,-9.0055732668675,-8.85535106321629,-8.7848842268555,-8.74089047733835,
-8.72087740837846,-8.70406230594376,-8.67853931489024,-8.53890406411337,
-8.45923850498894,-8.40166230375907,-8.36952009599412,-8.34032390293436,
-8.30067194889025,-8.18261088356668,-8.08785230533081,-8.03785700456833,
-8.00270826578259,-7.98494028438201,-7.96951250192704,-7.9458893753669,
-7.86262072124033,-7.76390596017912,-7.69268698263105,-7.63817216266634,
-7.60647064912219,-7.57712887290436,-7.53630054769812,-7.38561225972224,
-7.31539114302896,-7.27148935423217,-7.25149001879428,-7.23467061448617,
-7.2091182507377,-7.06928624042655,-6.98976200267619,-6.93224810822009,
-6.90011556261007,-6.87091528493107,-6.83123751778278,-6.71128806744215,
-6.59914285794704,-6.55961080606437,-6.52980993051937,-6.51306470671676,
-6.51219502816774),.UNSPECIFIED.);
#30136=B_SPLINE_CURVE_WITH_KNOTS('',3,(#164424,#164425,#164426,#164427,
#164428,#164429,#164430,#164431,#164432,#164433,#164434,#164435,#164436,
#164437,#164438,#164439,#164440,#164441,#164442,#164443,#164444,#164445,
#164446,#164447,#164448,#164449,#164450,#164451,#164452,#164453,#164454,
#164455,#164456,#164457,#164458,#164459,#164460,#164461,#164462,#164463,
#164464,#164465,#164466,#164467,#164468,#164469,#164470,#164471,#164472,
#164473,#164474,#164475,#164476,#164477,#164478,#164479,#164480,#164481,
#164482,#164483,#164484,#164485,#164486,#164487,#164488,#164489,#164490,
#164491,#164492,#164493,#164494,#164495,#164496,#164497,#164498,#164499,
#164500,#164501,#164502,#164503,#164504,#164505,#164506,#164507,#164508,
#164509,#164510,#164511,#164512,#164513,#164514,#164515,#164516,#164517,
#164518,#164519,#164520,#164521,#164522,#164523,#164524,#164525,#164526,
#164527,#164528,#164529,#164530,#164531,#164532,#164533,#164534,#164535,
#164536,#164537,#164538,#164539,#164540,#164541,#164542,#164543,#164544,
#164545,#164546,#164547,#164548,#164549,#164550,#164551,#164552,#164553,
#164554,#164555,#164556,#164557,#164558,#164559,#164560,#164561,#164562,
#164563,#164564,#164565,#164566,#164567,#164568,#164569,#164570,#164571,
#164572,#164573,#164574,#164575,#164576,#164577,#164578,#164579,#164580,
#164581,#164582,#164583,#164584,#164585,#164586,#164587,#164588,#164589,
#164590,#164591,#164592,#164593,#164594,#164595,#164596,#164597,#164598,
#164599,#164600,#164601,#164602,#164603,#164604,#164605,#164606,#164607,
#164608,#164609,#164610,#164611,#164612,#164613,#164614,#164615,#164616,
#164617,#164618,#164619,#164620,#164621,#164622,#164623,#164624,#164625,
#164626,#164627),.UNSPECIFIED.,.F.,.F.,(4,2,2,2,2,2,2,2,2,2,2,2,2,2,2,2,
2,2,2,2,2,2,2,2,2,2,2,2,2,2,2,2,2,2,2,2,2,2,2,2,2,2,2,2,2,2,2,2,2,2,2,2,
2,2,2,2,2,2,2,2,2,2,2,2,2,2,2,2,2,2,2,2,2,2,2,2,2,2,2,2,2,2,2,2,2,2,2,2,
2,2,2,2,2,2,2,2,2,2,2,2,2,4),(-29.154596735575,-29.0680469775082,-29.0366008769626,
-29.009649364794,-28.980358946728,-28.9398354719708,-28.7890301469152,-28.718512760047,
-28.6745063857758,-28.6544961985365,-28.6376883621472,-28.6121833791968,
-28.4726473149498,-28.392972725798,-28.3354005428435,-28.3032672134614,
-28.2740824766732,-28.2344514203136,-28.1168198660072,-28.0240766912348,
-27.9727401591336,-27.9369533008584,-27.9190734718067,-27.9035145225909,
-27.8800058295461,-27.7962157970364,-27.6975360912537,-27.6265168456998,
-27.572110870966,-27.5404366680126,-27.5110995257468,-27.4702426019138,
-27.3202111034496,-27.2496914600294,-27.2056836775571,-27.1856728499932,
-27.1688644757543,-27.143358676646,-27.0038181472543,-26.9241410085203,
-26.8665669832593,-26.8344326256126,-26.8052469549149,-26.7656146303642,
-26.647979311855,-26.555233169304,-26.5038949944387,-26.4681069909873,-26.4502265897825,
-26.4346671426812,-26.4111576973591,-26.3273649835731,-26.2286821200446,
-26.1576606018781,-26.1032528861554,-26.0715776696288,-26.0422395885759,
-26.0013813573234,-25.8513450578567,-25.7808231578136,-25.7368139670951,
-25.7168024991859,-25.69999358708,-25.6744869717877,-25.534941977107,-25.4552622887116,
-25.3976864210865,-25.3655510351428,-25.3363644305056,-25.2967308377232,
-25.1790917548905,-25.0863426444483,-25.0350028267789,-24.9992136781203,
-24.9813327047451,-24.9657727597423,-24.9422625621174,-24.8584671670318,
-24.7597811456606,-24.6887573547836,-24.6343478980047,-24.6026716678716,
-24.5733326480036,-24.5324731092984,-24.3824320085824,-24.3119078518984,
-24.26789725291,-24.2478851446385,-24.231075694648,-24.2055682631395,-24.0660188029948,
-23.9863365648802,-23.9287588548426,-23.8966224405704,-23.8674349019629,
-23.8278000409034,-23.7101571933654,-23.6174051123933,-23.566063653479,
-23.5302733603428,-23.5123918149171,-23.5087927899511),.UNSPECIFIED.);
#30137=B_SPLINE_CURVE_WITH_KNOTS('',3,(#164628,#164629,#164630,#164631,
#164632,#164633,#164634,#164635,#164636,#164637,#164638,#164639,#164640,
#164641,#164642,#164643,#164644,#164645,#164646,#164647,#164648,#164649,
#164650,#164651,#164652,#164653,#164654,#164655,#164656,#164657,#164658,
#164659,#164660,#164661,#164662,#164663,#164664,#164665,#164666,#164667,
#164668,#164669,#164670,#164671,#164672,#164673,#164674,#164675,#164676,
#164677,#164678,#164679,#164680,#164681,#164682,#164683,#164684,#164685,
#164686,#164687,#164688,#164689,#164690,#164691,#164692,#164693,#164694,
#164695,#164696,#164697,#164698,#164699,#164700,#164701,#164702,#164703,
#164704,#164705,#164706,#164707,#164708,#164709,#164710,#164711,#164712,
#164713,#164714,#164715,#164716,#164717,#164718,#164719,#164720,#164721,
#164722,#164723,#164724,#164725,#164726,#164727,#164728,#164729,#164730,
#164731,#164732,#164733,#164734,#164735,#164736,#164737,#164738,#164739,
#164740,#164741,#164742,#164743,#164744,#164745,#164746,#164747,#164748,
#164749,#164750,#164751,#164752,#164753,#164754,#164755,#164756,#164757,
#164758,#164759,#164760,#164761,#164762,#164763,#164764,#164765,#164766,
#164767,#164768,#164769,#164770,#164771,#164772,#164773,#164774,#164775,
#164776,#164777,#164778,#164779,#164780,#164781,#164782,#164783,#164784,
#164785,#164786,#164787,#164788,#164789,#164790,#164791,#164792,#164793,
#164794,#164795,#164796,#164797,#164798,#164799,#164800,#164801,#164802,
#164803,#164804,#164805,#164806,#164807,#164808,#164809,#164810,#164811,
#164812,#164813,#164814,#164815,#164816,#164817,#164818,#164819,#164820,
#164821,#164822,#164823,#164824,#164825,#164826,#164827,#164828,#164829),
 .UNSPECIFIED.,.F.,.F.,(4,2,2,2,2,2,2,2,2,2,2,2,2,2,2,2,2,2,2,2,2,2,2,2,
2,2,2,2,2,2,2,2,2,2,2,2,2,2,2,2,2,2,2,2,2,2,2,2,2,2,2,2,2,2,2,2,2,2,2,2,
2,2,2,2,2,2,2,2,2,2,2,2,2,2,2,2,2,2,2,2,2,2,2,2,2,2,2,2,2,2,2,2,2,2,2,2,
2,2,2,2,4),(-6.51219502816774,-6.49689472217411,-6.46997129052892,-6.33929047170556,
-6.1947859721142,-6.1544204919948,-6.12512902835179,-6.09328081973178,-6.0374576478002,
-5.96164855254946,-5.82372445141555,-5.79375782895583,-5.77621192813791,
-5.75779046594482,-5.72318471319209,-5.67467744732633,-5.49150139516094,
-5.44913881236605,-5.41986448638267,-5.38874266249544,-5.33748016546924,
-5.27244324153535,-5.16593489972955,-5.07913909304673,-5.05515738971787,
-5.0396742219655,-5.02205748198278,-4.98772940484716,-4.93942033450216,
-4.75043426596149,-4.6977392235594,-4.66636225158126,-4.63688499827377,
-4.59510699534641,-4.56898087592549,-4.49447943642386,-4.34936201571812,
-4.32198775929466,-4.30506608009003,-4.28593306721165,-4.2473386632098,
-4.13084640770648,-4.01243634219351,-3.97453782714609,-3.94547904169831,
-3.91279926357094,-3.85263912610603,-3.76978323189877,-3.63075714172454,
-3.5948194464321,-3.57690857557399,-3.56135272833126,-3.53789146688165,
-3.45009573499749,-3.26259524537362,-3.21925017479097,-3.18980575538939,
-3.15898330002587,-3.10910265272203,-3.04533935388429,-2.94551417146924,
-2.87306010393177,-2.84904131658227,-2.83239378132126,-2.81150257496362,
-2.76140175815404,-2.67298551663729,-2.55248337600327,-2.51022340991007,
-2.48096579391245,-2.44981682268409,-2.39839539525427,-2.30730525960288,
-2.14514366857188,-2.11871346457313,-2.10421914390871,-2.08789929894286,
-2.06021402931002,-1.96797504792757,-1.78729165291815,-1.74656534219371,
-1.71722549523362,-1.68551857864315,-1.63051638189085,-1.55645807035467,
-1.41006063025761,-1.38293344364847,-1.36605133247423,-1.34682686522701,
-1.30769669162197,-1.1903996757451,-1.07369608520175,-1.03576984837626,
-1.00670841764685,-0.974044489441254,-0.913975528066767,-0.8313170466221,
-0.693102441749089,-0.656423357532267,-0.638380021990908,-0.634450996246336),
 .UNSPECIFIED.);
#30138=B_SPLINE_CURVE_WITH_KNOTS('',3,(#164835,#164836,#164837,#164838,
#164839,#164840,#164841,#164842,#164843,#164844,#164845,#164846,#164847,
#164848,#164849,#164850,#164851,#164852,#164853,#164854,#164855,#164856,
#164857,#164858,#164859,#164860,#164861,#164862,#164863,#164864,#164865,
#164866,#164867,#164868,#164869,#164870,#164871,#164872,#164873,#164874,
#164875,#164876,#164877,#164878,#164879,#164880,#164881,#164882,#164883,
#164884,#164885,#164886,#164887,#164888,#164889,#164890,#164891,#164892,
#164893,#164894,#164895,#164896,#164897,#164898,#164899,#164900,#164901,
#164902,#164903,#164904,#164905,#164906,#164907,#164908,#164909,#164910,
#164911,#164912,#164913,#164914,#164915,#164916,#164917,#164918,#164919,
#164920,#164921,#164922,#164923,#164924,#164925,#164926,#164927,#164928,
#164929,#164930,#164931,#164932,#164933,#164934,#164935,#164936,#164937,
#164938,#164939,#164940,#164941,#164942,#164943,#164944,#164945,#164946,
#164947,#164948,#164949,#164950,#164951,#164952,#164953,#164954,#164955,
#164956,#164957,#164958,#164959,#164960,#164961,#164962,#164963,#164964,
#164965,#164966,#164967,#164968,#164969,#164970,#164971,#164972),
 .UNSPECIFIED.,.F.,.F.,(4,2,2,2,2,2,2,2,2,2,2,2,2,2,2,2,2,2,2,2,2,2,2,2,
2,2,2,2,2,2,2,2,2,2,2,2,2,2,2,2,2,2,2,2,2,2,2,2,2,2,2,2,2,2,2,2,2,2,2,2,
2,2,2,2,2,2,2,2,4),(-3.2456129003934,-3.24151973927817,-3.23300392887545,
-3.21464854915612,-3.13705852807635,-2.9528080579948,-2.89330519802188,
-2.87273145681729,-2.85933340186152,-2.84651462975601,-2.82887122294633,
-2.78603698053238,-2.72313221862484,-2.63586417862452,-2.53328362850053,
-2.51288600487319,-2.50369709015821,-2.49660483534415,-2.48825976819539,
-2.47268283796893,-2.35265936259145,-2.19298651208667,-2.16604760658548,
-2.1498637084089,-2.13722877649194,-2.12336785393765,-2.10063386868242,
-2.01050169504874,-1.90468427825519,-1.78700536024996,-1.7664172081085,
-1.75838355622291,-1.75176386535067,-1.74460349259306,-1.73282431405224,
-1.68904423506647,-1.60068618089287,-1.41986982946812,-1.38883000707498,
-1.37303502142016,-1.36047465266443,-1.34624116192914,-1.32175821863759,
-1.18262002171282,-1.03751793083754,-1.0189995758897,-1.01006323001346,
-1.00299723872,-0.994331961508112,-0.97719335369875,-0.954503392578678,
-0.897355449029842,-0.698170085462727,-0.672255062571138,-0.656192979047803,
-0.643606184760003,-0.629535838183939,-0.605829791594677,-0.499755432290025,
-0.405721615865298,-0.294140531709845,-0.273972105360895,-0.265761711513818,
-0.259098271344394,-0.252019846976943,-0.240611437057429,-0.200849659954101,
-0.125463182742716,-0.000228192652907022),.UNSPECIFIED.);
#30139=B_SPLINE_CURVE_WITH_KNOTS('',3,(#164975,#164976,#164977,#164978,
#164979,#164980,#164981,#164982,#164983,#164984,#164985,#164986,#164987,
#164988,#164989,#164990,#164991,#164992,#164993,#164994,#164995,#164996,
#164997,#164998,#164999,#165000,#165001,#165002,#165003,#165004,#165005,
#165006,#165007,#165008,#165009,#165010,#165011,#165012,#165013,#165014,
#165015,#165016,#165017,#165018,#165019,#165020,#165021,#165022,#165023,
#165024,#165025,#165026,#165027,#165028,#165029,#165030,#165031,#165032,
#165033,#165034,#165035,#165036,#165037,#165038,#165039,#165040,#165041,
#165042,#165043,#165044,#165045,#165046,#165047,#165048,#165049,#165050,
#165051,#165052,#165053,#165054,#165055,#165056,#165057,#165058,#165059,
#165060,#165061,#165062,#165063,#165064,#165065,#165066,#165067,#165068,
#165069,#165070,#165071,#165072,#165073,#165074,#165075,#165076,#165077,
#165078,#165079,#165080,#165081,#165082,#165083,#165084,#165085,#165086,
#165087,#165088,#165089,#165090,#165091,#165092,#165093,#165094,#165095,
#165096,#165097,#165098,#165099,#165100,#165101,#165102),.UNSPECIFIED.,
 .F.,.F.,(4,2,2,2,2,2,2,2,2,2,2,2,2,2,2,2,2,2,2,2,2,2,2,2,2,2,2,2,2,2,2,
2,2,2,2,2,2,2,2,2,2,2,2,2,2,2,2,2,2,2,2,2,2,2,2,2,2,2,2,2,2,2,2,4),(-20.6404265031114,
-20.5538188837533,-20.5366027537719,-20.5238741986076,-20.5110137403867,
-20.4992592678507,-20.4833663937635,-20.443525073977,-20.3505999831602,
-20.2477399606774,-20.2003627857329,-20.180268831843,-20.1646632979875,
-20.1563126916547,-20.1492219223327,-20.1400427117604,-20.1196965355734,
-20.0187640405624,-19.9332601172847,-19.8682796548066,-19.8244542175184,
-19.8066584598254,-19.7938137729206,-19.780463457377,-19.7601125918741,
-19.7024760434826,-19.5158994343518,-19.4383141633649,-19.4199601864392,
-19.4114450723809,-19.4049018792084,-19.3972056083733,-19.3833544735927,
-19.313452632251,-19.1726005317205,-19.0709030414189,-19.0417266274786,
-19.0265093092129,-19.0152021534447,-19.0009872434407,-18.9765899308292,
-18.8482124631035,-18.7550463745566,-18.7076579169902,-18.6782100025422,
-18.6674952982743,-18.6601941239403,-18.6534402627088,-18.6417779835096,
-18.6077638334634,-18.5659273946448,-18.4453233307968,-18.3774261007886,
-18.3322356165173,-18.3142332752973,-18.301351351476,-18.2896227119443,
-18.2708315619069,-18.2241038488764,-18.023334188905,-17.945581828206,-17.9272086899218,
-17.9186899223837,-17.9145909763123),.UNSPECIFIED.);
#30140=B_SPLINE_CURVE_WITH_KNOTS('',3,(#165107,#165108,#165109,#165110,
#165111,#165112,#165113,#165114,#165115,#165116,#165117,#165118,#165119,
#165120,#165121,#165122,#165123,#165124,#165125,#165126,#165127,#165128,
#165129,#165130,#165131,#165132,#165133,#165134,#165135,#165136,#165137,
#165138,#165139,#165140,#165141,#165142,#165143,#165144,#165145,#165146,
#165147,#165148,#165149,#165150,#165151,#165152,#165153,#165154,#165155,
#165156,#165157,#165158,#165159,#165160,#165161,#165162,#165163,#165164,
#165165,#165166,#165167,#165168,#165169,#165170,#165171,#165172,#165173,
#165174,#165175,#165176,#165177,#165178,#165179,#165180,#165181,#165182,
#165183,#165184,#165185,#165186,#165187,#165188,#165189,#165190,#165191,
#165192,#165193,#165194,#165195,#165196,#165197,#165198,#165199,#165200,
#165201,#165202,#165203,#165204,#165205,#165206,#165207,#165208,#165209,
#165210,#165211,#165212,#165213,#165214,#165215,#165216,#165217,#165218,
#165219,#165220,#165221,#165222,#165223,#165224,#165225,#165226,#165227,
#165228,#165229,#165230,#165231,#165232,#165233,#165234,#165235,#165236,
#165237,#165238,#165239,#165240,#165241,#165242,#165243,#165244,#165245,
#165246,#165247,#165248,#165249,#165250,#165251,#165252,#165253,#165254,
#165255,#165256,#165257,#165258,#165259,#165260,#165261,#165262,#165263,
#165264,#165265,#165266,#165267,#165268,#165269,#165270,#165271,#165272,
#165273,#165274,#165275,#165276,#165277,#165278,#165279,#165280,#165281,
#165282,#165283,#165284,#165285,#165286,#165287,#165288,#165289,#165290,
#165291,#165292,#165293,#165294,#165295,#165296,#165297,#165298,#165299,
#165300,#165301,#165302,#165303,#165304,#165305,#165306,#165307,#165308,
#165309,#165310,#165311,#165312,#165313,#165314,#165315,#165316,#165317,
#165318,#165319,#165320,#165321,#165322,#165323,#165324,#165325,#165326,
#165327,#165328,#165329,#165330,#165331,#165332,#165333,#165334,#165335,
#165336,#165337,#165338,#165339,#165340,#165341,#165342,#165343,#165344,
#165345,#165346,#165347,#165348,#165349,#165350,#165351,#165352,#165353,
#165354,#165355,#165356,#165357,#165358,#165359,#165360,#165361,#165362,
#165363,#165364,#165365,#165366,#165367,#165368),.UNSPECIFIED.,.F.,.F.,
(4,2,2,2,2,2,2,2,2,2,2,2,2,2,2,2,2,2,2,2,2,2,2,2,2,2,2,2,2,2,2,2,2,2,2,
2,2,2,2,2,2,2,2,2,2,2,2,2,2,2,2,2,2,2,2,2,2,2,2,2,2,2,2,2,2,2,2,2,2,2,2,
2,2,2,2,2,2,2,2,2,2,2,2,2,2,2,2,2,2,2,2,2,2,2,2,2,2,2,2,2,2,2,2,2,2,2,2,
2,2,2,2,2,2,2,2,2,2,2,2,2,2,2,2,2,2,2,2,2,2,2,4),(-9.21748158827845,-9.21382472857645,
-9.20555010398746,-9.19226665746033,-9.08755739849233,-8.91019214907064,
-8.86181086810311,-8.84276324903766,-8.83098746131698,-8.81814313254699,
-8.80035991220493,-8.75663018859442,-8.69185628427859,-8.60704520878716,
-8.50506244227701,-8.48467657989922,-8.47548919028004,-8.46839643428287,
-8.46004874080444,-8.44446181290621,-8.32379220608945,-8.16484608717407,
-8.1378515091685,-8.12165092296186,-8.10901261910952,-8.09515781045967,
-8.0724564945001,-7.98281494607982,-7.87666389084958,-7.75872555223543,
-7.73813633891077,-7.73010201566733,-7.72348167155071,-7.71632046338717,
-7.70453966708904,-7.66075062345517,-7.5723683063852,-7.39145494653566,
-7.36047267593528,-7.34468856583957,-7.33212801135452,-7.31788486353923,
-7.29336115763615,-7.15172956036571,-7.00959248101371,-6.99079374299124,
-6.9818031416346,-6.97473458651297,-6.96611549471299,-6.94920905223148,
-6.92691915070103,-6.87134369617109,-6.68734580804887,-6.64781616132574,
-6.63203215980734,-6.62030286023555,-6.60741590293669,-6.58939729735798,
-6.54429661423769,-6.47795241799782,-6.3801374681796,-6.26582878573395,
-6.24560893993672,-6.23738911415706,-6.23072274995958,-6.22364722066697,
-6.21225423137606,-6.17265924039142,-6.09778395559222,-5.91021013481413,
-5.87184439771556,-5.85618008270338,-5.84447963852268,-5.83156765660398,
-5.81340717427366,-5.76715521131481,-5.6969415960481,-5.56013740382126,
-5.50779235098627,-5.49427484489502,-5.48637114686605,-5.47916739440721,
-5.46899522993174,-5.44329686608043,-5.40422697089216,-5.30154519405414,
-5.16939500832562,-5.14495830728065,-5.130733968207,-5.11942656235678,-5.10421827374453,
-5.07509171248983,-4.97376105119414,-4.83335887206876,-4.76256814021437,
-4.74867875224038,-4.74097340161693,-4.73443047191177,-4.72592605206858,
-4.70763247322185,-4.63058636455537,-4.43098599274847,-4.3827660741241,
-4.36374392954782,-4.35197342868982,-4.33912660745904,-4.32132461119646,
-4.27746619415442,-4.21241844540731,-4.12696444880667,-4.02604803005594,
-4.00570078156937,-3.99652078718055,-3.98942928108482,-3.98107764425874,
-3.96546978382914,-3.94537271838847,-3.89798711802878,-3.80481214765171,
-3.6764259104078,-3.65202668378943,-3.63781060333696,-3.62650248684246,
-3.61128383069372,-3.58210472001241,-3.4803963523489,-3.3395213464396,-3.26961286108437,
-3.25576043951311,-3.24806348956315,-3.2456129003934),.UNSPECIFIED.);
#30141=B_SPLINE_CURVE_WITH_KNOTS('',3,(#165369,#165370,#165371,#165372,
#165373,#165374,#165375,#165376,#165377,#165378,#165379,#165380,#165381,
#165382,#165383,#165384,#165385,#165386,#165387,#165388,#165389,#165390,
#165391,#165392,#165393,#165394,#165395,#165396,#165397,#165398,#165399,
#165400,#165401,#165402,#165403,#165404,#165405,#165406,#165407,#165408,
#165409,#165410,#165411,#165412,#165413,#165414,#165415,#165416,#165417,
#165418,#165419,#165420,#165421,#165422,#165423,#165424,#165425,#165426,
#165427,#165428,#165429,#165430,#165431,#165432,#165433,#165434,#165435,
#165436,#165437,#165438,#165439,#165440,#165441,#165442,#165443,#165444,
#165445,#165446,#165447,#165448,#165449,#165450,#165451,#165452,#165453,
#165454,#165455,#165456,#165457,#165458,#165459,#165460,#165461,#165462,
#165463,#165464,#165465,#165466,#165467,#165468,#165469,#165470,#165471,
#165472,#165473,#165474,#165475,#165476,#165477,#165478,#165479,#165480,
#165481,#165482,#165483,#165484,#165485,#165486,#165487,#165488,#165489,
#165490,#165491,#165492,#165493,#165494,#165495,#165496,#165497,#165498,
#165499,#165500,#165501,#165502,#165503,#165504,#165505,#165506,#165507,
#165508,#165509,#165510,#165511,#165512,#165513,#165514,#165515,#165516,
#165517,#165518,#165519,#165520,#165521,#165522,#165523,#165524,#165525,
#165526,#165527,#165528,#165529,#165530,#165531,#165532,#165533,#165534,
#165535,#165536,#165537,#165538,#165539,#165540,#165541,#165542,#165543,
#165544,#165545,#165546,#165547,#165548,#165549,#165550,#165551,#165552,
#165553,#165554,#165555,#165556,#165557,#165558,#165559,#165560,#165561,
#165562,#165563,#165564,#165565,#165566,#165567,#165568,#165569,#165570,
#165571,#165572,#165573,#165574,#165575,#165576,#165577,#165578,#165579,
#165580,#165581,#165582,#165583,#165584,#165585,#165586,#165587,#165588,
#165589,#165590,#165591,#165592,#165593,#165594,#165595,#165596,#165597,
#165598,#165599,#165600,#165601,#165602,#165603,#165604,#165605,#165606,
#165607,#165608,#165609,#165610,#165611,#165612,#165613,#165614,#165615,
#165616,#165617,#165618,#165619,#165620,#165621,#165622,#165623,#165624,
#165625,#165626,#165627,#165628,#165629,#165630,#165631,#165632),
 .UNSPECIFIED.,.F.,.F.,(4,2,2,2,2,2,2,2,2,2,2,2,2,2,2,2,2,2,2,2,2,2,2,2,
2,2,2,2,2,2,2,2,2,2,2,2,2,2,2,2,2,2,2,2,2,2,2,2,2,2,2,2,2,2,2,2,2,2,2,2,
2,2,2,2,2,2,2,2,2,2,2,2,2,2,2,2,2,2,2,2,2,2,2,2,2,2,2,2,2,2,2,2,2,2,2,2,
2,2,2,2,2,2,2,2,2,2,2,2,2,2,2,2,2,2,2,2,2,2,2,2,2,2,2,2,2,2,2,2,2,2,2,4),
(-17.9145909763123,-17.9121463149229,-17.9044523773332,-17.8906120035617,
-17.8209721505478,-17.6800253356371,-17.5781715345178,-17.54897299257,-17.5337510479476,
-17.5224432866508,-17.5082313166204,-17.4838484557573,-17.3562463996887,
-17.2096147603588,-17.1840722578969,-17.1739245593704,-17.1667253213257,
-17.1588122855645,-17.1452501576726,-17.0922772504089,-16.9568654998564,
-16.8862532631213,-16.8398218323326,-16.8216360627537,-16.8087201634212,
-16.7970255318323,-16.7813829594699,-16.7431418448027,-16.5554414631575,
-16.4805350359567,-16.44093113087,-16.4295378614113,-16.4224626400556,-16.4157969688591,
-16.407578422791,-16.3873637604223,-16.2732260223652,-16.1759908051098,
-16.1092168867775,-16.063908043945,-16.045858903648,-16.032967121291,-16.0196881544029,
-15.9996738026445,-15.9441875189247,-15.7934054825846,-15.7083435345649,
-15.6887186401988,-15.6795730555433,-15.6731710144705,-15.6649712812535,
-15.6504804351063,-15.5781271396811,-15.4490463168124,-15.3875712717742,
-15.3454305202164,-15.327896376873,-15.315096658422,-15.3016643759991,-15.2809279154852,
-15.2199961674478,-15.0375383776727,-14.9599290406113,-14.9415717234541,
-14.9330556653237,-14.9265120238059,-14.9188155523938,-14.9049648168994,
-14.8350890776082,-14.6942153229771,-14.5924951584541,-14.563314626739,
-14.5480958880551,-14.5367879748653,-14.5225725022773,-14.4981752146796,
-14.3698760047884,-14.2769009697618,-14.2293264238139,-14.2091768931081,
-14.1935376486409,-14.1851795551169,-14.178089090624,-14.1689186335417,
-14.1486238867513,-14.0491287473219,-13.96599195866,-13.8986326047346,-13.8536902543354,
-13.8357241923833,-13.8228481238843,-13.8111112307353,-13.7922769922941,
-13.7452785462086,-13.5244599296396,-13.4587110752116,-13.445452469443,
-13.43796725459,-13.431386335647,-13.4226838224456,-13.4027832550075,-13.2605232472613,
-13.1476410845656,-13.1048876281172,-13.072374830324,-13.0565009335129,
-13.0439321930748,-13.0297469209276,-13.0054930521031,-12.8877696989127,
-12.7638180454279,-12.7286386699555,-12.7048203340245,-12.694945031054,
-12.6877878228131,-12.679748777692,-12.6656090121849,-12.6035138427132,
-12.4753422918281,-12.4065313559282,-12.3609185071692,-12.3428520073658,
-12.3299572223299,-12.3182390812238,-12.3025011560222,-12.2633670807237,
-12.0765034759226,-12.001805440768,-11.9622690274271,-11.9508816527243,
-11.943807305019,-11.9431123563756),.UNSPECIFIED.);
#30142=B_SPLINE_CURVE_WITH_KNOTS('',3,(#165637,#165638,#165639,#165640,
#165641,#165642,#165643,#165644,#165645,#165646,#165647,#165648,#165649,
#165650,#165651,#165652,#165653,#165654,#165655,#165656,#165657,#165658,
#165659,#165660,#165661,#165662,#165663,#165664,#165665,#165666,#165667,
#165668,#165669,#165670,#165671,#165672,#165673,#165674,#165675,#165676,
#165677,#165678,#165679,#165680,#165681,#165682,#165683,#165684,#165685,
#165686,#165687,#165688,#165689,#165690,#165691,#165692,#165693,#165694,
#165695,#165696,#165697,#165698,#165699,#165700,#165701,#165702,#165703,
#165704,#165705,#165706,#165707,#165708,#165709,#165710,#165711,#165712,
#165713,#165714,#165715,#165716,#165717,#165718,#165719,#165720,#165721,
#165722,#165723,#165724,#165725,#165726,#165727,#165728,#165729,#165730,
#165731,#165732,#165733,#165734,#165735,#165736,#165737,#165738,#165739,
#165740,#165741,#165742,#165743,#165744,#165745,#165746,#165747,#165748,
#165749,#165750,#165751,#165752,#165753,#165754,#165755,#165756,#165757,
#165758,#165759,#165760,#165761,#165762,#165763,#165764,#165765,#165766,
#165767,#165768,#165769,#165770,#165771,#165772,#165773,#165774,#165775,
#165776,#165777,#165778,#165779,#165780,#165781,#165782,#165783,#165784,
#165785,#165786,#165787,#165788,#165789,#165790,#165791,#165792,#165793,
#165794,#165795,#165796,#165797,#165798,#165799,#165800,#165801,#165802,
#165803,#165804,#165805,#165806,#165807,#165808,#165809,#165810,#165811,
#165812,#165813,#165814,#165815,#165816,#165817,#165818,#165819,#165820,
#165821,#165822,#165823,#165824,#165825,#165826,#165827,#165828,#165829,
#165830,#165831,#165832,#165833,#165834,#165835,#165836,#165837,#165838,
#165839,#165840,#165841,#165842,#165843,#165844,#165845,#165846,#165847,
#165848,#165849,#165850,#165851,#165852,#165853,#165854,#165855,#165856,
#165857,#165858,#165859,#165860,#165861,#165862,#165863,#165864,#165865,
#165866,#165867,#165868,#165869,#165870,#165871,#165872,#165873,#165874,
#165875,#165876,#165877,#165878,#165879,#165880,#165881,#165882,#165883,
#165884,#165885,#165886,#165887,#165888,#165889,#165890,#165891,#165892,
#165893,#165894),.UNSPECIFIED.,.F.,.F.,(4,2,2,2,2,2,2,2,2,2,2,2,2,2,2,2,
2,2,2,2,2,2,2,2,2,2,2,2,2,2,2,2,2,2,2,2,2,2,2,2,2,2,2,2,2,2,2,2,2,2,2,2,
2,2,2,2,2,2,2,2,2,2,2,2,2,2,2,2,2,2,2,2,2,2,2,2,2,2,2,2,2,2,2,2,2,2,2,2,
2,2,2,2,2,2,2,2,2,2,2,2,2,2,2,2,2,2,2,2,2,2,2,2,2,2,2,2,2,2,2,2,2,2,2,2,
2,2,2,2,4),(-15.1894918505391,-15.1870416113486,-15.1793449807329,-15.1654935784906,
-15.0956024288551,-14.9547347015735,-14.8530224898747,-14.8238430395983,
-14.8086244993549,-14.7973165838072,-14.7831009124023,-14.7587027856351,
-14.630360052036,-14.5372855031732,-14.4898030161241,-14.4696791059428,
-14.454055252677,-14.4457003681928,-14.4386094579693,-14.4294344476659,
-14.4091143926754,-14.3088148987986,-14.2245001378627,-14.1583731650709,
-14.1140060255117,-14.0961267125243,-14.0832662687304,-14.0715119973594,
-14.055623424675,-14.0159071042666,-13.8297933552427,-13.7552867640185,
-13.7158143430029,-13.7044335377081,-13.697360822426,-13.6906930729186,
-13.6824673822671,-13.6622128678422,-13.5463875921862,-13.4437057197943,
-13.3812049502699,-13.3380028272016,-13.3202768897009,-13.3074427391972,
-13.2956541141949,-13.279625563326,-13.2389695955077,-13.0360789886683,
-12.9938057328544,-12.9666215028766,-12.9562264642999,-12.9489840600123,
-12.9411684396504,-12.9280538875842,-12.8802722446436,-12.7580389718178,
-12.6446841141885,-12.6143616073319,-12.5989223745428,-12.5863880816962,
-12.5719003467737,-12.5469281275898,-12.4053145989166,-12.3029797615794,
-12.2271850700113,-12.2134714137552,-12.2058879386375,-12.1993269724132,
-12.1907856736944,-12.1717946060692,-12.0175252796335,-11.9120985255636,
-11.850578002158,-11.8304076522327,-11.817093934446,-11.8043690444182,-11.7865383770859,
-11.7457246786345,-11.5444433204555,-11.5013100213407,-11.4737357750924,
-11.4632838017366,-11.4560310320658,-11.4482361697524,-11.4352167257948,
-11.3885284613779,-11.2436700442378,-11.1743561017675,-11.1285126424949,
-11.1104117471717,-11.0975103862839,-11.0857983146814,-11.0700866097557,
-11.0314408922365,-10.8441545081836,-10.7693489375529,-10.7297765622723,
-10.7183854673745,-10.7113101760597,-10.704643235399,-10.6964218823539,
-10.6761942862667,-10.5615499096762,-10.4627030421729,-10.3637923074457,
-10.3404874588252,-10.3265022755237,-10.313895769996,-10.2976747381143,
-10.2712173056198,-10.1051474455863,-9.99192088572466,-9.97554911063105,
-9.96703865407043,-9.95996315371423,-9.95084044521359,-9.93134226763777,
-9.79865177725536,-9.64905950282259,-9.6243062037698,-9.61001368715274,
-9.59745903772131,-9.58174779079974,-9.55008366237157,-9.3726918540088,
-9.24337589625386,-9.22823720114878,-9.22035297280733,-9.21748158827845),
 .UNSPECIFIED.);
#30143=B_SPLINE_CURVE_WITH_KNOTS('',3,(#165895,#165896,#165897,#165898,
#165899,#165900,#165901,#165902,#165903,#165904,#165905,#165906,#165907,
#165908,#165909,#165910,#165911,#165912,#165913,#165914,#165915,#165916,
#165917,#165918,#165919,#165920,#165921,#165922,#165923,#165924,#165925,
#165926,#165927,#165928,#165929,#165930,#165931,#165932,#165933,#165934,
#165935,#165936,#165937,#165938,#165939,#165940,#165941,#165942,#165943,
#165944,#165945,#165946,#165947,#165948,#165949,#165950,#165951,#165952,
#165953,#165954,#165955,#165956,#165957,#165958,#165959,#165960,#165961,
#165962,#165963,#165964,#165965,#165966,#165967,#165968,#165969,#165970,
#165971,#165972,#165973,#165974,#165975,#165976,#165977,#165978,#165979,
#165980,#165981,#165982,#165983,#165984,#165985,#165986,#165987,#165988,
#165989,#165990,#165991,#165992,#165993,#165994,#165995,#165996,#165997,
#165998,#165999,#166000,#166001,#166002,#166003,#166004,#166005,#166006,
#166007,#166008,#166009,#166010,#166011,#166012,#166013,#166014,#166015,
#166016,#166017,#166018,#166019,#166020,#166021,#166022,#166023,#166024,
#166025,#166026,#166027,#166028,#166029,#166030,#166031,#166032,#166033,
#166034,#166035,#166036,#166037,#166038,#166039,#166040,#166041,#166042,
#166043,#166044,#166045,#166046,#166047,#166048,#166049,#166050,#166051,
#166052,#166053,#166054,#166055,#166056,#166057,#166058,#166059,#166060,
#166061,#166062,#166063,#166064,#166065,#166066,#166067,#166068,#166069,
#166070,#166071,#166072,#166073,#166074,#166075,#166076,#166077,#166078,
#166079,#166080,#166081,#166082,#166083,#166084,#166085,#166086,#166087,
#166088,#166089,#166090,#166091,#166092,#166093,#166094,#166095,#166096,
#166097,#166098,#166099,#166100,#166101,#166102,#166103,#166104,#166105,
#166106,#166107,#166108,#166109,#166110,#166111,#166112,#166113,#166114,
#166115,#166116,#166117,#166118,#166119,#166120,#166121,#166122,#166123,
#166124,#166125,#166126,#166127,#166128,#166129,#166130,#166131,#166132,
#166133,#166134,#166135,#166136,#166137,#166138,#166139,#166140,#166141,
#166142,#166143,#166144,#166145,#166146),.UNSPECIFIED.,.F.,.F.,(4,2,2,2,
2,2,2,2,2,2,2,2,2,2,2,2,2,2,2,2,2,2,2,2,2,2,2,2,2,2,2,2,2,2,2,2,2,2,2,2,
2,2,2,2,2,2,2,2,2,2,2,2,2,2,2,2,2,2,2,2,2,2,2,2,2,2,2,2,2,2,2,2,2,2,2,2,
2,2,2,2,2,2,2,2,2,2,2,2,2,2,2,2,2,2,2,2,2,2,2,2,2,2,2,2,2,2,2,2,2,2,2,2,
2,2,2,2,2,2,2,2,2,2,2,2,2,4),(-11.9431123563756,-11.9371400945385,-11.9289172128653,
-11.9086800441113,-11.7935921533514,-11.6937260935414,-11.5961479228807,
-11.5729244680541,-11.5589570921374,-11.5463470432184,-11.5300939069081,
-11.5035247186011,-11.3389085811387,-11.2244999409633,-11.2080933282744,
-11.1995758733406,-11.1925011265811,-11.1833878091642,-11.163939126086,
-11.0289354641812,-10.8816233132815,-10.8568526541824,-10.8425566844538,
-10.8300028599394,-10.8142977371823,-10.7826638439394,-10.6049158771398,
-10.4759113732513,-10.4607769398394,-10.4528937237041,-10.4463656172844,
-10.4380902808621,-10.4248040481589,-10.3201645482951,-10.1429649225121,
-10.0944200747842,-10.0753480613444,-10.0635681277133,-10.0507278873983,
-10.0329662673887,-9.98937506419385,-9.92489190637708,-9.83947252087029,
-9.73761962873634,-9.71723787208984,-9.70805136989529,-9.70095887054295,
-9.69261095916566,-9.67702232298835,-9.55619263636395,-9.39744205095968,
-9.37043487760053,-9.3542309551249,-9.34159248032378,-9.32773995372433,
-9.30504806897216,-9.21553396853199,-9.10930686262019,-8.99130820639629,
-8.97071987207343,-8.9626858184261,-8.95606566791012,-8.94890463241116,
-8.93712405068992,-8.89333496225985,-8.8049507937886,-8.62404902692935,
-8.59306706635493,-8.57728327829012,-8.5647230588297,-8.55048037517143,
-8.52595768399791,-8.38435368020825,-8.24219256233126,-8.22339668294539,
-8.21440677514545,-8.20733843167372,-8.19871918972571,-8.18181129598609,
-8.15951872072812,-8.10393200279178,-7.91985797885726,-7.88039864853292,
-7.86462621735444,-7.85289991712386,-7.84001077378147,-7.82197876899257,
-7.77678742211517,-7.71025611290615,-7.61268765976083,-7.49845077059258,
-7.47823291956886,-7.47001356919396,-7.46334745266185,-7.45627201130869,
-7.4448788503633,-7.40527997835284,-7.3303917020678,-7.14276316507474,-7.10445327262611,
-7.08879861871029,-7.07710069280272,-7.06418683841725,-7.0460148300962,
-6.99968191063227,-6.92928866499938,-6.79311596066494,-6.74047763658306,
-6.72693901068511,-6.7190308384122,-6.71182913972786,-6.70166840345522,
-6.6760433499676,-6.52931785629973,-6.4019090495025,-6.37752900447575,-6.3633171389559,
-6.35200863497734,-6.33678461469793,-6.30757837164564,-6.20567478274499,
-6.06469422378829,-5.99511169331124,-5.9812730275737,-5.97357921617743,
-5.97113581786257),.UNSPECIFIED.);
#30144=B_SPLINE_CURVE_WITH_KNOTS('',3,(#166152,#166153,#166154,#166155,
#166156,#166157,#166158,#166159,#166160,#166161,#166162,#166163,#166164,
#166165,#166166,#166167,#166168,#166169,#166170,#166171,#166172,#166173,
#166174,#166175,#166176,#166177,#166178,#166179,#166180,#166181,#166182,
#166183,#166184,#166185,#166186,#166187,#166188,#166189,#166190,#166191,
#166192,#166193,#166194,#166195,#166196,#166197,#166198,#166199,#166200,
#166201,#166202,#166203,#166204,#166205,#166206,#166207,#166208,#166209,
#166210,#166211,#166212,#166213,#166214,#166215,#166216,#166217,#166218,
#166219,#166220,#166221,#166222,#166223,#166224,#166225,#166226,#166227,
#166228,#166229,#166230,#166231,#166232,#166233,#166234,#166235,#166236,
#166237,#166238,#166239,#166240,#166241,#166242,#166243,#166244,#166245,
#166246,#166247,#166248,#166249,#166250,#166251,#166252,#166253,#166254,
#166255,#166256,#166257,#166258,#166259,#166260,#166261,#166262,#166263,
#166264,#166265,#166266,#166267,#166268,#166269,#166270,#166271,#166272,
#166273,#166274,#166275,#166276,#166277,#166278,#166279,#166280,#166281),
 .UNSPECIFIED.,.F.,.F.,(4,2,2,2,2,2,2,2,2,2,2,2,2,2,2,2,2,2,2,2,2,2,2,2,
2,2,2,2,2,2,2,2,2,2,2,2,2,2,2,2,2,2,2,2,2,2,2,2,2,2,2,2,2,2,2,2,2,2,2,2,
2,2,2,2,4),(-2.98559501155222,-2.98150198114167,-2.97298644258405,-2.95463164891737,
-2.87704410593891,-2.69279950536456,-2.63329855246361,-2.6127254688512,
-2.59932784173563,-2.58650947868206,-2.56886663441153,-2.52603375527301,
-2.46313099303798,-2.37586575689804,-2.27328847636493,-2.25289150371308,
-2.24370288227929,-2.23661085383845,-2.22826605306425,-2.21268962008674,
-2.09266997970115,-1.93300222104418,-1.90606417573725,-1.88988079422555,
-1.87724626561229,-1.86338578543205,-1.84065252559053,-1.75052322562678,
-1.6447091884978,-1.60221390767052,-1.59627120130252,-1.51738924746365,
-1.50320025983768,-1.49542858053529,-1.48889345528827,-1.48048152497209,
-1.46267647594869,-1.38981484332574,-1.22508601237974,-1.1449703970151,
-1.12220342944022,-1.10833580321562,-1.09570342214667,-1.07926100385269,
-1.04359994854982,-0.909885413282459,-0.7793738821061,-0.75972942411144,
-0.750580439955319,-0.743504377630477,-0.73501714993527,-0.718754160922146,
-0.608988500037552,-0.438698349799292,-0.412595483209955,-0.396478855141943,
-0.383886264642389,-0.369847521045809,-0.346287165374704,-0.242897536326381,
-0.1472765080372,-0.0299220292933785,-0.0125922719991535,-0.00561123964068375,
-9.99999651085659E-7),.UNSPECIFIED.);
#30145=B_SPLINE_CURVE_WITH_KNOTS('',3,(#166282,#166283,#166284,#166285,
#166286,#166287,#166288,#166289,#166290,#166291,#166292,#166293,#166294,
#166295,#166296,#166297,#166298,#166299,#166300,#166301,#166302,#166303,
#166304,#166305,#166306,#166307,#166308,#166309,#166310,#166311,#166312,
#166313,#166314,#166315,#166316,#166317,#166318,#166319,#166320,#166321,
#166322,#166323,#166324,#166325,#166326,#166327,#166328,#166329,#166330,
#166331,#166332,#166333,#166334,#166335,#166336,#166337,#166338,#166339,
#166340,#166341,#166342,#166343,#166344,#166345,#166346,#166347,#166348,
#166349,#166350,#166351,#166352,#166353,#166354,#166355,#166356,#166357,
#166358,#166359,#166360,#166361,#166362,#166363,#166364,#166365,#166366,
#166367,#166368,#166369,#166370,#166371,#166372,#166373,#166374,#166375,
#166376,#166377,#166378,#166379,#166380,#166381,#166382,#166383,#166384,
#166385,#166386,#166387,#166388,#166389,#166390,#166391,#166392,#166393,
#166394,#166395,#166396,#166397,#166398,#166399,#166400,#166401,#166402,
#166403,#166404,#166405,#166406,#166407,#166408,#166409,#166410,#166411),
 .UNSPECIFIED.,.F.,.F.,(4,2,2,2,2,2,2,2,2,2,2,2,2,2,2,2,2,2,2,2,2,2,2,2,
2,2,2,2,2,2,2,2,2,2,2,2,2,2,2,2,2,2,2,2,2,2,2,2,2,2,2,2,2,2,2,2,2,2,2,2,
2,2,2,2,4),(-18.1752349093479,-18.1694917945602,-18.1622828023296,-18.1443097264025,
-17.9872703263121,-17.8830902947781,-17.8220212711318,-17.8019035257271,
-17.7886017324481,-17.7758716274271,-17.7580056736581,-17.7169856263102,
-17.5342909142115,-17.4794120198481,-17.4573025911209,-17.4405020101241,
-17.4319049037613,-17.4248361097276,-17.4158219926332,-17.3968965427577,
-17.254827872475,-17.1133639183328,-17.0888453045179,-17.0746042249777,
-17.062044963451,-17.0462617705439,-17.0152790027055,-16.8344193773344,
-16.7460153965524,-16.7022220974958,-16.6904417728106,-16.6832811659422,
-16.6766616260191,-16.6686285405048,-16.6480438794491,-16.5336006504433,
-16.4358128480918,-16.3694654431122,-16.3243638435582,-16.306345979109,
-16.2934599031709,-16.2801724230947,-16.2601171578566,-16.2043216964771,
-16.053818098587,-15.9688583704556,-15.9492442538141,-15.9401006618835,
-15.9336988464382,-15.9254977628865,-15.9110009495152,-15.8384879693636,
-15.7095382702265,-15.6480862356229,-15.6059566916617,-15.588424302149,
-15.575624865703,-15.5621919813025,-15.5414527579674,-15.4804967773218,
-15.298057267305,-15.2204573774013,-15.2021011181322,-15.1935852478966,
-15.1894918505391),.UNSPECIFIED.);
#30146=B_SPLINE_CURVE_WITH_KNOTS('',3,(#166413,#166414,#166415,#166416,
#166417,#166418,#166419,#166420,#166421,#166422,#166423,#166424,#166425,
#166426,#166427,#166428,#166429,#166430,#166431,#166432,#166433,#166434,
#166435,#166436,#166437,#166438,#166439,#166440,#166441,#166442,#166443,
#166444,#166445,#166446,#166447,#166448,#166449,#166450,#166451,#166452,
#166453,#166454,#166455,#166456,#166457,#166458,#166459,#166460,#166461,
#166462,#166463,#166464,#166465,#166466,#166467,#166468,#166469,#166470,
#166471,#166472,#166473,#166474,#166475,#166476,#166477,#166478,#166479,
#166480,#166481,#166482,#166483,#166484,#166485,#166486,#166487,#166488,
#166489,#166490,#166491,#166492,#166493,#166494,#166495,#166496,#166497,
#166498,#166499,#166500,#166501,#166502,#166503,#166504,#166505,#166506,
#166507,#166508,#166509,#166510,#166511,#166512,#166513,#166514,#166515,
#166516,#166517,#166518,#166519,#166520,#166521,#166522,#166523,#166524,
#166525,#166526,#166527,#166528,#166529,#166530,#166531,#166532,#166533,
#166534,#166535,#166536,#166537,#166538,#166539,#166540,#166541,#166542,
#166543,#166544,#166545,#166546,#166547,#166548,#166549,#166550,#166551,
#166552,#166553,#166554,#166555,#166556,#166557,#166558,#166559,#166560,
#166561,#166562,#166563,#166564,#166565,#166566,#166567,#166568,#166569,
#166570,#166571,#166572,#166573,#166574,#166575,#166576,#166577,#166578,
#166579,#166580,#166581,#166582,#166583,#166584,#166585,#166586,#166587,
#166588,#166589,#166590,#166591,#166592,#166593,#166594,#166595,#166596,
#166597,#166598,#166599,#166600,#166601,#166602,#166603,#166604,#166605,
#166606,#166607,#166608,#166609,#166610,#166611,#166612,#166613,#166614,
#166615,#166616,#166617,#166618,#166619,#166620,#166621,#166622,#166623,
#166624,#166625,#166626,#166627,#166628,#166629,#166630,#166631,#166632,
#166633,#166634,#166635,#166636,#166637,#166638,#166639,#166640,#166641,
#166642,#166643,#166644,#166645,#166646,#166647,#166648,#166649,#166650,
#166651,#166652,#166653,#166654,#166655,#166656,#166657,#166658,#166659,
#166660,#166661,#166662,#166663,#166664,#166665,#166666,#166667,#166668,
#166669,#166670,#166671,#166672,#166673,#166674,#166675,#166676,#166677,
#166678),.UNSPECIFIED.,.F.,.F.,(4,2,2,2,2,2,2,2,2,2,2,2,2,2,2,2,2,2,2,2,
2,2,2,2,2,2,2,2,2,2,2,2,2,2,2,2,2,2,2,2,2,2,2,2,2,2,2,2,2,2,2,2,2,2,2,2,
2,2,2,2,2,2,2,2,2,2,2,2,2,2,2,2,2,2,2,2,2,2,2,2,2,2,2,2,2,2,2,2,2,2,2,2,
2,2,2,2,2,2,2,2,2,2,2,2,2,2,2,2,2,2,2,2,2,2,2,2,2,2,2,2,2,2,2,2,2,2,2,2,
2,2,2,2,4),(-5.97113581786257,-5.96703516979956,-5.95851512437902,-5.9401366653248,
-5.8623426411769,-5.67954037707069,-5.61906809617788,-5.5983835578764,-5.58496217941587,
-5.57215643449029,-5.55458773859438,-5.51222895885169,-5.45030598444822,
-5.32232734328591,-5.24963238058043,-5.23512860741096,-5.22692591591118,
-5.22052431017789,-5.21138293579274,-5.19178101938982,-5.10693781792056,
-4.95674925962414,-4.90060919842211,-4.88050875704274,-4.86721179174308,
-4.8543318046417,-4.83634786235152,-4.79147080793593,-4.72558345883557,
-4.62720144626423,-4.5127253977237,-4.49250319162965,-4.48428327588057,
-4.47761719599568,-4.47054242167573,-4.45915145950253,-4.41957201846929,
-4.34474076754283,-4.15733451499403,-4.11882946199004,-4.10314234331012,
-4.09143700121037,-4.07853160422073,-4.06040325175182,-4.01436513329425,
-3.9446202562311,-3.80040739830392,-3.75378202972391,-3.74076905044114,
-3.73297613354094,-3.72572357546339,-3.71526964393254,-3.68767708447693,
-3.64450161772212,-3.45373144808359,-3.40531056592493,-3.38630582224035,
-3.37453779336924,-3.36168818876024,-3.34387079864031,-3.30007636261581,
-3.23638595947187,-3.1354675928041,-3.01989215553245,-2.9996451505462,-2.99142112221163,
-2.98475415599664,-2.97768154624234,-2.96629962408355,-2.92680969770483,
-2.85224733950829,-2.66590006190023,-2.62642566076004,-2.61057760629896,
-2.59883380587266,-2.58596582012182,-2.56804044398435,-2.52336307863607,
-2.45657025500021,-2.37292868558626,-2.27303609761326,-2.25273281200869,
-2.24356123296528,-2.23647112674232,-2.22811494126773,-2.21248301115083,
-2.19234534653522,-2.14481167510858,-2.051809674463,-1.92350792031644,-1.89911234172393,
-1.88489790562532,-1.87359083876238,-1.85837326087575,-1.82919505514916,
-1.72748290480389,-1.586610633051,-1.51673444542262,-1.50288442203188,-1.49518845044274,
-1.48864529902065,-1.48012996563862,-1.46177451981791,-1.38417588128721,
-1.20175612220662,-1.14081352461235,-1.12007688325711,-1.10664522153314,
-1.09384662500304,-1.0763148685492,-1.03418426671125,-0.972727660312583,
-0.843740801965002,-0.771211454106194,-0.756755952869671,-0.748564527438784,
-0.741446658718512,-0.731858433097371,-0.709753312347637,-0.67796812890868,
-0.576744370466088,-0.442416394878315,-0.411551338029357,-0.395803965344789,
-0.383248489665609,-0.368984292072017,-0.344374807045077,-0.217516004833518,
-0.0706040303832338,-0.0216738259340477,-0.00982584924864139,-0.00454025443351554,
-9.99999878459334E-7),.UNSPECIFIED.);
#30147=B_SPLINE_CURVE_WITH_KNOTS('',3,(#166679,#166680,#166681,#166682),
 .UNSPECIFIED.,.F.,.F.,(4,4),(-18.8333370051235,-18.8333271884725),
 .UNSPECIFIED.);
#30148=B_SPLINE_CURVE_WITH_KNOTS('',3,(#166687,#166688,#166689,#166690,
#166691,#166692,#166693,#166694,#166695,#166696,#166697,#166698,#166699,
#166700,#166701,#166702,#166703,#166704,#166705,#166706,#166707,#166708,
#166709,#166710,#166711,#166712,#166713,#166714,#166715,#166716,#166717,
#166718,#166719,#166720,#166721,#166722,#166723,#166724,#166725,#166726,
#166727,#166728,#166729,#166730,#166731,#166732,#166733,#166734,#166735,
#166736,#166737,#166738,#166739,#166740,#166741,#166742,#166743,#166744,
#166745,#166746,#166747,#166748,#166749,#166750,#166751,#166752,#166753,
#166754,#166755,#166756,#166757,#166758,#166759,#166760,#166761,#166762,
#166763,#166764,#166765,#166766,#166767,#166768,#166769,#166770,#166771,
#166772,#166773,#166774,#166775,#166776,#166777,#166778,#166779,#166780,
#166781,#166782,#166783,#166784,#166785,#166786,#166787,#166788,#166789,
#166790,#166791,#166792,#166793,#166794,#166795,#166796,#166797,#166798,
#166799,#166800,#166801,#166802,#166803,#166804,#166805,#166806,#166807,
#166808,#166809,#166810,#166811,#166812,#166813,#166814,#166815,#166816,
#166817,#166818,#166819,#166820,#166821,#166822,#166823,#166824,#166825,
#166826,#166827,#166828,#166829,#166830,#166831,#166832,#166833,#166834,
#166835,#166836,#166837,#166838,#166839,#166840,#166841,#166842,#166843,
#166844,#166845,#166846,#166847,#166848,#166849,#166850,#166851,#166852,
#166853,#166854,#166855,#166856,#166857,#166858,#166859,#166860,#166861,
#166862,#166863,#166864,#166865,#166866,#166867,#166868,#166869,#166870,
#166871,#166872,#166873,#166874,#166875,#166876,#166877,#166878,#166879,
#166880,#166881,#166882,#166883,#166884,#166885,#166886,#166887,#166888,
#166889,#166890,#166891,#166892,#166893,#166894,#166895,#166896,#166897,
#166898,#166899,#166900,#166901,#166902,#166903,#166904,#166905,#166906,
#166907,#166908,#166909,#166910,#166911,#166912,#166913,#166914,#166915,
#166916,#166917,#166918,#166919,#166920,#166921,#166922,#166923,#166924,
#166925,#166926,#166927,#166928,#166929,#166930,#166931,#166932,#166933,
#166934,#166935,#166936,#166937,#166938,#166939,#166940,#166941,#166942,
#166943,#166944,#166945,#166946,#166947,#166948),.UNSPECIFIED.,.F.,.F.,
(4,2,2,2,2,2,2,2,2,2,2,2,2,2,2,2,2,2,2,2,2,2,2,2,2,2,2,2,2,2,2,2,2,2,2,
2,2,2,2,2,2,2,2,2,2,2,2,2,2,2,2,2,2,2,2,2,2,2,2,2,2,2,2,2,2,2,2,2,2,2,2,
2,2,2,2,2,2,2,2,2,2,2,2,2,2,2,2,2,2,2,2,2,2,2,2,2,2,2,2,2,2,2,2,2,2,2,2,
2,2,2,2,2,2,2,2,2,2,2,2,2,2,2,2,2,2,2,2,2,2,2,4),(-8.95728479359192,-8.95319472449675,
-8.94468023383271,-8.92633397429123,-8.84883028474799,-8.66233517595378,
-8.60452255113426,-8.58414805233119,-8.57079131157462,-8.55794712790372,
-8.54016299966128,-8.49642508642479,-8.43163306182336,-8.34684859799388,
-8.24487810698112,-8.22449313291941,-8.215306077125,-8.20821354925228,-8.19986608835073,
-8.18427950485201,-8.06360244357754,-7.90467452639556,-7.87767987699411,
-7.86147954027321,-7.84884159944553,-7.83498735981955,-7.81228737062127,
-7.72265732029666,-7.61650411289081,-7.49856511562014,-7.47797657330771,
-7.4699425069411,-7.46332237256215,-7.45616138878537,-7.44438095692343,
-7.40059321091551,-7.31221339382306,-7.13130619173945,-7.10032486236829,
-7.08454124288637,-7.07198108414554,-7.05773839078626,-7.03321548194083,
-6.89158995899938,-6.74945547485728,-6.73065748832695,-6.72166720088065,
-6.71459887002994,-6.70598002412953,-6.68907398587613,-6.66678456595408,
-6.61121000187179,-6.42721250257005,-6.38768873538252,-6.37190597674247,
-6.36017722647903,-6.34729050649113,-6.3292715422203,-6.28416615324382,
-6.2178114586612,-6.12001578804295,-6.00571535221424,-5.9854962422321,-5.97727669281131,
-5.97061054338669,-5.96353523018159,-5.95214256758366,-5.91254848917706,
-5.83767454670796,-5.65010258573478,-5.61174177655313,-5.5960785818475,
-5.58437865598323,-5.57146693088284,-5.55330620761518,-5.50705014156774,
-5.43682646825714,-5.30006812615573,-5.2477056193848,-5.23418713840763,
-5.22628338385167,-5.21907998035943,-5.20890886608527,-5.1832160667927,
-5.14415746687846,-5.04146737251542,-4.90931636189658,-4.88488043077842,
-4.87065654056488,-4.85934949190088,-4.84414168417916,-4.81501604558257,
-4.71368860411346,-4.57329089134552,-4.50250234339957,-4.48861339196056,
-4.48090828422289,-4.47436556122808,-4.46586141066861,-4.44756841324618,
-4.37052476982206,-4.17093079682548,-4.12271230327394,-4.10369074462931,
-4.09192061287048,-4.07907419965218,-4.06127277836163,-4.0174158295572,
-3.95237031059405,-3.86691882248367,-3.76600549780537,-3.74565888803279,
-3.73647918287974,-3.7293879006948,-3.72103652814687,-3.70542916306244,
-3.68533273633539,-3.63794864683019,-3.54477660405748,-3.41639441498623,
-3.39199595887229,-3.37778032739539,-3.36647256806141,-3.35125439261519,
-3.3220762037064,-3.22037104968136,-3.07950049421774,-3.00959421440906,
-2.99574223024993,-2.98804552337654,-2.98559501155222),.UNSPECIFIED.);
#30149=B_SPLINE_CURVE_WITH_KNOTS('',3,(#166949,#166950,#166951,#166952,
#166953,#166954,#166955,#166956,#166957,#166958,#166959,#166960,#166961,
#166962,#166963,#166964,#166965,#166966,#166967,#166968,#166969,#166970,
#166971,#166972,#166973,#166974,#166975,#166976,#166977,#166978,#166979,
#166980,#166981,#166982,#166983,#166984,#166985,#166986,#166987,#166988,
#166989,#166990,#166991,#166992,#166993,#166994,#166995,#166996,#166997,
#166998,#166999,#167000,#167001,#167002,#167003,#167004,#167005,#167006,
#167007,#167008,#167009,#167010,#167011,#167012,#167013,#167014,#167015,
#167016,#167017,#167018,#167019,#167020,#167021,#167022,#167023,#167024,
#167025,#167026,#167027,#167028,#167029,#167030,#167031,#167032,#167033,
#167034,#167035,#167036,#167037,#167038,#167039,#167040,#167041,#167042,
#167043,#167044,#167045,#167046,#167047,#167048,#167049,#167050,#167051,
#167052,#167053,#167054,#167055,#167056,#167057,#167058,#167059,#167060,
#167061,#167062,#167063,#167064,#167065,#167066,#167067,#167068,#167069,
#167070,#167071,#167072,#167073,#167074,#167075,#167076,#167077,#167078,
#167079,#167080,#167081,#167082,#167083,#167084,#167085,#167086,#167087,
#167088,#167089,#167090,#167091,#167092,#167093,#167094,#167095,#167096,
#167097,#167098,#167099,#167100,#167101,#167102,#167103,#167104,#167105,
#167106,#167107,#167108,#167109,#167110,#167111,#167112,#167113,#167114,
#167115,#167116,#167117,#167118,#167119,#167120,#167121,#167122,#167123,
#167124,#167125,#167126,#167127,#167128,#167129,#167130,#167131,#167132,
#167133,#167134,#167135,#167136,#167137,#167138,#167139,#167140,#167141,
#167142,#167143,#167144,#167145,#167146,#167147,#167148,#167149,#167150,
#167151,#167152,#167153,#167154,#167155,#167156,#167157,#167158,#167159,
#167160,#167161,#167162,#167163,#167164,#167165,#167166,#167167,#167168,
#167169,#167170,#167171,#167172,#167173,#167174,#167175,#167176,#167177,
#167178,#167179,#167180,#167181,#167182,#167183,#167184,#167185,#167186,
#167187,#167188,#167189,#167190,#167191,#167192,#167193,#167194,#167195,
#167196,#167197,#167198,#167199,#167200,#167201,#167202,#167203,#167204,
#167205,#167206),.UNSPECIFIED.,.F.,.F.,(4,2,2,2,2,2,2,2,2,2,2,2,2,2,2,2,
2,2,2,2,2,2,2,2,2,2,2,2,2,2,2,2,2,2,2,2,2,2,2,2,2,2,2,2,2,2,2,2,2,2,2,2,
2,2,2,2,2,2,2,2,2,2,2,2,2,2,2,2,2,2,2,2,2,2,2,2,2,2,2,2,2,2,2,2,2,2,2,2,
2,2,2,2,2,2,2,2,2,2,2,2,2,2,2,2,2,2,2,2,2,2,2,2,2,2,2,2,2,2,2,2,2,2,2,2,
2,2,2,2,4),(-18.8333271884725,-18.8275940477612,-18.8203839697781,-18.8024196795371,
-18.6453570392404,-18.5411895733732,-18.4801256944877,-18.460008870824,
-18.4467075020269,-18.4339776683675,-18.4161118680451,-18.375091133818,
-18.1923737134745,-18.1375160076914,-18.1154122623847,-18.0986151018949,
-18.0900188208057,-18.0829501757085,-18.0739355756863,-18.0550068553597,
-17.9129861507796,-17.771488224752,-17.7469696911682,-17.7327288580406,
-17.720169932425,-17.7043873196533,-17.6734062048385,-17.492540611656,-17.404145715695,
-17.3603555239855,-17.3485756734211,-17.3414152873433,-17.3347958973036,
-17.3267629383907,-17.3061783015708,-17.1911532016556,-17.091763619604,
-17.0267286513643,-16.9822694059548,-16.9643495926245,-16.9514815782364,
-16.9397344228996,-16.9238730979679,-16.8842277090151,-16.7005117606719,
-16.6449853395928,-16.6227088785986,-16.6058107651318,-16.597193892138,
-16.5901259991452,-16.5811347858343,-16.5623299166487,-16.4203128318417,
-16.2786154058817,-16.2540932728942,-16.2398513787375,-16.2272921284468,
-16.2115099216185,-16.1805322523859,-15.9996063329079,-15.9112437615492,
-15.8674624103931,-15.855683074692,-15.8485226543329,-15.841902953222,-15.8338693319389,
-15.8132814509296,-15.6956110629582,-15.5898043085768,-15.4996663502823,
-15.4769319562555,-15.4630709099522,-15.450435944843,-15.434252114158,-15.4073135534577,
-15.2476220380605,-15.1276041320696,-15.1120270662866,-15.103681946473,
-15.0965896569689,-15.0874007136488,-15.0670030768978,-14.9644159953963,
-14.8771844477364,-14.8142680640235,-14.7714278774235,-14.753783490814,
-14.7409644926401,-14.7275666328729,-14.7069940650418,-14.6475023361526,
-14.4632269531374,-14.3856347370723,-14.3672790928821,-14.3587631990604,
-14.3522194038388,-14.3445224214826,-14.3306699983082,-14.2607614060004,
-14.1198964716473,-14.0181897845375,-13.9890107076789,-13.9737919930991,
-13.9624837967593,-13.9482675746057,-13.9238679997972,-13.7954778226951,
-13.7023011561734,-13.6549102029061,-13.6348116213243,-13.6192029026326,
-13.6108510494741,-13.6037595108128,-13.5945796676636,-13.5742334846981,
-13.4733444630476,-13.3879432573216,-13.3228519253627,-13.2789724969996,
-13.2611672051614,-13.2483197197274,-13.2365497775743,-13.2175311549447,
-13.1693351315456,-12.9697029535102,-12.8926450250858,-12.8743500572872,
-12.8658453317366,-12.8617719349234),.UNSPECIFIED.);
#30150=B_SPLINE_CURVE_WITH_KNOTS('',3,(#167211,#167212,#167213,#167214,
#167215,#167216,#167217,#167218,#167219,#167220,#167221,#167222,#167223,
#167224,#167225,#167226,#167227,#167228,#167229,#167230,#167231,#167232,
#167233,#167234,#167235,#167236,#167237,#167238,#167239,#167240,#167241,
#167242,#167243,#167244,#167245,#167246,#167247,#167248,#167249,#167250,
#167251,#167252,#167253,#167254,#167255,#167256,#167257,#167258,#167259,
#167260,#167261,#167262,#167263,#167264,#167265,#167266,#167267,#167268,
#167269,#167270,#167271,#167272,#167273,#167274,#167275,#167276,#167277,
#167278,#167279,#167280,#167281,#167282,#167283,#167284,#167285,#167286,
#167287,#167288,#167289,#167290,#167291,#167292,#167293,#167294,#167295,
#167296,#167297,#167298,#167299,#167300,#167301,#167302,#167303,#167304,
#167305,#167306,#167307,#167308,#167309,#167310,#167311,#167312,#167313,
#167314,#167315,#167316,#167317,#167318,#167319,#167320,#167321,#167322,
#167323,#167324,#167325,#167326,#167327,#167328,#167329,#167330,#167331,
#167332,#167333,#167334,#167335,#167336,#167337,#167338,#167339,#167340,
#167341,#167342,#167343,#167344,#167345,#167346,#167347,#167348,#167349,
#167350,#167351,#167352,#167353,#167354,#167355,#167356,#167357,#167358,
#167359,#167360,#167361,#167362,#167363,#167364,#167365,#167366,#167367,
#167368,#167369,#167370,#167371,#167372,#167373,#167374,#167375,#167376,
#167377,#167378,#167379,#167380,#167381,#167382,#167383,#167384,#167385,
#167386,#167387,#167388,#167389,#167390,#167391,#167392,#167393,#167394,
#167395,#167396,#167397,#167398,#167399,#167400,#167401,#167402,#167403,
#167404,#167405,#167406,#167407,#167408,#167409,#167410,#167411,#167412,
#167413,#167414,#167415,#167416,#167417,#167418,#167419,#167420,#167421,
#167422,#167423,#167424,#167425,#167426,#167427,#167428,#167429,#167430,
#167431,#167432,#167433,#167434,#167435,#167436,#167437,#167438,#167439,
#167440,#167441,#167442,#167443,#167444,#167445,#167446,#167447,#167448,
#167449,#167450,#167451,#167452,#167453,#167454,#167455,#167456,#167457,
#167458,#167459,#167460,#167461,#167462,#167463,#167464,#167465,#167466),
 .UNSPECIFIED.,.F.,.F.,(4,2,2,2,2,2,2,2,2,2,2,2,2,2,2,2,2,2,2,2,2,2,2,2,
2,2,2,2,2,2,2,2,2,2,2,2,2,2,2,2,2,2,2,2,2,2,2,2,2,2,2,2,2,2,2,2,2,2,2,2,
2,2,2,2,2,2,2,2,2,2,2,2,2,2,2,2,2,2,2,2,2,2,2,2,2,2,2,2,2,2,2,2,2,2,2,2,
2,2,2,2,2,2,2,2,2,2,2,2,2,2,2,2,2,2,2,2,2,2,2,2,2,2,2,2,2,2,2,4),(-14.9292022091245,
-14.923567848276,-14.9155341105952,-14.8949460842086,-14.7772119848963,
-14.6713208808229,-14.5813074281692,-14.5585814134627,-14.5447220021843,
-14.532086278869,-14.5158983704316,-14.4889460233737,-14.3294359857361,
-14.2092587418778,-14.1936792881916,-14.1853335696015,-14.1782412028746,
-14.1690527018714,-14.1486581371181,-14.0462436492217,-13.9591442328379,
-13.8960387366708,-13.8531072092446,-13.8354483602321,-13.8226266564347,
-13.8108252555576,-13.7916316878714,-13.7422707253191,-13.5444346773123,
-13.4671801679223,-13.4488627636572,-13.4403538635117,-13.4338105149843,
-13.4261082427384,-13.4122327471416,-13.3417770796311,-13.2011855204261,
-13.0997264424969,-13.0705816646625,-13.055369630315,-13.0440618000276,
-13.0298400228771,-13.0054156065968,-12.8753958462801,-12.778500397953,
-12.7345197398789,-12.7065653235143,-12.6960588499837,-12.6887963047187,
-12.6810213838878,-12.6680920382948,-12.6224112606043,-12.4766601981801,
-12.4071756784451,-12.3612548710066,-12.3431429768141,-12.330239929755,
-12.3185304465873,-12.3028283856362,-12.2642382658227,-12.0768994616907,
-12.0020816544984,-11.9625057608874,-11.951114588555,-11.9440394418029,
-11.9373728006283,-11.9291519853375,-11.908926530449,-11.7943512630132,
-11.6956862626441,-11.6300243870223,-11.5852562952438,-11.5672881231649,
-11.5544103051328,-11.5426710915306,-11.5238338682072,-11.4765392065805,
-11.2819867366182,-11.2401878322433,-11.2132200192572,-11.2028566142301,
-11.1956196884502,-11.1877918092086,-11.1746219634921,-11.126199909589,
-11.0044460772341,-10.8913054656154,-10.8610086976045,-10.8455742764201,
-10.8330399416849,-10.8185477591444,-10.7935568043138,-10.6486808977673,
-10.4995747290421,-10.4683272210659,-10.4575045034846,-10.4512436687114,
-10.4445376682149,-10.4349039388764,-10.4098576410527,-10.2759531399225,
-10.1197007614083,-10.0868019207057,-10.070854188857,-10.0582776597712,
-10.0441369193296,-10.0200926579586,-9.8991450338858,-9.7823285925319,-9.72702940003429,
-9.71330714876304,-9.70535850075845,-9.69817116751192,-9.68810144970114,
-9.66306661532859,-9.51695087688235,-9.38814289118255,-9.36373472735201,
-9.34951606401935,-9.33820730175752,-9.32298959921333,-9.29381865170373,
-9.19217652373736,-9.05135798675799,-8.98129727795255,-8.96743769117316,
-8.95973879369766,-8.95728479359192),.UNSPECIFIED.);
#30151=B_SPLINE_CURVE_WITH_KNOTS('',3,(#167467,#167468,#167469,#167470,
#167471,#167472,#167473,#167474,#167475,#167476,#167477,#167478,#167479,
#167480,#167481,#167482,#167483,#167484,#167485,#167486,#167487,#167488,
#167489,#167490,#167491,#167492,#167493,#167494,#167495,#167496,#167497,
#167498,#167499,#167500,#167501,#167502,#167503,#167504,#167505,#167506,
#167507,#167508,#167509,#167510,#167511,#167512,#167513,#167514,#167515,
#167516,#167517,#167518,#167519,#167520,#167521,#167522,#167523,#167524,
#167525,#167526,#167527,#167528,#167529,#167530,#167531,#167532,#167533,
#167534,#167535,#167536,#167537,#167538,#167539,#167540,#167541,#167542,
#167543,#167544,#167545,#167546,#167547,#167548,#167549,#167550,#167551,
#167552,#167553,#167554,#167555,#167556,#167557,#167558,#167559,#167560,
#167561,#167562,#167563,#167564,#167565,#167566,#167567,#167568,#167569,
#167570,#167571,#167572,#167573,#167574,#167575,#167576,#167577,#167578,
#167579,#167580,#167581,#167582,#167583,#167584,#167585,#167586,#167587,
#167588,#167589,#167590,#167591,#167592,#167593,#167594,#167595,#167596,
#167597,#167598,#167599,#167600,#167601,#167602,#167603,#167604,#167605,
#167606,#167607,#167608,#167609,#167610,#167611,#167612,#167613,#167614,
#167615,#167616,#167617,#167618,#167619,#167620,#167621,#167622,#167623,
#167624,#167625,#167626,#167627,#167628,#167629,#167630,#167631,#167632,
#167633,#167634,#167635,#167636,#167637,#167638,#167639,#167640,#167641,
#167642,#167643,#167644,#167645,#167646,#167647,#167648,#167649,#167650,
#167651,#167652,#167653,#167654,#167655,#167656,#167657,#167658,#167659,
#167660,#167661,#167662,#167663,#167664,#167665,#167666,#167667,#167668,
#167669,#167670,#167671,#167672,#167673,#167674,#167675,#167676,#167677,
#167678,#167679,#167680,#167681,#167682,#167683,#167684,#167685,#167686,
#167687,#167688,#167689,#167690,#167691,#167692,#167693,#167694,#167695,
#167696,#167697,#167698,#167699,#167700,#167701,#167702,#167703,#167704,
#167705,#167706,#167707,#167708,#167709,#167710,#167711,#167712,#167713,
#167714,#167715,#167716,#167717,#167718,#167719,#167720,#167721,#167722,
#167723,#167724,#167725,#167726),.UNSPECIFIED.,.F.,.F.,(4,2,2,2,2,2,2,2,
2,2,2,2,2,2,2,2,2,2,2,2,2,2,2,2,2,2,2,2,2,2,2,2,2,2,2,2,2,2,2,2,2,2,2,2,
2,2,2,2,2,2,2,2,2,2,2,2,2,2,2,2,2,2,2,2,2,2,2,2,2,2,2,2,2,2,2,2,2,2,2,2,
2,2,2,2,2,2,2,2,2,2,2,2,2,2,2,2,2,2,2,2,2,2,2,2,2,2,2,2,2,2,2,2,2,2,2,2,
2,2,2,2,2,2,2,2,2,2,2,2,2,4),(-12.8617719349234,-12.8593023241814,-12.8515970655534,
-12.8377082814962,-12.7669327203902,-12.6265298016717,-12.5251956232254,
-12.49606833127,-12.4808598072358,-12.4695522810842,-12.4553278686535,-12.4308912403472,
-12.2991307505065,-12.1995197234588,-12.1583227167709,-12.1316317780818,
-12.1213096379905,-12.1140801976905,-12.10623694004,-12.0929959929273,-12.043773588809,
-11.9016248725565,-11.8324692487148,-11.7866985870222,-11.7686087890099,
-11.7557097663079,-11.7439960831697,-11.7282766155344,-11.6895828141384,
-11.5023558809494,-11.4275661604878,-11.3879994857,-11.3766091817801,-11.3695342066581,
-11.3628674155391,-11.3546460937897,-11.3344178309401,-11.2197183683731,
-11.1207216231782,-11.0553340160798,-11.0107002159779,-10.9927524665652,
-10.9798783126377,-10.9681349984893,-10.9522932121648,-10.9127736872259,
-10.7083497078901,-10.6659936754757,-10.6387714549941,-10.6283706075608,
-10.6211269577052,-10.6133130587186,-10.6002072217801,-10.5525305406158,
-10.4302114902307,-10.3168161925509,-10.2864881132567,-10.2710474189525,
-10.2585125939678,-10.2440249727032,-10.2190547818093,-10.0776537287402,
-9.97574544739281,-9.899336844425,-9.88559839442322,-9.87800941917835,-9.87144911684368,
-9.86291555704555,-9.8446590378013,-9.68403702367608,-9.58244682924576,
-9.5223222386069,-9.50231115753956,-9.48903031329043,-9.4762839175659,-9.45833352891559,
-9.41682296164706,-9.35477089637641,-9.22897195441992,-9.15454515242283,
-9.13989428577581,-9.13165811439528,-9.12526143896965,-9.11616746861413,
-9.09682227198179,-9.01438845433282,-8.87050666068671,-8.80699307239601,
-8.7860572217461,-8.77258364035977,-8.75980291871828,-8.74239063754349,
-8.70115789900073,-8.56483678196901,-8.41530816135717,-8.3959393881213,
-8.38733031481535,-8.38076111016192,-8.37321974237346,-8.35970258424534,
-8.28855502052216,-8.18353147904001,-8.03964364301497,-8.01465295388328,
-8.00016073279213,-7.98762625014456,-7.97219150134397,-7.94189362359652,
-7.82874507750857,-7.70697846726183,-7.65856242753242,-7.64539296358926,
-7.63756511240549,-7.63032804522553,-7.61996420972807,-7.59299394905434,
-7.55119024130368,-7.3565467777315,-7.30933025176023,-7.2905047541494,-7.27876750651671,
-7.26588756893653,-7.24790841281392,-7.20306912679643,-7.13726129300237,
-7.03876501592092,-6.92424400669048,-6.90401931289166,-6.89579856302506,
-6.88983016741359),.UNSPECIFIED.);
#30152=B_SPLINE_CURVE_WITH_KNOTS('',3,(#167731,#167732,#167733,#167734,
#167735,#167736,#167737,#167738,#167739,#167740,#167741,#167742,#167743,
#167744,#167745,#167746,#167747,#167748,#167749,#167750,#167751,#167752,
#167753,#167754,#167755,#167756,#167757,#167758,#167759,#167760,#167761,
#167762,#167763,#167764,#167765,#167766,#167767,#167768,#167769,#167770,
#167771,#167772,#167773,#167774,#167775,#167776,#167777,#167778,#167779,
#167780,#167781,#167782,#167783,#167784,#167785,#167786,#167787,#167788,
#167789,#167790,#167791,#167792,#167793,#167794,#167795,#167796,#167797,
#167798,#167799,#167800,#167801,#167802,#167803,#167804,#167805,#167806,
#167807,#167808,#167809,#167810,#167811,#167812,#167813,#167814,#167815,
#167816,#167817,#167818,#167819,#167820,#167821,#167822,#167823,#167824,
#167825,#167826,#167827,#167828,#167829,#167830,#167831,#167832,#167833,
#167834,#167835,#167836,#167837,#167838,#167839,#167840,#167841,#167842,
#167843,#167844,#167845,#167846,#167847,#167848,#167849,#167850,#167851,
#167852,#167853,#167854,#167855,#167856,#167857,#167858,#167859,#167860,
#167861,#167862,#167863,#167864,#167865,#167866,#167867,#167868,#167869,
#167870,#167871,#167872,#167873,#167874,#167875,#167876,#167877,#167878,
#167879,#167880,#167881,#167882,#167883,#167884,#167885,#167886,#167887,
#167888,#167889,#167890,#167891,#167892,#167893,#167894,#167895,#167896,
#167897,#167898,#167899,#167900,#167901,#167902,#167903,#167904,#167905,
#167906,#167907,#167908,#167909,#167910,#167911,#167912,#167913,#167914,
#167915,#167916,#167917,#167918,#167919,#167920,#167921,#167922,#167923,
#167924,#167925,#167926,#167927,#167928,#167929,#167930,#167931,#167932,
#167933,#167934,#167935,#167936,#167937,#167938,#167939,#167940,#167941,
#167942,#167943,#167944,#167945,#167946,#167947,#167948,#167949,#167950,
#167951,#167952,#167953,#167954,#167955,#167956,#167957,#167958,#167959,
#167960,#167961,#167962,#167963,#167964,#167965,#167966,#167967,#167968,
#167969,#167970,#167971,#167972,#167973,#167974,#167975,#167976,#167977,
#167978,#167979,#167980,#167981,#167982,#167983,#167984,#167985,#167986,
#167987,#167988,#167989,#167990),.UNSPECIFIED.,.F.,.F.,(4,2,2,2,2,2,2,2,
2,2,2,2,2,2,2,2,2,2,2,2,2,2,2,2,2,2,2,2,2,2,2,2,2,2,2,2,2,2,2,2,2,2,2,2,
2,2,2,2,2,2,2,2,2,2,2,2,2,2,2,2,2,2,2,2,2,2,2,2,2,2,2,2,2,2,2,2,2,2,2,2,
2,2,2,2,2,2,2,2,2,2,2,2,2,2,2,2,2,2,2,2,2,2,2,2,2,2,2,2,2,2,2,2,2,2,2,2,
2,2,2,2,2,2,2,2,2,2,2,2,2,4),(-20.9006012202032,-20.9001713274698,-20.8931717655193,
-20.8821215261626,-20.8491311403437,-20.6723703761679,-20.5554857242621,
-20.5312640626005,-20.5170832713651,-20.5045162344918,-20.4886402304745,
-20.46335858551,-20.2855464468007,-20.2606342106676,-20.2051108428453,-20.1828357216655,
-20.1659386604881,-20.1573223608734,-20.1502549590852,-20.1412643971362,
-20.1224609782449,-19.9804519675184,-19.8387658755263,-19.8142454645421,
-19.8000045625636,-19.7874461825262,-19.7716650630128,-19.7406895076086,
-19.5597765529035,-19.4714198381321,-19.427641443944,-19.4158629181493,
-19.4087029927893,-19.4020837514475,-19.394050690327,-19.3734642567595,
-19.2557971422429,-19.1499911356937,-19.0598695108081,-19.0371373970091,
-19.0232774638021,-19.0106433339887,-18.9944603255084,-18.9675225755179,
-18.8078568045629,-18.6878347478868,-18.6722585963133,-18.6639140204238,
-18.6568222275419,-18.6476339708278,-18.6272380245924,-18.524672664206,
-18.4373387556432,-18.3744826699684,-18.3316724264722,-18.3140334760254,
-18.30121609886,-18.2894116798905,-18.2701973403491,-18.2206891858261,-18.02308286435,
-17.9458270936638,-17.9275103897592,-17.9190020728669,-17.9124592911764,
-17.9047578257945,-17.8908841094032,-17.8204478463093,-17.6798613297729,
-17.578405869207,-17.5492629245707,-17.5340520893621,-17.5227452498584,
-17.5085248488967,-17.4841031272564,-17.3541406182398,-17.2572377856411,
-17.2132418255269,-17.1852813098867,-17.1747745418703,-17.1675124160736,
-17.159738620634,-17.1468124030856,-17.1011576398705,-16.9554451076541,
-16.8859350592151,-16.8400038759811,-16.8218914626414,-16.8089891702259,
-16.7972811244549,-16.7815821181825,-16.7427129174984,-16.5555966950846,
-16.4808374821355,-16.4412822773744,-16.4298937963868,-16.4228196488019,
-16.4161533791638,-16.4079324339744,-16.3877038028021,-16.2729139990718,
-16.1736785289361,-16.1085075153986,-16.0639811768673,-16.0460508824072,
-16.033180786685,-16.0214354292174,-16.00558215487,-15.9659871155828,-15.7822086477371,
-15.7266708932671,-15.7043913636228,-15.6874913849516,-15.6788740340354,
-15.6718060178269,-15.6628149885053,-15.6440116358243,-15.5019690116316,
-15.3602881984508,-15.3357658661288,-15.3215237544323,-15.3089642519043,
-15.293181647654,-15.2622029365615,-15.0812788830013,-14.9929111169226,
-14.9491279008498,-14.9373482475801,-14.9301876685023,-14.9292022091245),
 .UNSPECIFIED.);
#30153=B_SPLINE_CURVE_WITH_KNOTS('',3,(#167991,#167992,#167993,#167994,
#167995,#167996,#167997,#167998,#167999,#168000,#168001,#168002,#168003,
#168004,#168005,#168006,#168007,#168008,#168009,#168010,#168011,#168012,
#168013,#168014,#168015,#168016,#168017,#168018,#168019,#168020,#168021,
#168022,#168023,#168024,#168025,#168026,#168027,#168028,#168029,#168030,
#168031,#168032,#168033,#168034,#168035,#168036,#168037,#168038,#168039,
#168040,#168041,#168042,#168043,#168044,#168045,#168046,#168047,#168048,
#168049,#168050,#168051,#168052,#168053,#168054,#168055,#168056,#168057,
#168058,#168059,#168060,#168061,#168062,#168063,#168064,#168065,#168066,
#168067,#168068,#168069,#168070,#168071,#168072,#168073,#168074,#168075,
#168076,#168077,#168078,#168079,#168080,#168081,#168082,#168083,#168084,
#168085,#168086,#168087,#168088,#168089,#168090,#168091,#168092,#168093,
#168094,#168095,#168096,#168097,#168098,#168099,#168100,#168101,#168102,
#168103,#168104,#168105,#168106,#168107,#168108,#168109,#168110,#168111,
#168112,#168113,#168114,#168115,#168116,#168117,#168118,#168119,#168120,
#168121,#168122,#168123,#168124,#168125,#168126,#168127,#168128,#168129,
#168130,#168131,#168132,#168133,#168134,#168135,#168136,#168137,#168138,
#168139,#168140,#168141,#168142,#168143,#168144,#168145,#168146,#168147,
#168148,#168149,#168150,#168151,#168152,#168153,#168154,#168155,#168156,
#168157,#168158,#168159,#168160,#168161,#168162,#168163,#168164,#168165,
#168166,#168167,#168168,#168169,#168170,#168171,#168172,#168173,#168174,
#168175,#168176,#168177,#168178,#168179,#168180,#168181,#168182,#168183,
#168184,#168185,#168186,#168187,#168188,#168189,#168190,#168191,#168192,
#168193,#168194,#168195,#168196,#168197,#168198,#168199,#168200,#168201,
#168202,#168203,#168204,#168205,#168206,#168207,#168208,#168209,#168210,
#168211,#168212,#168213,#168214,#168215,#168216,#168217,#168218,#168219,
#168220,#168221,#168222,#168223,#168224,#168225,#168226,#168227,#168228,
#168229,#168230,#168231,#168232,#168233,#168234,#168235,#168236,#168237,
#168238,#168239,#168240,#168241,#168242,#168243,#168244,#168245,#168246,
#168247,#168248,#168249,#168250,#168251,#168252),.UNSPECIFIED.,.F.,.F.,
(4,2,2,2,2,2,2,2,2,2,2,2,2,2,2,2,2,2,2,2,2,2,2,2,2,2,2,2,2,2,2,2,2,2,2,
2,2,2,2,2,2,2,2,2,2,2,2,2,2,2,2,2,2,2,2,2,2,2,2,2,2,2,2,2,2,2,2,2,2,2,2,
2,2,2,2,2,2,2,2,2,2,2,2,2,2,2,2,2,2,2,2,2,2,2,2,2,2,2,2,2,2,2,2,2,2,2,2,
2,2,2,2,2,2,2,2,2,2,2,2,2,2,2,2,2,2,2,2,2,2,2,4),(-6.88983016741359,-6.88913187945072,
-6.88205655671293,-6.87066487676115,-6.83108467296479,-6.75625495688335,
-6.56886418117328,-6.53027002139335,-6.51459700351551,-6.50289434311178,
-6.48998415268692,-6.4718342803467,-6.42565615619463,-6.35560590871231,
-6.21578913304267,-6.16583993697248,-6.15250743531802,-6.1446440885681,
-6.13742341550088,-6.12715205788757,-6.10080113134887,-6.06033902727961,
-5.95983271440256,-5.82778172939104,-5.80334462110304,-5.78912002043135,
-5.77781239346956,-5.76260379046175,-5.73347656809926,-5.63214325597553,
-5.49173722693558,-5.4209469594796,-5.40705737814925,-5.39935189510391,
-5.39280883646972,-5.38430422767557,-5.36601016540622,-5.28896143768228,
-5.08935389687434,-5.04113647014719,-5.0221144770105,-5.01034384103868,
-4.99749669163258,-4.97969390512581,-4.93583173165814,-4.87077658430402,
-4.78532759720732,-4.6844124882172,-4.66406498299851,-4.6548848352987,-4.6477931940593,
-4.63944137778573,-4.62383313110876,-4.60373553696183,-4.55634851930268,
-4.46317227607844,-4.33478378698708,-4.31038409151202,-4.2961677363078,
-4.28485940041794,-4.26964044790941,-4.24046076520245,-4.13875038094999,
-3.9978726072158,-3.92796285072478,-3.91411016406304,-3.90641306564974,
-3.89986918837637,-3.89135321171877,-3.87299747003301,-3.79540589136508,
-3.6111522481167,-3.55164796341351,-3.53107379195006,-3.51767547057735,
-3.50485645359576,-3.48721272592217,-3.44437778906765,-3.38147208978702,
-3.29420172201006,-3.19161934222916,-3.17122132608957,-3.16203223373006,
-3.15493984144054,-3.14659461208925,-3.13101737798728,-3.01099143845297,
-2.85131565252643,-2.82437621305624,-2.80819199776416,-2.79555682039172,
-2.78169563072154,-2.7589612123388,-2.66882740144109,-2.56300786050056,
-2.4453266069816,-2.42473805582632,-2.41670424819144,-2.41008442896301,
-2.40292391733999,-2.39114451031011,-2.34736358150708,-2.25900381099065,
-2.07808271695856,-2.04710499079443,-2.03132262104751,-2.01876317554152,
-2.00452099006845,-1.9799981858713,-1.83829539055137,-1.69626853256855,
-1.67746325548576,-1.66847186983495,-1.66140385800443,-1.6527868476265,
-1.63588850664463,-1.61361192701009,-1.55808564607875,-1.37436955231147,
-1.33472785306068,-1.31886697147818,-1.30711978196907,-1.29425137666648,
-1.27633036569073,-1.23186467230361,-1.16681634436809,-1.06744511505669,
-0.952573777543494,-0.93234314610872,-0.924121854583241,-0.918151647035043),
 .UNSPECIFIED.);
#30154=B_SPLINE_CURVE_WITH_KNOTS('',3,(#168257,#168258,#168259,#168260,
#168261,#168262,#168263,#168264,#168265,#168266,#168267,#168268,#168269,
#168270,#168271,#168272,#168273,#168274,#168275,#168276,#168277,#168278),
 .UNSPECIFIED.,.F.,.F.,(4,2,2,2,2,2,2,2,2,2,4),(5.94644245477199,6.60767518318918,
7.16805975801899,7.45354600572087,8.24302433165703,8.85682530139938,9.73093935598426,
10.4069887989121,10.7296063241796,11.5427165923998,12.1931059899322),
 .UNSPECIFIED.);
#30155=B_SPLINE_CURVE_WITH_KNOTS('',3,(#168285,#168286,#168287,#168288,
#168289,#168290,#168291,#168292,#168293,#168294,#168295,#168296,#168297,
#168298,#168299,#168300,#168301,#168302,#168303,#168304,#168305,#168306,
#168307,#168308,#168309,#168310,#168311,#168312,#168313,#168314,#168315,
#168316,#168317,#168318,#168319,#168320,#168321,#168322,#168323,#168324,
#168325,#168326,#168327,#168328,#168329,#168330,#168331,#168332,#168333,
#168334,#168335,#168336,#168337,#168338,#168339,#168340,#168341,#168342,
#168343,#168344,#168345,#168346,#168347,#168348,#168349,#168350,#168351,
#168352,#168353,#168354,#168355,#168356,#168357,#168358,#168359,#168360,
#168361,#168362,#168363,#168364,#168365,#168366,#168367,#168368,#168369,
#168370,#168371,#168372,#168373,#168374,#168375,#168376,#168377,#168378,
#168379,#168380,#168381,#168382,#168383,#168384,#168385,#168386,#168387,
#168388,#168389,#168390,#168391,#168392,#168393,#168394,#168395,#168396,
#168397,#168398,#168399,#168400,#168401,#168402,#168403,#168404,#168405,
#168406,#168407,#168408,#168409,#168410,#168411,#168412,#168413,#168414,
#168415,#168416,#168417,#168418,#168419,#168420,#168421,#168422,#168423,
#168424,#168425,#168426,#168427,#168428,#168429,#168430,#168431,#168432,
#168433,#168434,#168435,#168436,#168437,#168438,#168439,#168440,#168441,
#168442,#168443,#168444,#168445,#168446,#168447,#168448,#168449,#168450,
#168451,#168452,#168453,#168454),.UNSPECIFIED.,.F.,.F.,(4,2,2,2,2,2,2,2,
2,2,2,2,2,2,2,2,2,2,2,2,2,2,2,2,2,2,2,2,2,2,2,2,2,2,2,2,2,2,2,2,2,2,2,2,
2,2,2,2,2,2,2,2,2,2,2,2,2,2,2,2,2,2,2,2,2,2,2,2,2,2,2,2,2,2,2,2,2,2,2,2,
2,2,2,2,4),(6.28535341527715,6.2882021757388,6.29605541836851,6.31102864908079,
6.43737275494601,6.63842224468773,6.66961171887247,6.68545158990087,6.69801645538159,
6.71220958836953,6.7364685902245,6.85630095703125,6.94659497629758,6.99453804280581,
7.04788912249746,7.06155273754703,7.06949213793895,7.07666834134776,7.08667011430709,
7.11120329448208,7.1476244638425,7.27630821386669,7.40475824841285,7.42926164513167,
7.44364646837022,7.45618756100137,7.47174426974938,7.50255643735899,7.61491829777165,
7.77285165013532,7.83346066295643,7.84687487291156,7.85447634465023,7.86036935737998,
7.8686049787064,7.88546936373978,8.02338035809764,8.20747132524815,8.24052449108624,
8.25651548122264,8.26909538961242,8.28319562460639,8.3070237362241,8.41671539152207,
8.54804794796548,8.61753783005534,8.63199261912393,8.64018895056254,8.64658274565332,
8.65566809018836,8.6749299946092,8.75544417864585,8.95913615221126,8.99437645690017,
9.01058745452713,9.02322647636245,9.03706252120184,9.05965723658158,9.14635359296998,
9.34916066368639,9.40547507906998,9.41862132410928,9.42616183785918,9.43206403156523,
9.44038584770225,9.45769282285902,9.54606472904573,9.68702931575528,9.79297945277671,
9.81732212763114,9.83167508673994,9.84421940676834,9.85982122175962,9.89090303956229,
10.0085276021679,10.1331155412817,10.1902336610209,10.2041589880414,10.2121554877834,
10.2193127852824,10.2291918164983,10.2529662604549,10.2878607508683,10.4008697061023,
10.5463583837695),.UNSPECIFIED.);
#30156=B_SPLINE_CURVE_WITH_KNOTS('',3,(#168457,#168458,#168459,#168460,
#168461,#168462,#168463,#168464,#168465,#168466,#168467,#168468,#168469,
#168470,#168471,#168472,#168473,#168474,#168475,#168476,#168477,#168478,
#168479,#168480,#168481,#168482,#168483,#168484,#168485,#168486,#168487,
#168488,#168489,#168490,#168491,#168492,#168493,#168494,#168495,#168496,
#168497,#168498,#168499,#168500,#168501,#168502,#168503,#168504,#168505,
#168506,#168507,#168508,#168509,#168510,#168511,#168512,#168513,#168514,
#168515,#168516,#168517,#168518,#168519,#168520,#168521,#168522,#168523,
#168524,#168525,#168526,#168527,#168528,#168529,#168530,#168531,#168532,
#168533,#168534,#168535,#168536,#168537,#168538,#168539,#168540,#168541,
#168542,#168543,#168544,#168545,#168546,#168547,#168548,#168549,#168550,
#168551,#168552,#168553,#168554,#168555,#168556,#168557,#168558,#168559,
#168560,#168561,#168562,#168563,#168564,#168565,#168566,#168567,#168568,
#168569,#168570,#168571,#168572,#168573,#168574,#168575,#168576,#168577,
#168578,#168579,#168580,#168581,#168582,#168583,#168584,#168585,#168586,
#168587,#168588,#168589,#168590,#168591,#168592,#168593,#168594,#168595,
#168596,#168597,#168598,#168599,#168600,#168601,#168602,#168603,#168604,
#168605,#168606,#168607,#168608,#168609,#168610,#168611,#168612,#168613,
#168614,#168615,#168616,#168617,#168618,#168619,#168620,#168621,#168622,
#168623,#168624,#168625,#168626),.UNSPECIFIED.,.F.,.F.,(4,2,2,2,2,2,2,2,
2,2,2,2,2,2,2,2,2,2,2,2,2,2,2,2,2,2,2,2,2,2,2,2,2,2,2,2,2,2,2,2,2,2,2,2,
2,2,2,2,2,2,2,2,2,2,2,2,2,2,2,2,2,2,2,2,2,2,2,2,2,2,2,2,2,2,2,2,2,2,2,2,
2,2,2,2,4),(1.00000001185263E-6,0.150101630938482,0.170066194866638,0.179282640036017,
0.186361094252854,0.194748588751972,0.210058493834735,0.316330590351473,
0.435034177154938,0.521604396572538,0.544106270412088,0.557919985969065,
0.570565783326518,0.586820611551792,0.622241305541521,0.84800481608078,
0.913931869336241,0.950727236159845,0.961855658571001,0.968875094076227,
0.975562470997592,0.983858611106606,1.00475445095198,1.12080859978613,1.21725245728034,
1.33448460862351,1.3589192729214,1.37315386374228,1.38571315148011,1.40149051951235,
1.43347410104357,1.58431113222412,1.64004883439538,1.72963380932092,1.74455462876196,
1.75276600851946,1.75987086077602,1.76919159027147,1.79028359486636,1.9026442337869,
2.00292651393419,2.06259211451374,2.10406030440563,2.12151597717192,2.13430430318827,
2.14614602816371,2.16554724661403,2.21600599884866,2.41998820713048,2.48550210351074,
2.52214600587198,2.53325856796103,2.54027469808609,2.5469647451392,2.55527026966158,
2.5762216464443,2.69549981884673,2.81463287731623,2.90837872677946,2.9314844011882,
2.94543206021137,2.958044291966,2.97431291194609,3.00088446214869,3.20676318283083,
3.29314567079042,3.31305386420129,3.32226044982287,3.32933874691901,3.33773489966039,
3.35308167124301,3.46207783141478,3.5408332891298,3.661231340971,3.68551358051179,
3.69971254026873,3.71227789042278,3.72811210673465,3.76034118921313,3.95468021994065,
3.98625084726419,4.08243792313468,4.10007838852451,4.10846490510006,4.11237294021447),
 .UNSPECIFIED.);
#30157=B_SPLINE_CURVE_WITH_KNOTS('',3,(#168631,#168632,#168633,#168634,
#168635,#168636,#168637,#168638,#168639,#168640,#168641,#168642,#168643,
#168644,#168645,#168646,#168647,#168648,#168649,#168650,#168651,#168652,
#168653,#168654,#168655,#168656,#168657,#168658,#168659,#168660,#168661,
#168662,#168663,#168664,#168665,#168666,#168667,#168668,#168669,#168670,
#168671,#168672,#168673,#168674,#168675,#168676,#168677,#168678,#168679,
#168680,#168681,#168682,#168683,#168684,#168685,#168686,#168687,#168688,
#168689,#168690,#168691,#168692,#168693,#168694,#168695,#168696,#168697,
#168698,#168699,#168700,#168701,#168702,#168703,#168704,#168705,#168706,
#168707,#168708,#168709,#168710,#168711,#168712,#168713,#168714,#168715,
#168716,#168717,#168718,#168719,#168720,#168721,#168722,#168723,#168724,
#168725,#168726,#168727,#168728,#168729,#168730,#168731,#168732,#168733,
#168734,#168735,#168736,#168737,#168738,#168739,#168740,#168741,#168742,
#168743,#168744,#168745,#168746,#168747,#168748,#168749,#168750,#168751,
#168752,#168753,#168754,#168755,#168756,#168757,#168758,#168759,#168760,
#168761,#168762,#168763,#168764,#168765,#168766,#168767,#168768,#168769,
#168770,#168771,#168772,#168773,#168774,#168775,#168776,#168777,#168778,
#168779,#168780,#168781,#168782,#168783,#168784,#168785,#168786,#168787,
#168788,#168789,#168790,#168791,#168792,#168793,#168794,#168795,#168796,
#168797,#168798,#168799,#168800,#168801,#168802,#168803,#168804,#168805,
#168806,#168807,#168808,#168809,#168810,#168811,#168812,#168813,#168814,
#168815,#168816,#168817,#168818,#168819,#168820,#168821,#168822,#168823,
#168824,#168825,#168826,#168827,#168828,#168829,#168830,#168831,#168832,
#168833,#168834,#168835,#168836,#168837,#168838,#168839,#168840,#168841,
#168842,#168843,#168844,#168845,#168846,#168847,#168848,#168849,#168850,
#168851,#168852,#168853,#168854,#168855,#168856,#168857,#168858,#168859,
#168860,#168861,#168862,#168863,#168864,#168865,#168866,#168867,#168868,
#168869,#168870,#168871,#168872,#168873,#168874,#168875,#168876,#168877,
#168878,#168879,#168880,#168881,#168882,#168883,#168884,#168885,#168886,
#168887,#168888,#168889,#168890,#168891,#168892,#168893,#168894,#168895,
#168896,#168897,#168898,#168899,#168900,#168901,#168902),.UNSPECIFIED.,
 .F.,.F.,(4,2,2,2,2,2,2,2,2,2,2,2,2,2,2,2,2,2,2,2,2,2,2,2,2,2,2,2,2,2,2,
2,2,2,2,2,2,2,2,2,2,2,2,2,2,2,2,2,2,2,2,2,2,2,2,2,2,2,2,2,2,2,2,2,2,2,2,
2,2,2,2,2,2,2,2,2,2,2,2,2,2,2,2,2,2,2,2,2,2,2,2,2,2,2,2,2,2,2,2,2,2,2,2,
2,2,2,2,2,2,2,2,2,2,2,2,2,2,2,2,2,2,2,2,2,2,2,2,2,2,2,2,2,2,2,2,4),(9.99999999287575E-7,
0.00579850576153826,0.0130944527428375,0.0312216908045841,0.163439922679926,
0.283087003150158,0.339763914128201,0.380142608406775,0.397437276560381,
0.410198455738976,0.422080475513747,0.441697421133798,0.493971521459607,
0.676471733323956,0.753758194362052,0.772650638227882,0.781665847663628,
0.788051868319968,0.796296770705438,0.81096749919682,0.885366770739691,
1.01994513665708,1.08770771085909,1.13312676587809,1.15119793582843,1.16409485308743,
1.1758052929941,1.19150611991899,1.22216538739257,1.3900571992775,1.48397377965424,
1.5485818796735,1.56183522765093,1.56932203819386,1.57589345274377,1.58453343338458,
1.60404586310083,1.76897444173588,1.9080950100385,1.9506200734075,1.96826493692671,
1.98108579046468,1.99447300352144,2.01498659070443,2.07385730127611,2.24945901727584,
2.3253583410306,2.34408872720265,2.35307295373937,2.35945578029628,2.36772302362599,
2.38249325130372,2.45845701526486,2.59112407090777,2.65899065332678,2.7044588852972,
2.72253748740991,2.73543581242198,2.7471449159159,2.7628400386619,2.80128879284624,
3.00159230559794,3.02120568491813,3.08719297854698,3.12401020127794,3.13514080317366,
3.14216062614208,3.14884751616431,3.15714215977869,3.17802955164812,3.30232441387236,
3.41284103904473,3.47702967743191,3.52128993031315,3.53920839103398,3.55207833050819,
3.5638205452224,3.58266524932496,3.62972081729748,3.81840317907358,3.89636745759488,
3.91533878679841,3.92436925730299,3.93075713430037,3.93899184877964,3.95361631767279,
4.02580908780727,4.16285994804546,4.23052055026061,4.27589195482301,4.29395642310159,
4.30685250034773,4.31856482546026,4.3342721450285,4.36495623236491,4.52847566179826,
4.59036293734492,4.65786274620942,4.69523138105016,4.70642031242063,4.71345305817074,
4.72013168762499,4.72839469380622,4.748843539932,4.89135152044875,5.01667084527042,
5.0625835962627,5.09701600028071,5.1132662608486,5.12587601579613,5.13983170110593,
5.16298891662328,5.24872203885499,5.2729098659224,5.40421699200536,5.41407604116132,
5.47550495518287,5.48954889310835,5.49765233942526,5.50478027069231,5.51445064472022,
5.53697449813832,5.56940984470954,5.67197838103664,5.82120496738593,5.85324470132735,
5.86903283780541,5.88159303574035,5.89582048127871,5.92022221704508,6.03674823352164,
6.17586231118275,6.26019775401805,6.27341835675887,6.28167831501583,6.28535341527715),
 .UNSPECIFIED.);
#30158=B_SPLINE_CURVE_WITH_KNOTS('',3,(#168903,#168904,#168905,#168906,
#168907,#168908,#168909,#168910,#168911,#168912,#168913,#168914,#168915,
#168916,#168917,#168918,#168919,#168920,#168921,#168922,#168923,#168924,
#168925,#168926,#168927,#168928,#168929,#168930,#168931,#168932,#168933,
#168934,#168935,#168936,#168937,#168938,#168939,#168940,#168941,#168942,
#168943,#168944,#168945,#168946,#168947,#168948,#168949,#168950,#168951,
#168952,#168953,#168954,#168955,#168956,#168957,#168958,#168959,#168960,
#168961,#168962,#168963,#168964,#168965,#168966,#168967,#168968,#168969,
#168970,#168971,#168972,#168973,#168974,#168975,#168976,#168977,#168978,
#168979,#168980,#168981,#168982,#168983,#168984,#168985,#168986,#168987,
#168988,#168989,#168990,#168991,#168992,#168993,#168994,#168995,#168996,
#168997,#168998,#168999,#169000,#169001,#169002,#169003,#169004,#169005,
#169006,#169007,#169008,#169009,#169010,#169011,#169012,#169013,#169014,
#169015,#169016,#169017,#169018,#169019,#169020,#169021,#169022,#169023,
#169024,#169025,#169026,#169027,#169028,#169029,#169030,#169031,#169032,
#169033,#169034,#169035,#169036,#169037,#169038,#169039,#169040,#169041,
#169042,#169043,#169044,#169045,#169046,#169047,#169048,#169049,#169050,
#169051,#169052,#169053,#169054,#169055,#169056,#169057,#169058,#169059,
#169060,#169061,#169062,#169063,#169064,#169065,#169066,#169067,#169068,
#169069,#169070,#169071,#169072,#169073,#169074,#169075,#169076,#169077,
#169078,#169079,#169080,#169081,#169082,#169083,#169084,#169085,#169086,
#169087,#169088,#169089,#169090,#169091,#169092,#169093,#169094,#169095,
#169096,#169097,#169098,#169099,#169100,#169101,#169102,#169103,#169104,
#169105,#169106,#169107,#169108,#169109,#169110,#169111,#169112,#169113,
#169114,#169115,#169116,#169117,#169118,#169119,#169120,#169121,#169122,
#169123,#169124,#169125,#169126,#169127,#169128,#169129,#169130,#169131,
#169132,#169133,#169134,#169135,#169136,#169137,#169138,#169139,#169140,
#169141,#169142,#169143,#169144,#169145,#169146,#169147,#169148,#169149,
#169150,#169151,#169152,#169153,#169154),.UNSPECIFIED.,.F.,.F.,(4,2,2,2,
2,2,2,2,2,2,2,2,2,2,2,2,2,2,2,2,2,2,2,2,2,2,2,2,2,2,2,2,2,2,2,2,2,2,2,2,
2,2,2,2,2,2,2,2,2,2,2,2,2,2,2,2,2,2,2,2,2,2,2,2,2,2,2,2,2,2,2,2,2,2,2,2,
2,2,2,2,2,2,2,2,2,2,2,2,2,2,2,2,2,2,2,2,2,2,2,2,2,2,2,2,2,2,2,2,2,2,2,2,
2,2,2,2,2,2,2,2,2,2,2,2,2,4),(4.11237294021447,4.11499671540717,4.12275024725038,
4.13683830501483,4.20978481128889,4.35604088880456,4.46691615971153,4.49752961927095,
4.51304796272934,4.52558752430315,4.54000297149108,4.56463849871281,4.70111758557034,
4.82312637138642,4.85861870830937,4.88269262212078,4.89262103687441,4.89978637009214,
4.90776066981282,4.92158188465078,4.97712479566213,5.12304864411524,5.23352835707963,
5.25739535856455,5.27150488114816,5.28408466278652,5.30006401991669,5.333050898281,
5.5181062787572,5.65345504765757,5.67143550863331,5.67988672844655,5.6864234272891,
5.69412908227144,5.70800319637131,5.77711412488523,5.934056353816,6.04921965618755,
6.07355850453487,6.08777303761054,6.1003361048332,6.11614692858305,6.14830104965685,
6.28008600210841,6.42798092955698,6.45365732446582,6.46383937666132,6.47104577798304,
6.47890933151204,6.49222419299424,6.54163787607225,6.69229401929071,6.80493120638159,
6.82889626978474,6.84302694337066,6.85560310826527,6.87154732706019,6.90434975836392,
7.09179331270864,7.22950648522972,7.2446744633357,7.25256853281062,7.25909094906039,
7.26730456963467,7.28036948296626,7.35908002395987,7.50405901090792,7.62067937323755,
7.64508719825605,7.65931671199228,7.67187784592876,7.6876659723343,7.71970146956426,
7.86898929485801,7.97152845851285,8.00395985205691,8.0264822770266,8.03615289547914,
8.04328135068401,8.05138578328401,8.06543225656834,8.12688992260981,8.15132715251319,
8.2596074085133,8.37615632891564,8.40028841541381,8.4144552245251,8.42702575626741,
8.44291177725569,8.4754092597276,8.66657758043566,8.80098951246528,8.81619630230322,
8.82409848938872,8.83062069222283,8.83882534150094,8.85186014475097,8.92965837482495,
9.07493776300742,9.19218121001687,9.21661824665642,9.23085422137612,9.24341473125934,
9.25919363608272,9.29118033834613,9.44306193458432,9.54367339790887,9.57577175484967,
9.59812209770917,9.60776344964721,9.6148881825251,9.62300890999991,9.63712669646708,
9.69989933794189,9.8206613702415,9.94708314232956,9.97157566291891,9.98582009690826,
9.99837945079697,10.0141445049674,10.0460144784218,10.2807586240382,10.3693192933289,
10.386629671906,10.394952971852,10.398744700606),.UNSPECIFIED.);
#30159=B_SPLINE_CURVE_WITH_KNOTS('',3,(#169159,#169160,#169161,#169162,
#169163,#169164,#169165,#169166,#169167,#169168,#169169,#169170,#169171,
#169172,#169173,#169174,#169175,#169176,#169177,#169178,#169179,#169180,
#169181,#169182,#169183,#169184,#169185,#169186,#169187,#169188,#169189,
#169190,#169191,#169192,#169193,#169194,#169195,#169196,#169197,#169198,
#169199,#169200,#169201,#169202,#169203,#169204,#169205,#169206,#169207,
#169208,#169209,#169210,#169211,#169212,#169213,#169214,#169215,#169216,
#169217,#169218,#169219,#169220,#169221,#169222,#169223,#169224,#169225,
#169226,#169227,#169228,#169229,#169230,#169231,#169232,#169233,#169234,
#169235,#169236,#169237,#169238,#169239,#169240,#169241,#169242,#169243,
#169244,#169245,#169246,#169247,#169248,#169249,#169250,#169251,#169252,
#169253,#169254,#169255,#169256,#169257,#169258,#169259,#169260,#169261,
#169262,#169263,#169264,#169265,#169266,#169267,#169268,#169269,#169270,
#169271,#169272,#169273,#169274,#169275,#169276,#169277,#169278,#169279,
#169280,#169281,#169282,#169283,#169284,#169285,#169286,#169287,#169288,
#169289,#169290,#169291,#169292,#169293,#169294,#169295,#169296,#169297,
#169298,#169299,#169300,#169301,#169302,#169303,#169304,#169305,#169306,
#169307,#169308,#169309,#169310,#169311,#169312,#169313,#169314,#169315,
#169316,#169317,#169318,#169319,#169320,#169321,#169322,#169323,#169324,
#169325,#169326,#169327,#169328,#169329,#169330,#169331,#169332,#169333,
#169334,#169335,#169336,#169337,#169338,#169339,#169340,#169341,#169342,
#169343,#169344,#169345,#169346,#169347,#169348,#169349,#169350,#169351,
#169352,#169353,#169354,#169355,#169356,#169357,#169358,#169359,#169360,
#169361,#169362,#169363,#169364,#169365,#169366,#169367,#169368,#169369,
#169370,#169371,#169372,#169373,#169374,#169375,#169376,#169377,#169378,
#169379,#169380,#169381,#169382,#169383,#169384,#169385,#169386,#169387,
#169388,#169389,#169390,#169391,#169392,#169393,#169394,#169395,#169396,
#169397,#169398,#169399,#169400,#169401,#169402,#169403,#169404,#169405,
#169406,#169407,#169408,#169409,#169410),.UNSPECIFIED.,.F.,.F.,(4,2,2,2,
2,2,2,2,2,2,2,2,2,2,2,2,2,2,2,2,2,2,2,2,2,2,2,2,2,2,2,2,2,2,2,2,2,2,2,2,
2,2,2,2,2,2,2,2,2,2,2,2,2,2,2,2,2,2,2,2,2,2,2,2,2,2,2,2,2,2,2,2,2,2,2,2,
2,2,2,2,2,2,2,2,2,2,2,2,2,2,2,2,2,2,2,2,2,2,2,2,2,2,2,2,2,2,2,2,2,2,2,2,
2,2,2,2,2,2,2,2,2,2,2,2,2,4),(17.0758907305399,17.0798166350792,17.0882129209521,
17.105905153377,17.2444158663091,17.426428078424,17.459622874717,17.4756414594216,
17.4882250997439,17.5023107956712,17.5260684540758,17.6342620918617,17.7654974805742,
17.8365209489007,17.8510995376378,17.8593241227922,17.8657138629315,17.8747595927644,
17.8938100934201,17.9724594159901,18.1722338642068,18.2108072615323,18.2265118770991,
18.2382237784594,18.2511231586535,18.2692007711738,18.3144950827931,18.3807542873899,
18.4889661851832,18.6118628459642,18.6328859914446,18.6412077212122,18.647901962198,
18.6549114403332,18.6659943338251,18.7023633466317,18.7671353237329,18.9999060308964,
19.0318809578003,19.047665143945,19.0602248040117,19.0744536190217,19.0988787402169,
19.223344276648,19.3402849661336,19.4084121406566,19.42279793497,19.4309787255063,
19.4373752639112,19.4464838998575,19.4658693135521,19.5474830491216,19.5843922286228,
19.7569805605909,19.7845790192998,19.8009653554527,19.8136297031117,19.8273820175657,
19.8495890327939,19.9313998380183,20.106038918756,20.193591928415,20.2069032270294,
20.2151902137928,20.2217152871771,20.2295458143085,20.2444105787853,20.361350433356,
20.5655089110364,20.6012945033035,20.6176145467569,20.6302695062486,20.6440514222814,
20.666406735545,20.7516291900446,20.8565065700056,20.9694213497286,20.9905136728443,
20.9998340943112,21.0069385234827,21.0151491862314,21.0300681730316,21.1196154049678,
21.1748681507587,21.3261318313632,21.3581709385152,21.3739583841935,21.386517859895,
21.400744303133,21.425143854543,21.5416471411628,21.6785621967833,21.7649847628388,
21.7782658435484,21.7865436391079,21.7930680104112,21.8009055493004,21.8158047600009,
21.935410808731,22.1449971702972,22.1724889157877,22.1888602393926,22.2015222615868,
22.215279162764,22.2375203072286,22.3212395471551,22.5391114964196,22.560925794966,
22.5697953674184,22.576994920778,22.5846989944394,22.5972913076029,22.6436473705236,
22.7390977572285,22.8979241991219,22.929780157148,22.9455322610994,22.9580885575351,
22.9723380812627,22.9968448691232,23.1156962121063,23.261330431272,23.3360193182187,
23.3505702488122,23.3566815208642,23.3617662463869),.UNSPECIFIED.);
#30160=B_SPLINE_CURVE_WITH_KNOTS('',3,(#169411,#169412,#169413,#169414,
#169415,#169416,#169417,#169418,#169419,#169420,#169421,#169422,#169423,
#169424,#169425,#169426,#169427,#169428,#169429,#169430,#169431,#169432,
#169433,#169434,#169435,#169436,#169437,#169438,#169439,#169440,#169441,
#169442,#169443,#169444,#169445,#169446,#169447,#169448,#169449,#169450,
#169451,#169452,#169453,#169454,#169455,#169456,#169457,#169458,#169459,
#169460,#169461,#169462,#169463,#169464,#169465,#169466,#169467,#169468,
#169469,#169470,#169471,#169472,#169473,#169474,#169475,#169476,#169477,
#169478,#169479,#169480,#169481,#169482,#169483,#169484,#169485,#169486,
#169487,#169488,#169489,#169490,#169491,#169492,#169493,#169494,#169495,
#169496,#169497,#169498,#169499,#169500,#169501,#169502,#169503,#169504,
#169505,#169506,#169507,#169508,#169509,#169510,#169511,#169512,#169513,
#169514,#169515,#169516,#169517,#169518,#169519,#169520,#169521,#169522,
#169523,#169524,#169525,#169526,#169527,#169528,#169529,#169530,#169531,
#169532,#169533,#169534,#169535,#169536,#169537,#169538,#169539,#169540,
#169541,#169542,#169543,#169544,#169545,#169546,#169547,#169548,#169549,
#169550,#169551,#169552,#169553,#169554,#169555,#169556,#169557,#169558,
#169559,#169560,#169561,#169562,#169563,#169564,#169565,#169566,#169567,
#169568,#169569,#169570,#169571,#169572,#169573,#169574,#169575,#169576,
#169577,#169578,#169579,#169580,#169581,#169582,#169583,#169584,#169585,
#169586,#169587,#169588,#169589,#169590,#169591,#169592,#169593,#169594,
#169595,#169596,#169597,#169598,#169599,#169600,#169601,#169602,#169603,
#169604,#169605,#169606,#169607,#169608,#169609,#169610,#169611,#169612,
#169613,#169614,#169615,#169616,#169617,#169618,#169619,#169620,#169621,
#169622,#169623,#169624,#169625,#169626,#169627,#169628,#169629,#169630,
#169631,#169632,#169633,#169634,#169635,#169636,#169637,#169638,#169639,
#169640,#169641,#169642,#169643,#169644,#169645,#169646,#169647,#169648,
#169649,#169650,#169651,#169652,#169653,#169654,#169655,#169656,#169657,
#169658,#169659,#169660,#169661,#169662,#169663,#169664,#169665,#169666,
#169667,#169668,#169669,#169670),.UNSPECIFIED.,.F.,.F.,(4,2,2,2,2,2,2,2,
2,2,2,2,2,2,2,2,2,2,2,2,2,2,2,2,2,2,2,2,2,2,2,2,2,2,2,2,2,2,2,2,2,2,2,2,
2,2,2,2,2,2,2,2,2,2,2,2,2,2,2,2,2,2,2,2,2,2,2,2,2,2,2,2,2,2,2,2,2,2,2,2,
2,2,2,2,2,2,2,2,2,2,2,2,2,2,2,2,2,2,2,2,2,2,2,2,2,2,2,2,2,2,2,2,2,2,2,2,
2,2,2,2,2,2,2,2,2,2,2,2,2,4),(10.398744700606,10.4008561584502,10.4083978533202,
10.4215459790634,10.4778645782516,10.6496659209323,10.7641546126389,10.7884619920227,
10.8026701973569,10.8152349241933,10.8310575500151,10.8632705603044,11.0088451550061,
11.0685600676601,11.1590578976249,11.1740069389689,11.182224918033,11.1893295347377,
11.1986423962117,11.2196860193964,11.327127566098,11.4158727801605,11.4854634052821,
11.5308828072108,11.5494481126179,11.5623104951733,11.5754331156023,11.5946552612859,
11.6480146641304,11.7315857755624,11.9235202464166,11.952807537667,11.9633754704451,
11.9695883861885,11.9763187987357,11.986074391225,12.0118732800191,12.147869975836,
12.3201550382873,12.353828534035,12.3699385514725,12.3825334417738,12.3965691445339,
12.4200906361679,12.5236149349893,12.5892513133597,12.7216981890727,12.7420272310879,
12.7513541844365,12.7584605687789,12.7666698894368,12.7815779544907,12.8706802567874,
12.9156870915836,13.0788730815012,13.1098152906864,13.125595675421,13.1381566642025,
13.1523924342078,13.176827232678,13.2940113866893,13.4359751234392,13.4373849778119,
13.5170347572255,13.5301293116592,13.5383520503394,13.5448751221521,13.5527620192768,
13.5678942446418,13.7029026680166,13.8935507814303,13.9260940669884,13.9419891557434,
13.9545608964675,13.9687227709009,13.9928307458483,14.108782208555,14.2101541347645,
14.3013796617016,14.3166829553153,14.3250697110483,14.3321494089144,14.3413698938271,
14.3613520087862,14.4484221221795,14.5996623324507,14.6677741203912,14.6892948812208,
14.7028983303647,14.7156186369075,14.7326491796368,14.7714528188204,14.9085920463417,
15.0756709768052,15.0983213867863,15.1078750838088,15.1145012819586,15.1216269857896,
15.1332347905824,15.1748225824595,15.254629643548,15.4546686420783,15.4933965839387,
15.5091400695916,15.5208618855114,15.5337512176802,15.5517737548373,15.5968598132321,
15.6639151023815,15.75527402183,15.8641882624848,15.8852646694166,15.8945831053084,
15.9016881703043,15.9099021298115,15.9248331507426,16.0147265192899,16.0733653851664,
16.2207298875367,16.252893513232,16.2687063176727,16.2812697411125,16.2954833809431,
16.3198174413809,16.4348764186703,16.5931907105774,16.661136587772,16.6749536492156,
16.6826465666522,16.6851291404356),.UNSPECIFIED.);
#30161=B_SPLINE_CURVE_WITH_KNOTS('',3,(#169675,#169676,#169677,#169678,
#169679,#169680,#169681,#169682,#169683,#169684,#169685,#169686,#169687,
#169688,#169689,#169690,#169691,#169692,#169693,#169694,#169695,#169696,
#169697,#169698,#169699,#169700,#169701,#169702,#169703,#169704,#169705,
#169706,#169707,#169708,#169709,#169710,#169711,#169712,#169713,#169714,
#169715,#169716,#169717,#169718,#169719,#169720,#169721,#169722,#169723,
#169724,#169725,#169726,#169727,#169728,#169729,#169730,#169731,#169732,
#169733,#169734,#169735,#169736,#169737,#169738,#169739,#169740,#169741,
#169742,#169743,#169744,#169745,#169746,#169747,#169748,#169749,#169750,
#169751,#169752,#169753,#169754,#169755,#169756,#169757,#169758,#169759,
#169760,#169761,#169762,#169763,#169764,#169765,#169766,#169767,#169768,
#169769,#169770,#169771,#169772,#169773,#169774,#169775,#169776,#169777,
#169778,#169779,#169780,#169781,#169782,#169783,#169784,#169785,#169786,
#169787,#169788,#169789,#169790,#169791,#169792,#169793,#169794,#169795,
#169796,#169797,#169798,#169799,#169800,#169801,#169802,#169803,#169804,
#169805,#169806,#169807,#169808,#169809,#169810,#169811,#169812,#169813,
#169814,#169815,#169816,#169817,#169818,#169819,#169820,#169821,#169822,
#169823,#169824,#169825,#169826,#169827,#169828,#169829,#169830,#169831,
#169832,#169833,#169834,#169835,#169836,#169837,#169838,#169839,#169840,
#169841,#169842,#169843,#169844,#169845,#169846,#169847,#169848,#169849,
#169850,#169851,#169852,#169853,#169854,#169855,#169856,#169857,#169858,
#169859,#169860,#169861,#169862,#169863,#169864,#169865,#169866,#169867,
#169868,#169869,#169870,#169871,#169872,#169873,#169874,#169875,#169876,
#169877,#169878,#169879,#169880,#169881,#169882,#169883,#169884,#169885,
#169886,#169887,#169888,#169889,#169890,#169891,#169892,#169893,#169894,
#169895,#169896,#169897,#169898,#169899,#169900,#169901,#169902,#169903,
#169904,#169905,#169906,#169907,#169908,#169909,#169910,#169911,#169912,
#169913,#169914,#169915,#169916,#169917,#169918,#169919,#169920,#169921,
#169922,#169923,#169924,#169925,#169926,#169927,#169928,#169929,#169930,
#169931,#169932),.UNSPECIFIED.,.F.,.F.,(4,2,2,2,2,2,2,2,2,2,2,2,2,2,2,2,
2,2,2,2,2,2,2,2,2,2,2,2,2,2,2,2,2,2,2,2,2,2,2,2,2,2,2,2,2,2,2,2,2,2,2,2,
2,2,2,2,2,2,2,2,2,2,2,2,2,2,2,2,2,2,2,2,2,2,2,2,2,2,2,2,2,2,2,2,2,2,2,2,
2,2,2,2,2,2,2,2,2,2,2,2,2,2,2,2,2,2,2,2,2,2,2,2,2,2,2,2,2,2,2,2,2,2,2,2,
2,2,2,2,4),(10.7898186351041,10.7921918032135,10.7998388212371,10.81345228456,
10.8774594094187,11.0730362515152,11.1297095366792,11.1700874911333,11.1873832545396,
11.2001457554164,11.212029370956,11.2316498044645,11.2839383106706,11.4490478245626,
11.5412621511017,11.5617799221726,11.5710981300933,11.5781225898265,11.5864135061441,
11.6012871678741,11.6806489981361,11.8469704721643,11.9155152772257,11.9370845669454,
11.9506979558565,11.9634133058162,11.9804155693687,12.0190575894802,12.1584082443195,
12.329256882272,12.3481323806516,12.356791095682,12.3633655219846,12.3708426765423,
12.3840494355145,12.447782440295,12.5678857268475,12.7240782105056,12.7495763548337,
12.7641899982491,12.776595107701,12.791806092072,12.8209212843122,12.923312511244,
13.0847249400031,13.1260740585857,13.1386353954765,13.1463332793623,13.1536224450291,
13.1642608951442,13.1930339260669,13.2384968635326,13.3428181055496,13.4806114046105,
13.5052647290925,13.5196842057074,13.5322234380873,13.5477364300346,13.5783227669092,
13.6889965649581,13.836999880382,13.9085375802838,13.9225654133134,13.9303055077478,
13.9368386191739,13.9452430332507,13.9629770823624,14.0929601954303,14.2846050717009,
14.3170628758517,14.3329410859518,14.3455106299147,14.3596818144301,14.3838350793634,
14.5009185353507,14.6114904867803,14.6766888519298,14.7020986700663,14.7125218106092,
14.7196989835066,14.7274475075633,14.7402394020425,14.7889374272439,14.8932704507135,
14.9027599775658,15.0399758877475,15.0721676908585,15.0879855904972,15.1005491202281,
15.1147586884187,15.1390752337641,15.2537823369036,15.4198558817108,15.4810594717459,
15.4945173671567,15.5021291215348,15.5086158320848,15.5171670899168,15.5356813053504,
15.6137538003989,15.7923997336184,15.8725197194364,15.8953818904609,15.909276893723,
15.9219020955858,15.9382735080365,15.9734247060353,16.0211412591509,16.1631561245004,
16.2189479944778,16.2677062901924,16.2809645850439,16.2888156350195,16.2960271150681,
16.3062395469988,16.3321140375229,16.4801830654789,16.6236315158137,16.6482764948441,
16.6626938420286,16.6752328748452,16.6907477502608,16.7213449429958,16.8321021951556,
16.9793319257277,17.0514845874532,17.0655384951259,17.0732842839512,17.0758907305399),
 .UNSPECIFIED.);
#30162=B_SPLINE_CURVE_WITH_KNOTS('',3,(#169933,#169934,#169935,#169936,
#169937,#169938,#169939,#169940,#169941,#169942,#169943,#169944,#169945,
#169946,#169947,#169948,#169949,#169950,#169951,#169952,#169953,#169954,
#169955,#169956,#169957,#169958,#169959,#169960,#169961,#169962,#169963,
#169964,#169965,#169966,#169967,#169968,#169969,#169970,#169971,#169972,
#169973,#169974,#169975,#169976,#169977,#169978,#169979,#169980,#169981,
#169982,#169983,#169984,#169985,#169986,#169987,#169988,#169989,#169990,
#169991,#169992,#169993,#169994,#169995,#169996,#169997,#169998,#169999,
#170000,#170001,#170002,#170003,#170004,#170005,#170006,#170007,#170008,
#170009,#170010,#170011,#170012,#170013,#170014,#170015,#170016,#170017,
#170018,#170019,#170020,#170021,#170022,#170023,#170024,#170025,#170026,
#170027,#170028,#170029,#170030,#170031,#170032,#170033,#170034,#170035,
#170036,#170037,#170038,#170039,#170040,#170041,#170042,#170043,#170044,
#170045,#170046,#170047,#170048,#170049,#170050,#170051,#170052,#170053,
#170054,#170055,#170056,#170057,#170058,#170059,#170060,#170061,#170062,
#170063,#170064,#170065,#170066,#170067,#170068,#170069,#170070,#170071,
#170072,#170073,#170074,#170075,#170076,#170077,#170078,#170079,#170080,
#170081,#170082,#170083,#170084,#170085,#170086,#170087,#170088,#170089,
#170090,#170091,#170092,#170093,#170094,#170095,#170096,#170097,#170098,
#170099,#170100,#170101,#170102,#170103,#170104,#170105,#170106,#170107,
#170108,#170109,#170110,#170111,#170112,#170113,#170114,#170115,#170116,
#170117,#170118,#170119,#170120,#170121,#170122,#170123,#170124,#170125,
#170126,#170127,#170128,#170129,#170130,#170131,#170132,#170133,#170134,
#170135,#170136,#170137,#170138,#170139,#170140,#170141,#170142,#170143,
#170144,#170145,#170146,#170147,#170148,#170149,#170150,#170151,#170152,
#170153,#170154,#170155,#170156,#170157,#170158,#170159,#170160,#170161,
#170162,#170163,#170164,#170165,#170166,#170167,#170168,#170169,#170170,
#170171,#170172,#170173,#170174,#170175,#170176,#170177,#170178,#170179,
#170180,#170181,#170182,#170183,#170184,#170185,#170186,#170187,#170188),
 .UNSPECIFIED.,.F.,.F.,(4,2,2,2,2,2,2,2,2,2,2,2,2,2,2,2,2,2,2,2,2,2,2,2,
2,2,2,2,2,2,2,2,2,2,2,2,2,2,2,2,2,2,2,2,2,2,2,2,2,2,2,2,2,2,2,2,2,2,2,2,
2,2,2,2,2,2,2,2,2,2,2,2,2,2,2,2,2,2,2,2,2,2,2,2,2,2,2,2,2,2,2,2,2,2,2,2,
2,2,2,2,2,2,2,2,2,2,2,2,2,2,2,2,2,2,2,2,2,2,2,2,2,2,2,2,2,2,2,4),(16.6851291404356,
16.6891848353774,16.6976541060233,16.7157297009885,16.7900676343414,16.9900542918037,
17.056157653,17.0775654245892,17.0911462205749,17.1038750923964,17.1209649827791,
17.1602148900421,17.2155519530881,17.3153895467823,17.4358812228311,17.4568460367297,
17.4661446911833,17.4732473216251,17.4814735682872,17.496462703809,17.5883925759467,
17.6345856849508,17.7924757253217,17.8245046154945,17.8402912599175,17.8528520126454,
17.8670819451238,17.8914926423306,18.0081858277598,18.1534869576225,18.2317990716855,
18.2448506723089,18.253060198381,18.2595823246727,18.2674796199095,18.2826637129226,
18.4205221558987,18.6077739697828,18.6405916646402,18.6565385726394,18.6691147560217,
18.6832432446556,18.7071991515676,18.8196430282876,18.972893324294,19.0202446257863,
19.0333793978062,19.0412032996922,19.0484266834284,19.0587079185179,19.0850340229593,
19.2335282765803,19.3759126711263,19.4005697015907,19.4149897167684,19.427528439784,
19.4430395413321,19.473617927943,19.5842368592339,19.732684080907,19.8038603693889,
19.81787226502,19.8256086440089,19.8321418802572,19.8405506491336,19.8583084044284,
19.9653030926738,20.1544009353061,20.2038026128688,20.2230463201509,20.2348594163614,
20.2476692402974,20.2652494181708,20.3074917502285,20.3687021764774,20.4668259401795,
20.5787090711882,20.5997997406627,20.6091203243637,20.6162252571657,20.6244369547715,
20.6393588895596,20.7289719790186,20.7850143526512,20.9356988003089,20.9675777789258,
20.9833351182327,20.9958927941399,21.0101408919735,21.0346376318975,21.153229725294,
21.3107695392435,21.3758874242494,21.3895594649733,21.3972194484067,21.403761318284,
21.4122763457042,21.4305972497696,21.5070129869486,21.6834220473702,21.7670890648905,
21.7902759958697,21.8042410602935,21.8168489584327,21.8330837738811,21.8674914735401,
21.9138749148698,22.0321362705211,22.1501942121107,22.1712311239756,22.1805422020978,
22.1876459674459,22.1958635653018,22.2108133481679,22.3013794266412,22.3608920329085,
22.506580892971,22.5387878367801,22.5546082666932,22.5671715977257,22.5813785937464,
22.6056848362693,22.7201936103805,22.8619754129453,22.9442317078442,22.9594782998301,
22.9657894059735,22.970999517308),.UNSPECIFIED.);
#30163=B_SPLINE_CURVE_WITH_KNOTS('',3,(#170193,#170194,#170195,#170196,
#170197,#170198,#170199,#170200,#170201,#170202,#170203,#170204,#170205,
#170206,#170207,#170208,#170209,#170210,#170211,#170212,#170213,#170214,
#170215,#170216,#170217,#170218,#170219,#170220,#170221,#170222,#170223,
#170224,#170225,#170226,#170227,#170228,#170229,#170230,#170231,#170232,
#170233,#170234,#170235,#170236,#170237,#170238,#170239,#170240,#170241,
#170242,#170243,#170244,#170245,#170246,#170247,#170248,#170249,#170250,
#170251,#170252,#170253,#170254,#170255,#170256,#170257,#170258,#170259,
#170260,#170261,#170262,#170263,#170264,#170265,#170266,#170267,#170268,
#170269,#170270,#170271,#170272,#170273,#170274,#170275,#170276,#170277,
#170278,#170279,#170280,#170281,#170282,#170283,#170284,#170285,#170286,
#170287,#170288,#170289,#170290,#170291,#170292,#170293,#170294,#170295,
#170296,#170297,#170298,#170299,#170300,#170301,#170302,#170303,#170304,
#170305,#170306,#170307,#170308,#170309,#170310,#170311,#170312,#170313,
#170314,#170315,#170316,#170317,#170318,#170319,#170320,#170321,#170322,
#170323,#170324,#170325,#170326,#170327,#170328,#170329,#170330,#170331,
#170332,#170333,#170334,#170335,#170336,#170337,#170338,#170339,#170340,
#170341,#170342,#170343,#170344,#170345,#170346,#170347,#170348,#170349,
#170350,#170351,#170352,#170353,#170354,#170355,#170356,#170357,#170358,
#170359,#170360,#170361,#170362,#170363,#170364,#170365,#170366,#170367,
#170368,#170369,#170370,#170371,#170372,#170373,#170374,#170375,#170376,
#170377,#170378,#170379,#170380,#170381,#170382,#170383,#170384,#170385,
#170386,#170387,#170388,#170389,#170390,#170391,#170392,#170393,#170394,
#170395,#170396,#170397,#170398,#170399,#170400,#170401,#170402,#170403,
#170404,#170405,#170406,#170407,#170408,#170409,#170410,#170411,#170412,
#170413,#170414,#170415,#170416,#170417,#170418,#170419,#170420,#170421,
#170422,#170423,#170424,#170425,#170426,#170427,#170428,#170429,#170430,
#170431,#170432,#170433,#170434,#170435,#170436,#170437,#170438,#170439,
#170440,#170441,#170442,#170443,#170444,#170445,#170446,#170447,#170448,
#170449,#170450,#170451,#170452,#170453,#170454),.UNSPECIFIED.,.F.,.F.,
(4,2,2,2,2,2,2,2,2,2,2,2,2,2,2,2,2,2,2,2,2,2,2,2,2,2,2,2,2,2,2,2,2,2,2,
2,2,2,2,2,2,2,2,2,2,2,2,2,2,2,2,2,2,2,2,2,2,2,2,2,2,2,2,2,2,2,2,2,2,2,2,
2,2,2,2,2,2,2,2,2,2,2,2,2,2,2,2,2,2,2,2,2,2,2,2,2,2,2,2,2,2,2,2,2,2,2,2,
2,2,2,2,2,2,2,2,2,2,2,2,2,2,2,2,2,2,2,2,2,2,2,4),(4.50400203993545,4.50783078879762,
4.51617336957014,4.52967085577925,4.645661358127,4.66484391224903,4.77745340529264,
4.83969458000058,4.88296902407783,4.90073353901219,4.91357602962783,4.92535018303914,
4.94131179144098,4.98143819914888,5.17618136231952,5.23614973539588,5.27093510019915,
5.2823494982435,5.2897967772644,5.29639604111083,5.30547187381965,5.32850840604712,
5.47934159114501,5.60233834905262,5.64028225564697,5.6571486018372,5.66984239122988,
5.68351052058056,5.70532610630803,5.77509730238163,5.94562219603879,6.05030002355518,
6.06495719017102,6.07274448292501,6.07927301024529,6.08761480270507,6.10110926187093,
6.19816676464921,6.32365119136852,6.44056041220587,6.46498059683818,6.47921227426936,
6.4917722981847,6.50755500072208,6.5395651185537,6.69182664965174,6.74620444512316,
6.83569768772053,6.85061606014671,6.85882703442838,6.86593216358815,6.87525405511605,
6.89635192810502,7.01005492593952,7.13548735728464,7.18032138194295,7.21385502669898,
7.22992740954191,7.24251670474267,7.25657182177177,7.28017407340108,7.36995511210761,
7.54036075213862,7.61599982243425,7.63422947861459,7.6427274651935,7.64926788325522,
7.65693982831498,7.67066474042213,7.73679428780625,7.89388882437003,8.01188767967951,
8.03635792186589,8.05060041377246,8.06315900594515,8.07892529048758,8.11085007986573,
8.26434403883236,8.31769085454703,8.4071230587894,8.42203966058159,8.43025027784888,
8.43735551002728,8.44667806092502,8.46777955236474,8.58210897290625,8.68624202648577,
8.77090635592798,8.79322136798927,8.80699539494234,8.81965430041978,8.83599510682316,
8.86337577700412,9.07391539198163,9.19282037175703,9.20771235395789,9.21554900316822,
9.22207434434218,9.23035554118649,9.2436461332262,9.33104565818227,9.33430254033697,
9.46662507022681,9.58349671221414,9.6079159795697,9.62214784846763,9.63470847622948,
9.65049251760594,9.6825074199498,9.83408467373633,9.8891052812609,9.97864442223905,
9.99356469161716,10.0017762878928,10.0088816737712,10.0182035439249,10.03929991615,
10.152482068856,10.2783117601934,10.3232211169318,10.3567978592978,10.3728787422926,
10.3854694458644,10.3995207130716,10.4231033872177,10.5125759737873,10.6832927165416,
10.7589755972446,10.7772108283276,10.7857100808537,10.7898186351041),
 .UNSPECIFIED.);
#30164=B_SPLINE_CURVE_WITH_KNOTS('',3,(#170455,#170456,#170457,#170458,
#170459,#170460,#170461,#170462,#170463,#170464,#170465,#170466,#170467,
#170468,#170469,#170470,#170471,#170472,#170473,#170474,#170475,#170476,
#170477,#170478,#170479,#170480,#170481,#170482,#170483,#170484,#170485,
#170486,#170487,#170488,#170489,#170490,#170491,#170492,#170493,#170494,
#170495,#170496,#170497,#170498,#170499,#170500,#170501,#170502,#170503,
#170504,#170505,#170506,#170507,#170508,#170509,#170510,#170511,#170512,
#170513,#170514,#170515,#170516,#170517,#170518,#170519,#170520,#170521,
#170522,#170523,#170524,#170525,#170526,#170527,#170528,#170529,#170530,
#170531,#170532,#170533,#170534,#170535,#170536,#170537,#170538,#170539,
#170540,#170541,#170542,#170543,#170544,#170545,#170546,#170547,#170548,
#170549,#170550,#170551,#170552,#170553,#170554,#170555,#170556,#170557,
#170558,#170559,#170560,#170561,#170562,#170563,#170564,#170565,#170566,
#170567,#170568,#170569,#170570,#170571,#170572,#170573,#170574,#170575,
#170576,#170577,#170578,#170579,#170580,#170581,#170582,#170583,#170584,
#170585,#170586,#170587,#170588,#170589,#170590,#170591,#170592,#170593,
#170594,#170595,#170596,#170597,#170598,#170599,#170600,#170601,#170602,
#170603,#170604,#170605,#170606,#170607,#170608,#170609,#170610,#170611,
#170612,#170613,#170614,#170615,#170616,#170617,#170618,#170619,#170620,
#170621,#170622,#170623,#170624,#170625,#170626,#170627,#170628,#170629,
#170630,#170631,#170632,#170633,#170634,#170635,#170636,#170637,#170638,
#170639,#170640,#170641,#170642,#170643,#170644,#170645,#170646,#170647,
#170648,#170649,#170650,#170651,#170652,#170653,#170654,#170655,#170656,
#170657,#170658,#170659,#170660,#170661,#170662,#170663,#170664,#170665,
#170666,#170667,#170668,#170669,#170670,#170671,#170672,#170673,#170674,
#170675,#170676,#170677,#170678,#170679,#170680,#170681,#170682,#170683,
#170684,#170685,#170686,#170687,#170688,#170689,#170690,#170691,#170692,
#170693,#170694,#170695,#170696,#170697,#170698,#170699,#170700,#170701,
#170702,#170703,#170704,#170705,#170706,#170707,#170708,#170709,#170710,
#170711,#170712,#170713,#170714),.UNSPECIFIED.,.F.,.F.,(4,2,2,2,2,2,2,2,
2,2,2,2,2,2,2,2,2,2,2,2,2,2,2,2,2,2,2,2,2,2,2,2,2,2,2,2,2,2,2,2,2,2,2,2,
2,2,2,2,2,2,2,2,2,2,2,2,2,2,2,2,2,2,2,2,2,2,2,2,2,2,2,2,2,2,2,2,2,2,2,2,
2,2,2,2,2,2,2,2,2,2,2,2,2,2,2,2,2,2,2,2,2,2,2,2,2,2,2,2,2,2,2,2,2,2,2,2,
2,2,2,2,2,2,2,2,2,2,2,2,2,4),(9.99999999314102E-7,0.00521187694995086,0.0115243780586715,
0.0267764289715423,0.109101741016729,0.250843391215176,0.365307860432174,
0.389610755024793,0.403816410484198,0.416378925485257,0.432198823705125,
0.464406488465193,0.609941514961661,0.669861994045137,0.760150764001163,
0.775091551278359,0.783306881601369,0.790410465265545,0.799723570901651,
0.820774205379463,0.935181085531112,1.05604958818247,1.1029796647841,1.13769227386817,
1.15398250233226,1.16659640651649,1.18053067832399,1.20357838282418,1.2855080131829,
1.46234388816903,1.54006507023998,1.55853763968509,1.56708060882173,1.57356588606699,
1.5811817213839,1.59465978182557,1.65623642278592,1.82186528698761,1.93658062216615,
1.9608956522277,1.97510393887553,1.98766609565137,2.00348194636585,2.03566844989071,
2.17227750047059,2.31077637813875,2.33978744715114,2.35045844852665,2.35775323319897,
2.36543933592666,2.37794986739516,2.41882190395879,2.45513570201323,2.5920602532835,
2.69320597781548,2.71659414321804,2.73059928129607,2.74319738742964,2.75935406837429,
2.79328673569503,2.96175212978104,3.01795359068554,3.11761975813416,3.13216655731193,
3.13993029434479,3.14646027338732,3.15483108021548,3.1684242830127,3.27159172098514,
3.39073081656475,3.50766257455933,3.53208242695173,3.54631338335822,3.55887245508663,
3.57465353985711,3.60665887413866,3.76464241422557,3.86054773413309,3.89180580933521,
3.91371783832301,3.92328279764401,3.93039703745322,3.938558985752,3.95286180535382,
4.01904292745739,4.16220513375268,4.23014815079747,4.27565233493159,4.29373623108368,
4.3066354453395,4.3198978121195,4.33980939688194,4.39373370619213,4.57844285303776,
4.68387023636065,4.70156430183261,4.70996049778992,4.71649232258913,4.72423694408111,
4.73828744444111,4.81038147503658,4.95767073515514,5.06841665922256,5.09901083576851,
5.11452427933853,5.12706219853634,5.14147831364645,5.16612130980634,5.30330060422524,
5.40494466480211,5.47538811634404,5.48956928721446,5.49762129629522,5.50476222644121,
5.51452917883596,5.53762667411542,5.5711815501957,5.68048559906794,5.82074929137883,
5.85296115228007,5.86878205667884,5.88134489166568,5.8955503991264,5.91985176371621,
6.03427857298967,6.20680983655509,6.26247544082628,6.27557884477625,6.28310963195874,
6.28519602509786),.UNSPECIFIED.);
#30165=B_SPLINE_CURVE_WITH_KNOTS('',3,(#170720,#170721,#170722,#170723,
#170724,#170725,#170726,#170727,#170728,#170729,#170730,#170731,#170732,
#170733,#170734,#170735,#170736,#170737,#170738,#170739,#170740,#170741,
#170742,#170743,#170744,#170745,#170746,#170747,#170748,#170749,#170750,
#170751,#170752,#170753,#170754,#170755,#170756,#170757,#170758,#170759,
#170760,#170761,#170762,#170763,#170764,#170765,#170766,#170767,#170768,
#170769,#170770,#170771,#170772,#170773,#170774,#170775,#170776,#170777,
#170778,#170779,#170780,#170781,#170782,#170783,#170784,#170785,#170786,
#170787,#170788,#170789,#170790,#170791,#170792,#170793,#170794,#170795,
#170796,#170797,#170798,#170799,#170800,#170801,#170802,#170803,#170804,
#170805,#170806,#170807,#170808,#170809,#170810,#170811,#170812,#170813,
#170814,#170815,#170816,#170817,#170818,#170819,#170820,#170821,#170822,
#170823,#170824,#170825,#170826,#170827,#170828,#170829,#170830,#170831,
#170832,#170833,#170834,#170835,#170836,#170837,#170838,#170839,#170840,
#170841,#170842,#170843,#170844,#170845,#170846,#170847,#170848,#170849,
#170850,#170851,#170852,#170853,#170854,#170855,#170856,#170857,#170858,
#170859,#170860,#170861,#170862,#170863,#170864,#170865,#170866,#170867,
#170868,#170869,#170870,#170871,#170872,#170873),.UNSPECIFIED.,.F.,.F.,
(4,2,2,2,2,2,2,2,2,2,2,2,2,2,2,2,2,2,2,2,2,2,2,2,2,2,2,2,2,2,2,2,2,2,2,
2,2,2,2,2,2,2,2,2,2,2,2,2,2,2,2,2,2,2,2,2,2,2,2,2,2,2,2,2,2,2,2,2,2,2,2,
2,2,2,2,2,4),(6.44324130749359,6.45009989945945,6.46952174069895,6.51371948633358,
6.58264731915039,6.78450170032278,6.83051898716609,6.86078018873499,6.8909498277508,
6.93660137164695,6.99185200670286,7.12821205945386,7.21188928495002,7.23668756456504,
7.25341893997957,7.27328405056241,7.31537886060976,7.44333783601869,7.57348204528162,
7.61342556797451,7.64267743466213,7.67449810850209,7.72894478014473,7.8378171049123,
7.98611714158222,8.02850948778931,8.04763977263604,8.06135457370724,8.08107703485136,
8.12721051481373,8.20091774318204,8.4031357171896,8.44549529415767,8.47482898268042,
8.50573768590399,8.55550330556311,8.58880282586661,8.69495127610468,8.81377919504479,
8.84302264517212,8.86049944932598,8.8787284981319,8.91179996796876,8.95645174496428,
9.09585729472496,9.18897227904853,9.22661307320286,9.25566055395916,9.28823312004371,
9.34679551122857,9.42440073750344,9.52759101876076,9.62646011006886,9.65106087315707,
9.66667331032369,9.68373228491427,9.71477075757884,9.75606528653478,9.87174019916766,
10.0039500133767,10.0508708182577,10.0812947528742,10.1113136944997,10.1561082457514,
10.2825312016657,10.4279124024802,10.4552930886508,10.4707408756368,10.4888420793433,
10.5212606070798,10.6089376933129,10.7915881430545,10.832893936256,10.8623412354449,
10.8892975116174,10.9193612832434,10.9565256385629),.UNSPECIFIED.);
#30166=B_SPLINE_CURVE_WITH_KNOTS('',3,(#170876,#170877,#170878,#170879,
#170880,#170881,#170882,#170883,#170884,#170885,#170886,#170887,#170888,
#170889,#170890,#170891,#170892,#170893,#170894,#170895,#170896,#170897,
#170898,#170899,#170900,#170901,#170902,#170903,#170904,#170905,#170906,
#170907,#170908,#170909,#170910,#170911,#170912,#170913,#170914,#170915,
#170916,#170917,#170918,#170919,#170920,#170921,#170922,#170923,#170924,
#170925,#170926,#170927,#170928,#170929,#170930,#170931,#170932,#170933,
#170934,#170935,#170936,#170937,#170938,#170939,#170940,#170941,#170942,
#170943,#170944,#170945,#170946,#170947,#170948,#170949,#170950,#170951,
#170952,#170953,#170954,#170955,#170956,#170957,#170958,#170959,#170960,
#170961,#170962,#170963,#170964,#170965,#170966,#170967,#170968,#170969,
#170970,#170971,#170972,#170973,#170974,#170975,#170976,#170977,#170978,
#170979,#170980,#170981,#170982,#170983,#170984,#170985,#170986,#170987,
#170988,#170989,#170990,#170991,#170992,#170993,#170994,#170995,#170996,
#170997,#170998,#170999,#171000,#171001,#171002,#171003,#171004,#171005,
#171006,#171007,#171008,#171009,#171010,#171011,#171012,#171013),
 .UNSPECIFIED.,.F.,.F.,(4,2,2,2,2,2,2,2,2,2,2,2,2,2,2,2,2,2,2,2,2,2,2,2,
2,2,2,2,2,2,2,2,2,2,2,2,2,2,2,2,2,2,2,2,2,2,2,2,2,2,2,2,2,2,2,2,2,2,2,2,
2,2,2,2,2,2,2,2,4),(9.99999999894808E-7,0.0130525840280033,0.0250471003602153,
0.0423664309872074,0.0710432677210413,0.192633457570409,0.34076010321594,
0.384889710270354,0.414795624627185,0.445362477788186,0.493057746807944,
0.643693335011998,0.744750679568014,0.800416149366004,0.821461677838465,
0.83672923651018,0.855615531649739,0.896541970431237,1.04634851009296,1.16347119594112,
1.21379636485514,1.24485044205548,1.27410460991681,1.30938174994106,1.41967247131201,
1.54331898859052,1.58575137558574,1.61764879222985,1.63564784065184,1.65115457186324,
1.67889521792463,1.84512752293783,1.92455612337491,1.95224397680292,1.99600296939021,
2.02584569639317,2.0528694479377,2.09755771731233,2.30039509475668,2.37043808010399,
2.41509540238138,2.43458941151924,2.44981412633709,2.4697518945745,2.51413855687589,
2.76157189397774,2.81903983964568,2.85141405184491,2.88050549044656,2.91852224989909,
3.01334438430698,3.15056968303968,3.19493301374123,3.22785352038779,3.24605297969566,
3.26355178142859,3.29291102618676,3.45045501550115,3.53302930270614,3.59299173898179,
3.62572446262663,3.65474162204956,3.69206239054126,3.78016692247768,3.80006553634604,
3.95104662110329,4.01888554269364,4.04128254128481,4.05239777510564),
 .UNSPECIFIED.);
#30167=B_SPLINE_CURVE_WITH_KNOTS('',3,(#171018,#171019,#171020,#171021,
#171022,#171023,#171024,#171025,#171026,#171027,#171028,#171029,#171030,
#171031,#171032,#171033,#171034,#171035,#171036,#171037,#171038,#171039,
#171040,#171041,#171042,#171043,#171044,#171045,#171046,#171047,#171048,
#171049,#171050,#171051,#171052,#171053,#171054,#171055,#171056,#171057,
#171058,#171059,#171060,#171061,#171062,#171063,#171064,#171065,#171066,
#171067,#171068,#171069,#171070,#171071,#171072,#171073,#171074,#171075,
#171076,#171077,#171078,#171079,#171080,#171081,#171082,#171083,#171084,
#171085,#171086,#171087,#171088,#171089,#171090,#171091,#171092,#171093,
#171094,#171095,#171096,#171097,#171098,#171099,#171100,#171101,#171102,
#171103,#171104,#171105,#171106,#171107,#171108,#171109,#171110,#171111,
#171112,#171113,#171114,#171115,#171116,#171117,#171118,#171119,#171120,
#171121,#171122,#171123,#171124,#171125,#171126,#171127,#171128,#171129,
#171130,#171131,#171132,#171133,#171134,#171135,#171136,#171137,#171138,
#171139,#171140,#171141,#171142,#171143,#171144,#171145,#171146,#171147,
#171148,#171149,#171150,#171151,#171152,#171153,#171154,#171155,#171156,
#171157,#171158,#171159,#171160,#171161,#171162,#171163,#171164,#171165,
#171166,#171167,#171168,#171169,#171170,#171171,#171172,#171173,#171174,
#171175,#171176,#171177,#171178,#171179,#171180,#171181,#171182,#171183,
#171184,#171185,#171186,#171187,#171188,#171189,#171190,#171191,#171192,
#171193,#171194,#171195,#171196,#171197,#171198,#171199,#171200,#171201,
#171202,#171203,#171204,#171205,#171206,#171207,#171208,#171209,#171210,
#171211,#171212,#171213,#171214,#171215,#171216,#171217,#171218,#171219,
#171220,#171221,#171222,#171223,#171224,#171225,#171226,#171227,#171228,
#171229,#171230,#171231),.UNSPECIFIED.,.F.,.F.,(4,2,2,2,2,2,2,2,2,2,2,2,
2,2,2,2,2,2,2,2,2,2,2,2,2,2,2,2,2,2,2,2,2,2,2,2,2,2,2,2,2,2,2,2,2,2,2,2,
2,2,2,2,2,2,2,2,2,2,2,2,2,2,2,2,2,2,2,2,2,2,2,2,2,2,2,2,2,2,2,2,2,2,2,2,
2,2,2,2,2,2,2,2,2,2,2,2,2,2,2,2,2,2,2,2,2,2,4),(1.00000000121357E-6,0.0132985295892812,
0.0305000676118254,0.0775692256728027,0.240329177579876,0.317940181801879,
0.376505573386614,0.409079332936633,0.438127542992531,0.475768834166774,
0.568885314201447,0.708281105687855,0.752931035956093,0.786002062687976,
0.804231354419126,0.821708779458675,0.850954001770212,0.969779811205238,
1.07594614121046,1.10924966352201,1.15901958569497,1.18992963621842,1.219263685806,
1.26162217598733,1.46383810972887,1.53753889267239,1.56989739314913,1.5958354235727,
1.61185803830954,1.62857798714354,1.65793469577569,1.82894800314684,1.93570299071125,
1.99023923088798,2.02207672419668,2.05132329240569,2.09122617743967,2.21166682806551,
2.32613966015929,2.36711268145982,2.39822254302645,2.41606553077769,2.4316703550286,
2.45999901482697,2.59492100741736,2.7349024933847,2.77744414123908,2.80708613984153,
2.83804419215404,2.88785350445539,3.08662018715367,3.15275155788358,3.19577430269898,
3.21500758194648,3.2302454924629,3.25047873061391,3.29661415563424,3.5422014322881,
3.59928708186249,3.631591986514,3.66070082358628,3.69885666652083,3.79747243719323,
3.93139357911008,3.97531070010754,4.00799669647732,4.02615048001158,4.04368532504206,
4.07323084518633,4.17822468056961,4.29310811558839,4.32796978894856,4.37932841061905,
4.41052714031691,4.43970790316327,4.48109097958902,4.62179856396732,4.74007571658718,
4.78181922664451,4.81310234910538,4.83021039824333,4.84579753539331,4.87025488503379,
4.96231649282271,5.11014528919533,5.16899375117321,5.21725337041476,5.24792388189464,
5.27740809051997,5.32078858951301,5.47828530244555,5.59181491813238,5.62120983726276,
5.63871586987435,5.65690714073263,5.68978405857206,5.73406431524519,5.87065192694529,
5.96620333617338,6.00425804766391,6.03335479769658,6.06571117634368,6.12307795036316,
6.3700061840772,6.41485391950567,6.43487189935052,6.44324130749359),
 .UNSPECIFIED.);
#30168=B_SPLINE_CURVE_WITH_KNOTS('',3,(#171232,#171233,#171234,#171235,
#171236,#171237,#171238,#171239,#171240,#171241,#171242,#171243,#171244,
#171245,#171246,#171247,#171248,#171249,#171250,#171251,#171252,#171253,
#171254,#171255,#171256,#171257,#171258,#171259,#171260,#171261,#171262,
#171263,#171264,#171265,#171266,#171267,#171268,#171269,#171270,#171271,
#171272,#171273,#171274,#171275,#171276,#171277,#171278,#171279,#171280,
#171281,#171282,#171283,#171284,#171285,#171286,#171287,#171288,#171289,
#171290,#171291,#171292,#171293,#171294,#171295,#171296,#171297,#171298,
#171299,#171300,#171301,#171302,#171303,#171304,#171305,#171306,#171307,
#171308,#171309,#171310,#171311,#171312,#171313,#171314,#171315,#171316,
#171317,#171318,#171319,#171320,#171321,#171322,#171323,#171324,#171325,
#171326,#171327,#171328,#171329,#171330,#171331,#171332,#171333,#171334,
#171335,#171336,#171337,#171338,#171339,#171340,#171341,#171342,#171343,
#171344,#171345,#171346,#171347,#171348,#171349,#171350,#171351,#171352,
#171353,#171354,#171355,#171356,#171357,#171358,#171359,#171360,#171361,
#171362,#171363,#171364,#171365,#171366,#171367,#171368,#171369,#171370,
#171371,#171372,#171373,#171374,#171375,#171376,#171377,#171378,#171379,
#171380,#171381,#171382,#171383,#171384,#171385,#171386,#171387,#171388,
#171389,#171390,#171391,#171392,#171393,#171394,#171395,#171396,#171397,
#171398,#171399,#171400,#171401,#171402,#171403,#171404,#171405,#171406,
#171407,#171408,#171409,#171410,#171411,#171412,#171413,#171414,#171415,
#171416,#171417,#171418,#171419,#171420,#171421,#171422,#171423,#171424,
#171425,#171426,#171427,#171428,#171429,#171430,#171431,#171432,#171433,
#171434,#171435,#171436,#171437,#171438,#171439,#171440,#171441,#171442,
#171443),.UNSPECIFIED.,.F.,.F.,(4,2,2,2,2,2,2,2,2,2,2,2,2,2,2,2,2,2,2,2,
2,2,2,2,2,2,2,2,2,2,2,2,2,2,2,2,2,2,2,2,2,2,2,2,2,2,2,2,2,2,2,2,2,2,2,2,
2,2,2,2,2,2,2,2,2,2,2,2,2,2,2,2,2,2,2,2,2,2,2,2,2,2,2,2,2,2,2,2,2,2,2,2,
2,2,2,2,2,2,2,2,2,2,2,2,2,4),(4.05239777510564,4.05669631670699,4.07474633851778,
4.11093866250766,4.26584683425855,4.37831229643335,4.43228498905449,4.46401679397778,
4.49329763725746,4.53346068528141,4.72136923542866,4.7887627863517,4.83240337843136,
4.85252224128053,4.86919630816024,4.89353311098095,4.97224055757222,5.11298425432336,
5.16895743666786,5.21503078211746,5.24527378241042,5.27545830392223,5.32105479858966,
5.49217779118691,5.62009465225304,5.64716561778583,5.66341526327337,5.67985805846434,
5.70786619889621,5.85628026117951,5.99387218746446,6.04520914801298,6.07645108367382,
6.10593901988633,6.14750875484144,6.32568276461725,6.39712219394073,6.44239362779474,
6.46277280506414,6.47940028866236,6.50330774927925,6.57565196846024,6.68032886790893,
6.77136600383769,6.82166771010724,6.85267401853342,6.88195296346427,6.92396857806303,
7.12842560393073,7.20118416663039,7.23329968825024,7.25909217247564,7.27508598783313,
7.29184467424206,7.32139292930927,7.45773062558618,7.5685713966976,7.61991187333395,
7.66362259442563,7.69347684144813,7.72050184056222,7.76526263232103,7.88528335382165,
7.99189141685828,8.03150313511859,8.06186693922171,8.07956174812618,8.0952715064761,
8.12421574543822,8.27870822290594,8.39568712496389,8.4392540033007,8.46906416428899,
8.49611927663557,8.54100630939177,8.72358332366881,8.80651700789685,8.84114464854317,
8.868422612394,8.88471481574657,8.901112591712,8.92890207034066,9.0830228697413,
9.23064667717671,9.27435570711325,9.30420923578343,9.33123385761761,9.37599469200737,
9.4967220998385,9.62391582345146,9.66552184744801,9.68530456554423,9.70205609939084,
9.72701089006405,9.81416045760381,9.94776797301862,10.0025472904076,10.047920929013,
10.0780412027337,10.1083527593252,10.1546524015123,10.3132481468407,10.4106500529436,
10.4651792677483,10.4860798856037,10.4952223301995),.UNSPECIFIED.);
#30169=B_SPLINE_CURVE_WITH_KNOTS('',3,(#171448,#171449,#171450,#171451,
#171452,#171453,#171454,#171455,#171456,#171457,#171458,#171459,#171460,
#171461,#171462,#171463,#171464,#171465,#171466,#171467,#171468,#171469,
#171470,#171471,#171472,#171473,#171474,#171475,#171476,#171477,#171478,
#171479,#171480,#171481,#171482,#171483,#171484,#171485,#171486,#171487,
#171488,#171489,#171490,#171491,#171492,#171493,#171494,#171495,#171496,
#171497,#171498,#171499,#171500,#171501,#171502,#171503,#171504,#171505,
#171506,#171507,#171508,#171509,#171510,#171511,#171512,#171513,#171514,
#171515,#171516,#171517,#171518,#171519,#171520,#171521,#171522,#171523,
#171524,#171525,#171526,#171527,#171528,#171529,#171530,#171531,#171532,
#171533,#171534,#171535,#171536,#171537,#171538,#171539,#171540,#171541,
#171542,#171543,#171544,#171545,#171546,#171547,#171548,#171549,#171550,
#171551,#171552,#171553,#171554,#171555,#171556,#171557,#171558,#171559,
#171560,#171561,#171562,#171563,#171564,#171565,#171566,#171567,#171568,
#171569,#171570,#171571,#171572,#171573,#171574,#171575,#171576,#171577,
#171578,#171579,#171580,#171581,#171582,#171583,#171584,#171585,#171586,
#171587,#171588,#171589,#171590,#171591,#171592,#171593,#171594,#171595,
#171596,#171597,#171598,#171599,#171600,#171601,#171602,#171603,#171604,
#171605,#171606,#171607,#171608,#171609,#171610,#171611,#171612,#171613,
#171614,#171615,#171616,#171617,#171618,#171619,#171620,#171621,#171622,
#171623,#171624,#171625,#171626,#171627,#171628,#171629,#171630,#171631,
#171632,#171633,#171634,#171635,#171636,#171637,#171638,#171639,#171640,
#171641,#171642,#171643,#171644,#171645,#171646,#171647,#171648,#171649,
#171650,#171651,#171652,#171653,#171654,#171655,#171656,#171657,#171658,
#171659,#171660,#171661,#171662,#171663,#171664,#171665,#171666,#171667,
#171668,#171669,#171670,#171671,#171672,#171673,#171674,#171675),
 .UNSPECIFIED.,.F.,.F.,(4,2,2,2,2,2,2,2,2,2,2,2,2,2,2,2,2,2,2,2,2,2,2,2,
2,2,2,2,2,2,2,2,2,2,2,2,2,2,2,2,2,2,2,2,2,2,2,2,2,2,2,2,2,2,2,2,2,2,2,2,
2,2,2,2,2,2,2,2,2,2,2,2,2,2,2,2,2,2,2,2,2,2,2,2,2,2,2,2,2,2,2,2,2,2,2,2,
2,2,2,2,2,2,2,2,2,2,2,2,2,2,2,2,2,4),(19.7725472889628,19.7745630841054,
19.7916200476201,19.8226511599206,19.8639329635955,19.9795410716252,20.1118258377354,
20.1587444018553,20.1891668403298,20.2191842746196,20.2639765147832,20.3903925148979,
20.5357674478223,20.5631467123286,20.5785937213992,20.5966940425543,20.6291110480684,
20.6725208085203,20.8028168600046,20.814012064891,20.9073302683404,20.94498528383,
20.9740327647176,21.0065941451291,21.0651024941645,21.1426041463908,21.2457967031782,
21.3448266654611,21.369429300689,21.3850413381192,21.4020980314289,21.4331286521571,
21.4744098018785,21.5900160785627,21.7222987490248,21.7692165698878,21.7996385264272,
21.829655485198,21.8744470157887,22.0008610132948,22.1462336432735,22.1736124740533,
22.1890592384218,22.207159272843,22.2395757648267,22.2829848376073,22.4132788250151,
22.4244738525792,22.5177905777285,22.5554449967101,22.584492017446,22.6170528820414,
22.6755603042281,22.7530607287287,22.8562516508049,22.9552800443077,22.979882289796,
22.9954940799104,23.0125505030194,23.0435806321822,23.0848611279569,23.2004655732939,
23.3327461482097,23.3796632258316,23.4100847004467,23.4401011837089,23.4848920047424,
23.6113039996843,23.7566743267646,23.7840527238278,23.7994992434982,23.8175989911895,
23.8500149696512,23.8934233547716,24.0237152781391,24.0349101283707,24.128225375247,
24.1658791977297,24.1949257583198,24.2274861071055,24.2859926024538,24.3634917992416,
24.466681086628,24.5657079113769,24.590309767131,24.6059213099325,24.6229774628435,
24.6540071004445,24.6952869422768,24.8108895562715,24.9431680356764,24.9900843700649,
25.0205053627607,25.0505213705191,25.0953114820017,25.2217214743951,25.3670894986047,
25.394467461955,25.409913736931,25.4280131978972,25.4604286628444,25.5038363603156,
25.6341262196795,25.6453208925587,25.7386346611949,25.7762878871884,25.8053339876401,
25.8378938206237,25.8963993891451,25.9738973582341,26.1364067009837,26.1837594997724,
26.2010247288919,26.214356777113),.UNSPECIFIED.);
#30170=B_SPLINE_CURVE_WITH_KNOTS('',3,(#171676,#171677,#171678,#171679,
#171680,#171681,#171682,#171683,#171684,#171685,#171686,#171687,#171688,
#171689,#171690,#171691,#171692,#171693,#171694,#171695,#171696,#171697,
#171698,#171699,#171700,#171701,#171702,#171703,#171704,#171705,#171706,
#171707,#171708,#171709,#171710,#171711,#171712,#171713,#171714,#171715,
#171716,#171717,#171718,#171719,#171720,#171721,#171722,#171723,#171724,
#171725,#171726,#171727,#171728,#171729,#171730,#171731,#171732,#171733,
#171734,#171735,#171736,#171737,#171738,#171739,#171740,#171741,#171742,
#171743,#171744,#171745,#171746,#171747,#171748,#171749,#171750,#171751,
#171752,#171753,#171754,#171755,#171756,#171757,#171758,#171759,#171760,
#171761,#171762,#171763,#171764,#171765,#171766,#171767,#171768,#171769,
#171770,#171771,#171772,#171773,#171774,#171775,#171776,#171777,#171778,
#171779,#171780,#171781,#171782,#171783,#171784,#171785,#171786,#171787,
#171788,#171789,#171790,#171791,#171792,#171793,#171794,#171795,#171796,
#171797,#171798,#171799,#171800,#171801,#171802,#171803,#171804,#171805,
#171806,#171807,#171808,#171809,#171810,#171811,#171812,#171813,#171814,
#171815,#171816,#171817,#171818,#171819,#171820,#171821,#171822,#171823,
#171824,#171825,#171826,#171827,#171828,#171829,#171830,#171831,#171832,
#171833,#171834,#171835,#171836,#171837,#171838,#171839,#171840,#171841,
#171842,#171843,#171844,#171845,#171846,#171847,#171848,#171849,#171850,
#171851,#171852,#171853,#171854,#171855,#171856,#171857,#171858,#171859,
#171860,#171861,#171862,#171863,#171864,#171865,#171866,#171867,#171868,
#171869,#171870,#171871,#171872,#171873,#171874,#171875,#171876,#171877,
#171878,#171879,#171880,#171881,#171882,#171883,#171884,#171885,#171886,
#171887),.UNSPECIFIED.,.F.,.F.,(4,2,2,2,2,2,2,2,2,2,2,2,2,2,2,2,2,2,2,2,
2,2,2,2,2,2,2,2,2,2,2,2,2,2,2,2,2,2,2,2,2,2,2,2,2,2,2,2,2,2,2,2,2,2,2,2,
2,2,2,2,2,2,2,2,2,2,2,2,2,2,2,2,2,2,2,2,2,2,2,2,2,2,2,2,2,2,2,2,2,2,2,2,
2,2,2,2,2,2,2,2,2,2,2,2,2,4),(10.4952223301995,10.5011982931848,10.5201141668262,
10.5612176483542,10.710837565267,10.8203497273949,10.8747647732625,10.9065791759548,
10.9358323362552,10.9757890810257,11.1048464791224,11.2127858288314,11.2526351230995,
11.283129772312,11.3008502417718,11.3165402711789,11.3453708443362,11.5000195295456,
11.6170390156557,11.6606110326317,11.6904219297176,11.7211151365107,11.7695005285895,
11.828562249715,11.9776778622939,12.0680464038359,12.0924593207554,12.1080383104008,
12.1251609048322,12.1565187049553,12.1984009800228,12.3174927727997,12.4571046596959,
12.498499574189,12.5276815076566,12.5588752114482,12.6102098212781,12.6450479632141,
12.759799544636,12.8649609089739,12.8945062003926,12.9120406790426,12.9301937411356,
12.9628779515214,13.006792733061,13.1406938104117,13.2393422058225,13.277498416277,
13.3066065516965,13.3389096759854,13.3959895172866,13.6415455398334,13.6876856772709,
13.7079192110452,13.7231566936277,13.7423884942477,13.7854045169452,13.8515218100554,
14.0502772104686,14.1001091521979,14.1310707122562,14.1607090457987,14.2032327874398,
14.3423846151305,14.4786192579758,14.5066981968369,14.5222606947975,14.540167348806,
14.5715997902277,14.6131688489649,14.7312876623688,14.847328371507,14.8870639054878,
14.9162870388762,14.9481909710892,15.003091530125,15.1070660983584,15.281143780499,
15.3099583083846,15.3265670217133,15.342674080297,15.3690401714997,15.493534994602,
15.6700149594369,15.7153427746451,15.7454795322935,15.775773039985,15.8221301669671,
15.8785897321692,16.0224155298113,16.0974217418858,16.1215490604885,16.1381996504406,
16.1584426685227,16.2028543121936,16.2721398430011,16.4553927504788,16.4962505619495,
16.5256311179101,16.5571081893088,16.6097086821471,16.7383535874396,16.893752455785,
16.9215410247633,16.9379384083926,16.9381046579605),.UNSPECIFIED.);
#30171=B_SPLINE_CURVE_WITH_KNOTS('',3,(#171892,#171893,#171894,#171895,
#171896,#171897,#171898,#171899,#171900,#171901,#171902,#171903,#171904,
#171905,#171906,#171907,#171908,#171909,#171910,#171911,#171912,#171913,
#171914,#171915,#171916,#171917,#171918,#171919,#171920,#171921,#171922,
#171923,#171924,#171925,#171926,#171927,#171928,#171929,#171930,#171931,
#171932,#171933,#171934,#171935,#171936,#171937,#171938,#171939,#171940,
#171941,#171942,#171943,#171944,#171945,#171946,#171947,#171948,#171949,
#171950,#171951,#171952,#171953,#171954,#171955,#171956,#171957,#171958,
#171959,#171960,#171961,#171962,#171963,#171964,#171965,#171966,#171967,
#171968,#171969,#171970,#171971,#171972,#171973,#171974,#171975,#171976,
#171977,#171978,#171979,#171980,#171981,#171982,#171983,#171984,#171985,
#171986,#171987,#171988,#171989,#171990,#171991,#171992,#171993,#171994,
#171995,#171996,#171997,#171998,#171999,#172000,#172001,#172002,#172003,
#172004,#172005,#172006,#172007,#172008,#172009,#172010,#172011,#172012,
#172013,#172014,#172015,#172016,#172017,#172018,#172019,#172020,#172021,
#172022,#172023,#172024,#172025,#172026,#172027,#172028,#172029,#172030,
#172031,#172032,#172033,#172034,#172035,#172036,#172037,#172038,#172039,
#172040,#172041,#172042,#172043,#172044,#172045,#172046,#172047,#172048,
#172049,#172050,#172051,#172052,#172053,#172054,#172055,#172056,#172057,
#172058,#172059,#172060,#172061,#172062,#172063,#172064,#172065,#172066,
#172067,#172068,#172069,#172070,#172071,#172072,#172073,#172074,#172075,
#172076,#172077,#172078,#172079,#172080,#172081,#172082,#172083,#172084,
#172085,#172086,#172087,#172088,#172089,#172090,#172091,#172092,#172093,
#172094,#172095,#172096,#172097,#172098,#172099,#172100,#172101,#172102,
#172103,#172104,#172105,#172106,#172107,#172108,#172109,#172110,#172111,
#172112,#172113,#172114,#172115,#172116,#172117),.UNSPECIFIED.,.F.,.F.,
(4,2,2,2,2,2,2,2,2,2,2,2,2,2,2,2,2,2,2,2,2,2,2,2,2,2,2,2,2,2,2,2,2,2,2,
2,2,2,2,2,2,2,2,2,2,2,2,2,2,2,2,2,2,2,2,2,2,2,2,2,2,2,2,2,2,2,2,2,2,2,2,
2,2,2,2,2,2,2,2,2,2,2,2,2,2,2,2,2,2,2,2,2,2,2,2,2,2,2,2,2,2,2,2,2,2,2,2,
2,2,2,2,2,4),(13.3303028304434,13.3458863286888,13.3725516882644,13.4061359908023,
13.4847270614522,13.6759450464462,13.7198704120896,13.7467739054654,13.7767481029321,
13.8212814221794,13.9456252700599,14.0937325303308,14.1210689909734,14.1365098200614,
14.1546244755228,14.1871107313086,14.2306501286573,14.3618496144961,14.3712773604203,
14.4651102512911,14.5028139166799,14.5318685537057,14.5644070577876,14.622780848882,
14.7000165668204,14.803240976931,14.9027378911907,14.9273515713224,14.9429662990634,
14.9600209165184,14.9910377049003,15.0322924891111,15.1477404423996,15.2802530093577,
15.3271739658346,15.3575978832191,15.3876167246649,15.4324109611222,15.5588318702412,
15.7042153453161,15.7315958150163,15.7470435444722,15.7651447582422,15.7975634600849,
15.8409755746499,15.9712798357069,15.9824693531093,16.0757950332109,16.1134520915238,
16.1425009857032,16.1750637847203,16.2335741805707,16.3110780713012,16.4142756827816,
16.5133128430796,16.5379167027833,16.5535294938141,16.5705869832614,16.6016189978069,
16.642901958538,16.758512847704,16.8908030274003,16.9377230865701,16.9681464938793,
16.9981648836962,17.0429585488897,17.1693785651203,17.3147581392816,17.3421382747194,
17.3575857754761,17.3756866731555,17.4081047119725,17.4515158567751,17.5818160724451,
17.5930115847522,17.6863327831989,17.7239889995254,17.75303740547,17.7855998215379,
17.8441100275484,17.9216141358451,18.0248099792089,18.1238431139926,18.1484465329417,
18.1640590675117,18.1811163037496,18.2121479117771,18.2534303745975,18.3690403249464,
18.5013272165901,18.5482465312657,18.5786694564029,18.6086873708738,18.6534803275609,
18.7798983498586,18.9252756084132,18.9526553108944,18.968102567067,18.9862031777716,
19.0186207018643,19.0620311567516,19.1923292926769,19.2035246762882,19.2968443727149,
19.3344999905819,19.3635479361403,19.3961098374245,19.454619122368,19.5321220142945,
19.6353162218491,19.7343477684474,19.7589507972439,19.7725472889628),
 .UNSPECIFIED.);
#30172=B_SPLINE_CURVE_WITH_KNOTS('',3,(#172118,#172119,#172120,#172121,
#172122,#172123,#172124,#172125,#172126,#172127,#172128,#172129,#172130,
#172131,#172132,#172133,#172134,#172135,#172136,#172137,#172138,#172139,
#172140,#172141,#172142,#172143,#172144,#172145,#172146,#172147,#172148,
#172149,#172150,#172151,#172152,#172153,#172154,#172155,#172156,#172157,
#172158,#172159,#172160,#172161,#172162,#172163,#172164,#172165,#172166,
#172167,#172168,#172169,#172170,#172171,#172172,#172173,#172174,#172175,
#172176,#172177,#172178,#172179,#172180,#172181,#172182,#172183,#172184,
#172185,#172186,#172187,#172188,#172189,#172190,#172191,#172192,#172193,
#172194,#172195,#172196,#172197,#172198,#172199,#172200,#172201,#172202,
#172203,#172204,#172205,#172206,#172207,#172208,#172209,#172210,#172211,
#172212,#172213,#172214,#172215,#172216,#172217,#172218,#172219,#172220,
#172221,#172222,#172223,#172224,#172225,#172226,#172227,#172228,#172229,
#172230,#172231,#172232,#172233,#172234,#172235,#172236,#172237,#172238,
#172239,#172240,#172241,#172242,#172243,#172244,#172245,#172246,#172247,
#172248,#172249,#172250,#172251,#172252,#172253,#172254,#172255,#172256,
#172257,#172258,#172259,#172260,#172261,#172262,#172263,#172264,#172265,
#172266,#172267,#172268,#172269,#172270,#172271,#172272,#172273,#172274,
#172275,#172276,#172277,#172278,#172279,#172280,#172281,#172282,#172283,
#172284,#172285,#172286,#172287,#172288,#172289,#172290,#172291,#172292,
#172293,#172294,#172295,#172296,#172297,#172298,#172299,#172300,#172301,
#172302,#172303,#172304,#172305,#172306,#172307,#172308,#172309,#172310,
#172311,#172312,#172313,#172314,#172315,#172316,#172317,#172318,#172319,
#172320,#172321,#172322,#172323,#172324,#172325,#172326,#172327,#172328,
#172329,#172330,#172331),.UNSPECIFIED.,.F.,.F.,(4,2,2,2,2,2,2,2,2,2,2,2,
2,2,2,2,2,2,2,2,2,2,2,2,2,2,2,2,2,2,2,2,2,2,2,2,2,2,2,2,2,2,2,2,2,2,2,2,
2,2,2,2,2,2,2,2,2,2,2,2,2,2,2,2,2,2,2,2,2,2,2,2,2,2,2,2,2,2,2,2,2,2,2,2,
2,2,2,2,2,2,2,2,2,2,2,2,2,2,2,2,2,2,2,2,2,2,4),(16.9381046579605,16.9542302905378,
16.9815079559571,17.0161358369833,17.0990705756198,17.281663301635,17.326549864848,
17.3536045109049,17.3834139473609,17.4269794760336,17.5439546486233,17.6984511933568,
17.7273810036705,17.7430880273296,17.7607854896951,17.7911643203876,17.8308041244526,
17.9375671978045,18.0682962903425,18.1082285607795,18.1374781231329,18.1693017554341,
18.2237682312351,18.3321706252319,18.4795226022105,18.5228614178865,18.5421452229526,
18.5573792669162,18.5779107226447,18.6296544540729,18.7185914269492,18.890953761646,
18.9364903724993,18.9666642333328,18.9969183204702,19.0430541862303,19.0991338405693,
19.2405506256492,19.3184585592705,19.3427372301077,19.3594046237519,19.3795573368572,
19.4234070666597,19.4913104405511,19.6779605326234,19.7183153435066,19.7476231003178,
19.7792817711919,19.8328603398126,19.9634779221162,20.1149427588734,20.1428266872479,
20.1592436514563,20.1755166479756,20.2027028788878,20.3198431657269,20.5031939377934,
20.5480098810489,20.5750529876773,20.6048731800791,20.6485048061577,20.676078352161,
20.7550230088709,20.8598185225424,20.9290951282174,20.9533949765663,20.9700643472372,
20.9902035745078,21.0339724360505,21.1016797315993,21.2888092142557,21.3290899043742,
21.3583864408186,21.3900715902998,21.4437966655168,21.5550304345355,21.7058183901195,
21.7457737084136,21.764493496282,21.7797795670898,21.8010575967874,21.8586169404002,
21.9660703604165,22.1095203892109,22.1563819667218,22.1867943136484,22.2168211546372,
22.2616659667345,22.3885012027066,22.5332116036451,22.5606623169395,22.5761210114605,
22.5942007575406,22.6265121584786,22.6697225955412,22.7986257088523,22.8159852915396,
22.9057314308541,22.9430815651382,22.9720955805802,23.0048273479192,23.064282535774,
23.1436545541524,23.3102516102636,23.3521031003166,23.3680703288497,23.3806731202454),
 .UNSPECIFIED.);
#30173=B_SPLINE_CURVE_WITH_KNOTS('',3,(#172334,#172335,#172336,#172337,
#172338,#172339,#172340,#172341,#172342,#172343,#172344,#172345,#172346,
#172347,#172348,#172349,#172350,#172351,#172352,#172353,#172354,#172355,
#172356,#172357,#172358,#172359,#172360,#172361,#172362,#172363,#172364,
#172365,#172366,#172367,#172368,#172369,#172370,#172371,#172372,#172373,
#172374,#172375,#172376,#172377,#172378,#172379,#172380,#172381,#172382,
#172383,#172384,#172385,#172386,#172387,#172388,#172389,#172390,#172391,
#172392,#172393,#172394,#172395,#172396,#172397,#172398,#172399,#172400,
#172401,#172402,#172403,#172404,#172405,#172406,#172407,#172408,#172409,
#172410,#172411,#172412,#172413,#172414,#172415,#172416,#172417,#172418,
#172419,#172420,#172421,#172422,#172423,#172424,#172425,#172426,#172427,
#172428,#172429,#172430,#172431,#172432,#172433,#172434,#172435,#172436,
#172437,#172438,#172439,#172440,#172441,#172442,#172443,#172444,#172445,
#172446,#172447,#172448,#172449,#172450,#172451,#172452,#172453,#172454,
#172455,#172456,#172457,#172458,#172459,#172460,#172461,#172462,#172463,
#172464,#172465,#172466,#172467,#172468,#172469,#172470,#172471,#172472,
#172473,#172474,#172475,#172476,#172477,#172478,#172479,#172480,#172481,
#172482,#172483,#172484,#172485,#172486,#172487,#172488,#172489,#172490,
#172491,#172492,#172493,#172494,#172495,#172496,#172497,#172498,#172499,
#172500,#172501,#172502,#172503,#172504,#172505,#172506,#172507,#172508,
#172509,#172510,#172511,#172512,#172513,#172514,#172515,#172516,#172517,
#172518,#172519,#172520,#172521,#172522,#172523,#172524,#172525,#172526,
#172527,#172528,#172529,#172530,#172531,#172532,#172533,#172534,#172535,
#172536,#172537,#172538,#172539,#172540,#172541,#172542,#172543,#172544,
#172545,#172546,#172547),.UNSPECIFIED.,.F.,.F.,(4,2,2,2,2,2,2,2,2,2,2,2,
2,2,2,2,2,2,2,2,2,2,2,2,2,2,2,2,2,2,2,2,2,2,2,2,2,2,2,2,2,2,2,2,2,2,2,2,
2,2,2,2,2,2,2,2,2,2,2,2,2,2,2,2,2,2,2,2,2,2,2,2,2,2,2,2,2,2,2,2,2,2,2,2,
2,2,2,2,2,2,2,2,2,2,2,2,2,2,2,2,2,2,2,2,2,2,4),(9.99999998048566E-7,0.00834286144590505,
0.0177640667967872,0.0443704512860533,0.221553904266857,0.324776256047929,
0.379415729592964,0.411272071436925,0.440511894327933,0.480366880991184,
0.670334133764149,0.736926102996499,0.780236264571233,0.800302085622393,
0.816988116744412,0.841420562650441,0.919654749145134,1.06060638730221,
1.1166147636061,1.16270935329757,1.19295728388864,1.22314016131068,1.26872095420009,
1.47289041591499,1.54092443341236,1.58475036792778,1.60411311821516,1.61934395744352,
1.63942842626298,1.68466555767539,1.93119791592704,1.98848249191259,2.02082404286317,
2.0499245319029,2.08800904734668,2.18426336945691,2.32021421986361,2.36440785725355,
2.39723956796959,2.41542206247379,2.43293496630915,2.4623655809095,2.57485795209346,
2.68491529535448,2.75605909595906,2.79060108383157,2.81944402763495,2.85487328097934,
2.93073928908664,2.97254590531705,3.12096301605404,3.16720229429947,3.20086986220605,
3.21844505952338,3.23383104101312,3.25707899360891,3.32983882344906,3.49408295297215,
3.55547920711643,3.60522732965993,3.63617422684778,3.66548738009172,3.70103665451084,
3.8950751093854,3.95978285991415,4.00230356596832,4.02223977402358,4.0389546510325,
4.06362143231028,4.14508193895005,4.28328645306604,4.33884742264124,4.38468072972562,
4.41488280468269,4.44511197082407,4.49094911775094,4.65784511985492,4.75011904504832,
4.78685643259309,4.815353005971,4.83189707030005,4.84805919618089,4.87469627736907,
5.04137366155528,5.16197423512273,5.21402548464954,5.24540195989211,5.27482963215457,
5.3159927581544,5.49713950832766,5.56730735531076,5.61207477474198,5.63237534482196,
5.64901726063103,5.67305448454816,5.74695604356235,5.89178865167136,5.94840797686942,
5.9948584944394,6.02517022769549,6.05529422481561,6.1005414456489,6.27842455005587,
6.36402201393951,6.4146057232201,6.43497826388505,6.44334884079168),
 .UNSPECIFIED.);
#30174=B_SPLINE_CURVE_WITH_KNOTS('',3,(#172550,#172551,#172552,#172553,
#172554,#172555,#172556,#172557,#172558,#172559,#172560,#172561,#172562,
#172563,#172564,#172565,#172566,#172567,#172568,#172569,#172570,#172571,
#172572,#172573,#172574,#172575,#172576,#172577,#172578,#172579,#172580,
#172581,#172582,#172583,#172584,#172585,#172586,#172587,#172588,#172589,
#172590,#172591,#172592,#172593,#172594,#172595,#172596,#172597,#172598,
#172599,#172600,#172601,#172602,#172603,#172604,#172605,#172606,#172607,
#172608,#172609,#172610,#172611,#172612,#172613,#172614,#172615,#172616,
#172617,#172618,#172619,#172620,#172621,#172622,#172623,#172624,#172625,
#172626,#172627,#172628,#172629,#172630,#172631,#172632,#172633,#172634,
#172635,#172636,#172637,#172638,#172639,#172640,#172641,#172642,#172643,
#172644,#172645,#172646,#172647,#172648,#172649,#172650,#172651,#172652,
#172653,#172654,#172655,#172656,#172657,#172658,#172659,#172660,#172661,
#172662,#172663,#172664,#172665,#172666,#172667,#172668,#172669,#172670,
#172671,#172672,#172673,#172674,#172675,#172676,#172677,#172678,#172679,
#172680,#172681,#172682,#172683,#172684,#172685,#172686,#172687,#172688,
#172689,#172690,#172691,#172692,#172693,#172694,#172695,#172696,#172697,
#172698,#172699,#172700,#172701,#172702,#172703,#172704,#172705,#172706,
#172707,#172708,#172709,#172710,#172711,#172712,#172713,#172714,#172715,
#172716,#172717,#172718,#172719,#172720,#172721,#172722,#172723,#172724,
#172725,#172726,#172727,#172728,#172729,#172730,#172731,#172732,#172733,
#172734,#172735,#172736,#172737,#172738,#172739,#172740,#172741,#172742,
#172743,#172744,#172745,#172746,#172747,#172748,#172749,#172750,#172751,
#172752,#172753,#172754,#172755,#172756,#172757,#172758,#172759,#172760,
#172761,#172762,#172763,#172764,#172765),.UNSPECIFIED.,.F.,.F.,(4,2,2,2,
2,2,2,2,2,2,2,2,2,2,2,2,2,2,2,2,2,2,2,2,2,2,2,2,2,2,2,2,2,2,2,2,2,2,2,2,
2,2,2,2,2,2,2,2,2,2,2,2,2,2,2,2,2,2,2,2,2,2,2,2,2,2,2,2,2,2,2,2,2,2,2,2,
2,2,2,2,2,2,2,2,2,2,2,2,2,2,2,2,2,2,2,2,2,2,2,2,2,2,2,2,2,2,2,4),(6.8874084212544,
6.8931476979918,6.91193457522707,6.95227471359089,7.10269181429562,7.21258566515954,
7.26698091127184,7.29879233467828,7.32804777647773,7.36801574908982,7.49612765992609,
7.60475441792588,7.64472596340581,7.67528814179571,7.6930223285844,7.70870312128107,
7.73747796699285,7.87094346979186,8.01151058958166,8.05406317889222,8.08370690190195,
8.11466188078627,8.1644548820903,8.36323289561284,8.4293761871952,8.47240398190068,
8.49163805792286,8.50687588749096,8.52710810825527,8.57323741716685,8.81883048471187,
8.87591736430399,8.90822245361849,8.93733117746541,8.97548646279464,9.07408042293343,
9.20801948114663,9.25193901682701,9.284626268699,9.30278027668346,9.32031488611257,
9.34985929740095,9.45473430520403,9.569698342345,9.60457381044061,9.6559463214887,
9.6871475416497,9.71632703695402,9.75770205494782,9.89901768809575,10.0168511978477,
10.0585188144546,10.0897607296006,10.1068605476429,10.122451904686,10.1469331931645,
10.2422392832044,10.3452626589476,10.4250348771085,10.4846916825598,10.5174611178321,
10.5464706291868,10.5837619496263,10.6729396529996,10.6911461266842,10.8199600911317,
10.8631582851443,10.8954641080057,10.913543601221,10.9290042253279,10.9564621737753,
11.101154215805,11.2280278623349,11.2728797275263,11.3029093124564,11.3333228775806,
11.3801831351613,11.5231030291366,11.6309462642744,11.6886188773855,11.7099114723339,
11.7251997742406,11.7439118613215,11.7838177072938,11.9346844582464,12.0447904378391,
12.0991709762353,12.1309790482828,12.160234475402,12.2002073852251,12.3274474868857,
12.4367031745351,12.4767846487415,12.5074069829761,12.5251527368355,12.5408242511039,
12.56954680696,12.7303728832813,12.8255731826283,12.8770870522267,12.9083137430622,
12.937480647036,12.9787745915852,13.1086034429492,13.2847225008811,13.3131830449594,
13.3297191004029,13.3303028304434),.UNSPECIFIED.);
#30175=B_SPLINE_CURVE_WITH_KNOTS('',3,(#172770,#172771,#172772,#172773,
#172774,#172775,#172776,#172777,#172778,#172779,#172780,#172781,#172782,
#172783,#172784,#172785,#172786,#172787,#172788,#172789,#172790,#172791,
#172792,#172793,#172794,#172795,#172796,#172797,#172798,#172799,#172800,
#172801,#172802,#172803,#172804,#172805,#172806,#172807,#172808,#172809,
#172810,#172811,#172812,#172813,#172814,#172815,#172816,#172817,#172818,
#172819,#172820,#172821,#172822,#172823,#172824,#172825,#172826,#172827,
#172828,#172829,#172830,#172831,#172832,#172833,#172834,#172835,#172836,
#172837,#172838,#172839,#172840,#172841,#172842,#172843,#172844,#172845,
#172846,#172847,#172848,#172849,#172850,#172851,#172852,#172853,#172854,
#172855,#172856,#172857,#172858,#172859,#172860,#172861,#172862,#172863,
#172864,#172865,#172866,#172867,#172868,#172869,#172870,#172871,#172872,
#172873,#172874,#172875,#172876,#172877,#172878,#172879,#172880,#172881,
#172882,#172883,#172884,#172885,#172886,#172887,#172888,#172889,#172890,
#172891,#172892,#172893,#172894,#172895,#172896,#172897,#172898,#172899,
#172900,#172901,#172902,#172903,#172904,#172905,#172906,#172907,#172908,
#172909,#172910,#172911,#172912,#172913,#172914,#172915,#172916,#172917,
#172918,#172919,#172920,#172921,#172922,#172923,#172924,#172925,#172926,
#172927,#172928,#172929,#172930,#172931,#172932,#172933,#172934,#172935,
#172936,#172937,#172938,#172939,#172940,#172941,#172942,#172943,#172944,
#172945,#172946,#172947,#172948,#172949,#172950,#172951,#172952,#172953,
#172954,#172955,#172956,#172957,#172958,#172959,#172960,#172961,#172962,
#172963,#172964,#172965,#172966,#172967,#172968,#172969,#172970,#172971,
#172972,#172973,#172974,#172975,#172976,#172977,#172978,#172979,#172980,
#172981,#172982,#172983,#172984,#172985,#172986,#172987,#172988,#172989),
 .UNSPECIFIED.,.F.,.F.,(4,2,2,2,2,2,2,2,2,2,2,2,2,2,2,2,2,2,2,2,2,2,2,2,
2,2,2,2,2,2,2,2,2,2,2,2,2,2,2,2,2,2,2,2,2,2,2,2,2,2,2,2,2,2,2,2,2,2,2,2,
2,2,2,2,2,2,2,2,2,2,2,2,2,2,2,2,2,2,2,2,2,2,2,2,2,2,2,2,2,2,2,2,2,2,2,2,
2,2,2,2,2,2,2,2,2,2,2,2,2,4),(0.444473727037554,0.44569666576656,0.462457412279222,
0.492014020454777,0.628329929449259,0.739182942359156,0.790527183277837,
0.834240640537556,0.864096106430243,0.891121802638194,0.935882755657428,
1.05763238444124,1.18434537221623,1.22560492572548,1.24532970898227,1.26209779708942,
1.28717017897574,1.37652478081576,1.50837964394317,1.54592545196543,1.59994381909527,
1.63162659240943,1.66093134393032,1.7011771809382,1.81597295936036,1.95640075266018,
2.02212106258482,2.04430825171449,2.05969560079507,2.07786089714591,2.11467755976525,
2.29598519843079,2.37334946652739,2.43178921120935,2.46434054448088,2.49339387246809,
2.53107763597037,2.6246989682917,2.63523112299089,2.76576497900819,2.80920998407807,
2.84164689624057,2.85975234835858,2.87519915604307,2.90257021858942,3.0481565985851,
3.17446229849664,3.21924399553585,3.24926185225053,3.27613078212855,3.31982889901256,
3.51276298776419,3.59054732950157,3.62393340306708,3.65048220980924,3.66662635419815,
3.68319110718666,3.71178954442697,3.85235133245311,4.01206874999574,4.05577982322363,
4.08563447664817,4.11265994735563,4.15742177377,4.2775826652578,4.38409014260239,
4.42368407807875,4.45403819762537,4.47173127926597,4.48744280901574,4.51639634910409,
4.6049069265807,4.73187270442656,4.76869064443234,4.82199715813846,4.85355035898922,
4.88290365767978,4.92349119774373,5.03921135224957,5.21878780455633,5.25457793594768,
5.272554326443,5.28798876060115,5.30691252884742,5.35880973149051,5.51742213530823,
5.59482048757793,5.65327780260943,5.68583250404732,5.7148854397096,5.75256384255149,
5.84612289040229,5.85546426649575,5.98699907233347,6.03058577321119,6.06309777725836,
6.0812180662375,6.09665706722825,6.12397891103025,6.27063851247635,6.39617504209887,
6.4408606715366,6.47086214161049,6.50131068343722,6.54835923024429,6.69508442948009,
6.79989183914482,6.85668284467142,6.8778684731313,6.8874084212544),
 .UNSPECIFIED.);
#30176=B_SPLINE_CURVE_WITH_KNOTS('',3,(#172990,#172991,#172992,#172993,
#172994,#172995,#172996,#172997,#172998,#172999,#173000,#173001,#173002,
#173003,#173004,#173005,#173006,#173007,#173008,#173009,#173010,#173011,
#173012,#173013,#173014,#173015,#173016,#173017,#173018,#173019,#173020,
#173021,#173022,#173023,#173024,#173025,#173026,#173027,#173028,#173029,
#173030,#173031,#173032,#173033,#173034,#173035,#173036,#173037,#173038,
#173039,#173040,#173041,#173042,#173043,#173044,#173045,#173046,#173047,
#173048,#173049,#173050,#173051,#173052,#173053,#173054,#173055,#173056,
#173057,#173058,#173059,#173060,#173061,#173062,#173063,#173064,#173065,
#173066,#173067,#173068,#173069,#173070,#173071,#173072,#173073,#173074,
#173075,#173076,#173077,#173078,#173079,#173080,#173081,#173082,#173083,
#173084,#173085,#173086,#173087,#173088,#173089,#173090,#173091,#173092,
#173093,#173094,#173095,#173096,#173097,#173098,#173099,#173100,#173101,
#173102,#173103,#173104,#173105,#173106,#173107,#173108,#173109,#173110,
#173111,#173112,#173113,#173114,#173115,#173116,#173117,#173118,#173119,
#173120,#173121,#173122,#173123,#173124,#173125,#173126,#173127,#173128,
#173129,#173130,#173131,#173132,#173133,#173134,#173135,#173136,#173137,
#173138,#173139,#173140,#173141,#173142,#173143,#173144,#173145,#173146,
#173147,#173148,#173149,#173150,#173151,#173152,#173153,#173154,#173155,
#173156,#173157,#173158,#173159,#173160,#173161,#173162,#173163,#173164,
#173165,#173166,#173167,#173168,#173169,#173170,#173171,#173172,#173173,
#173174,#173175,#173176,#173177,#173178,#173179,#173180,#173181,#173182,
#173183,#173184,#173185,#173186,#173187,#173188,#173189,#173190,#173191,
#173192,#173193,#173194,#173195,#173196,#173197,#173198,#173199,#173200,
#173201),.UNSPECIFIED.,.F.,.F.,(4,2,2,2,2,2,2,2,2,2,2,2,2,2,2,2,2,2,2,2,
2,2,2,2,2,2,2,2,2,2,2,2,2,2,2,2,2,2,2,2,2,2,2,2,2,2,2,2,2,2,2,2,2,2,2,2,
2,2,2,2,2,2,2,2,2,2,2,2,2,2,2,2,2,2,2,2,2,2,2,2,2,2,2,2,2,2,2,2,2,2,2,2,
2,2,2,2,2,2,2,2,2,2,2,2,2,4),(6.44334884079168,6.45020661119763,6.46962829037362,
6.51382335570583,6.66036685340636,6.78577784535818,6.83120544377829,6.86136155765678,
6.89163898631733,6.93789674469328,6.99418382632804,7.1368919406878,7.21319192619572,
7.23742255677102,7.25408559679794,7.2742692991809,7.31830497201757,7.38666050837615,
7.57221427647539,7.61273808710649,7.64207177564436,7.6736714254471,7.72692292198614,
7.97430722930759,8.02454260163753,8.04331673182283,8.05872399488782,8.07680814039745,
8.11317957995387,8.16477632272232,8.36548425929763,8.42747741939418,8.46100201245027,
8.48990698799265,8.52663010527001,8.6142051062479,8.78865428560555,8.83380175441251,
8.85416243677422,8.87079439690745,8.89473536845016,8.97120891903685,9.0662520061906,
9.18490175020454,9.22474828480411,9.25398845615285,9.28585119258864,9.34051816110509,
9.44264250555622,9.6200699409606,9.64830880663657,9.6648002157263,9.68100899289069,
9.70787455058517,9.83759081362432,10.0071875525531,10.0528712137266,10.0830735221571,
10.1133043724582,10.1592969213707,10.2151287991287,10.3549877822516,10.4344870168673,
10.4590162143119,10.4757144924983,10.4957273242045,10.5387102019195,10.6045155043423,
10.7965513012817,10.8321923609652,10.8615262268871,10.8924393597251,10.9420025825363,
11.0030780687583,11.1650954388579,11.2402967619581,11.2637538045953,11.2791729209072,
11.2966600310387,11.329869563942,11.3752292103597,11.5170414657339,11.6304658632159,
11.6705671218966,11.6998511283669,11.731589488876,11.7859175753562,11.9149149054604,
12.0359141003639,12.0651286074155,12.0826003724143,12.1008378806642,12.1339502525029,
12.1786794885646,12.3186733571335,12.4111894815271,12.4487858940284,12.4778293853812,
12.5104283916848,12.5691324033298,12.6470142965126,12.7362314298784,12.8392947638747,
12.8688111094762,12.8855635427888,12.8867645288586),.UNSPECIFIED.);
#30177=B_SPLINE_CURVE_WITH_KNOTS('',3,(#173232,#173233,#173234,#173235,
#173236,#173237,#173238,#173239,#173240,#173241,#173242,#173243,#173244,
#173245,#173246,#173247,#173248,#173249,#173250,#173251,#173252,#173253,
#173254,#173255,#173256,#173257,#173258,#173259,#173260,#173261,#173262,
#173263,#173264,#173265,#173266,#173267,#173268,#173269,#173270,#173271),
 .UNSPECIFIED.,.F.,.F.,(4,2,2,2,2,2,2,2,2,2,2,2,2,2,2,2,2,2,2,4),(12.8867645288586,
12.9015623774001,12.9273795904343,12.9595366430601,13.0324541294685,13.2369391272014,
13.2788483163085,13.3081109800271,13.339149325778,13.3896247662921,13.43390330168,
13.451409382202,13.4562541410545,13.5522040596861,13.6466306131858,13.6758263086521,
13.693294127577,13.7085327834317,13.7271129613633,13.7835751351093),
 .UNSPECIFIED.);
#30178=B_SPLINE_CURVE_WITH_KNOTS('',3,(#173274,#173275,#173276,#173277,
#173278,#173279,#173280,#173281,#173282,#173283,#173284,#173285,#173286,
#173287,#173288,#173289,#173290,#173291),.UNSPECIFIED.,.F.,.F.,(4,2,2,2,
2,2,2,2,4),(1.00000000165542E-6,0.0153017020044519,0.0305119587961849,0.0583363701016362,
0.103708540329548,0.274366722756818,0.403915594495088,0.429703415281917,
0.444473727037554),.UNSPECIFIED.);
#30179=B_SPLINE_CURVE_WITH_KNOTS('',3,(#173314,#173315,#173316,#173317,
#173318,#173319,#173320,#173321,#173322,#173323,#173324,#173325,#173326,
#173327,#173328,#173329,#173330,#173331,#173332,#173333,#173334,#173335,
#173336,#173337,#173338,#173339,#173340,#173341,#173342,#173343,#173344,
#173345,#173346,#173347,#173348,#173349,#173350,#173351,#173352,#173353,
#173354,#173355,#173356,#173357,#173358,#173359,#173360,#173361,#173362,
#173363,#173364,#173365,#173366,#173367,#173368,#173369,#173370,#173371,
#173372,#173373,#173374,#173375,#173376,#173377,#173378,#173379,#173380,
#173381,#173382,#173383,#173384,#173385,#173386,#173387,#173388,#173389,
#173390,#173391,#173392,#173393,#173394,#173395,#173396,#173397,#173398,
#173399,#173400,#173401,#173402,#173403,#173404,#173405,#173406,#173407,
#173408,#173409,#173410,#173411,#173412,#173413,#173414,#173415,#173416,
#173417,#173418,#173419,#173420,#173421,#173422,#173423,#173424,#173425,
#173426,#173427,#173428,#173429,#173430,#173431,#173432,#173433,#173434,
#173435,#173436,#173437,#173438,#173439,#173440,#173441,#173442,#173443,
#173444,#173445,#173446,#173447,#173448,#173449,#173450,#173451,#173452,
#173453,#173454,#173455,#173456,#173457,#173458,#173459,#173460,#173461,
#173462,#173463,#173464,#173465,#173466,#173467,#173468,#173469,#173470,
#173471,#173472,#173473,#173474,#173475,#173476,#173477,#173478,#173479,
#173480,#173481,#173482,#173483,#173484,#173485,#173486,#173487,#173488,
#173489,#173490,#173491,#173492,#173493,#173494,#173495,#173496,#173497,
#173498,#173499,#173500,#173501,#173502,#173503,#173504,#173505,#173506,
#173507,#173508,#173509,#173510,#173511),.UNSPECIFIED.,.F.,.F.,(4,2,2,2,
2,2,2,2,2,2,2,2,2,2,2,2,2,2,2,2,2,2,2,2,2,2,2,2,2,2,2,2,2,2,2,2,2,2,2,2,
2,2,2,2,2,2,2,2,2,2,2,2,2,2,2,2,2,2,2,2,2,2,2,2,2,2,2,2,2,2,2,2,2,2,2,2,
2,2,2,2,2,2,2,2,2,2,2,2,2,2,2,2,2,2,2,2,2,2,4),(6.28519602509786,6.28901353086328,
6.2973498731085,6.31473179191909,6.42061492088043,6.605250658758,6.65926549255974,
6.67919017382771,6.69245539621225,6.70535294312242,6.72342705860252,6.76886510629959,
6.83666704283505,6.97041023924232,7.04545627146495,7.06019146936096,7.06845088399039,
7.07483484998806,7.08382997653377,7.10261711445801,7.17900000490521,7.36327396446623,
7.41502638214024,7.43456662500351,7.44643453864809,7.45920520306252,7.47655660759406,
7.51727707013666,7.57459858058148,7.77668831880739,7.83375294956289,7.84694800156893,
7.85449967082409,7.86040009869791,7.86870581179625,7.88592945551878,8.02473005738236,
8.2071975499987,8.24036039948964,8.25637220524566,8.26895431395015,8.28304224537606,
8.30681334748901,8.41531234773116,8.54652830008896,8.61723628696111,8.63180153041676,
8.64002274575152,8.6464124487705,8.65546147724681,8.6745314739972,8.7533573826537,
8.95342346288724,8.99164092946578,9.00728489469574,9.01898174064997,9.03189436830331,
9.05004724167751,9.09584396633112,9.16312306337085,9.27024738630931,9.32485842043261,
9.4031696771062,9.41621986821084,9.42442840472778,9.43094967347004,9.43884584386771,
9.45402753468027,9.59186406686353,9.77909615207739,9.81190911692872,9.82785384375041,
9.84042835903054,9.85455502825018,9.87850798525611,9.99094178889568,10.1313997308747,
10.1898738032537,10.2038850793348,10.2118999816578,10.219051102569,10.2288907422188,
10.2524276058154,10.2868502454306,10.4016740345544,10.5349748157314,10.5671441261324,
10.5829564142464,10.5955179364463,10.6097278392607,10.6340515108208,10.748959280512,
10.9316121773167,10.955771170825,10.9826093996835,10.9926127145221,10.9993377269722,
11.0044125226315,11.0097303272946),.UNSPECIFIED.);
#30180=B_SPLINE_CURVE_WITH_KNOTS('',3,(#173514,#173515,#173516,#173517,
#173518,#173519,#173520,#173521,#173522,#173523,#173524,#173525,#173526,
#173527,#173528,#173529,#173530,#173531,#173532,#173533,#173534,#173535,
#173536,#173537,#173538,#173539,#173540,#173541,#173542,#173543,#173544,
#173545,#173546,#173547,#173548,#173549,#173550,#173551,#173552,#173553,
#173554,#173555,#173556,#173557,#173558,#173559,#173560,#173561,#173562,
#173563,#173564,#173565,#173566,#173567,#173568,#173569,#173570,#173571,
#173572,#173573,#173574,#173575,#173576,#173577,#173578,#173579,#173580,
#173581,#173582,#173583,#173584,#173585,#173586,#173587,#173588,#173589,
#173590,#173591,#173592,#173593,#173594,#173595,#173596,#173597,#173598,
#173599,#173600,#173601,#173602,#173603,#173604,#173605,#173606,#173607,
#173608,#173609,#173610,#173611,#173612,#173613,#173614,#173615,#173616,
#173617,#173618,#173619,#173620,#173621,#173622,#173623,#173624,#173625,
#173626,#173627,#173628,#173629,#173630,#173631,#173632,#173633,#173634,
#173635,#173636,#173637,#173638,#173639,#173640,#173641,#173642,#173643,
#173644,#173645,#173646,#173647,#173648,#173649,#173650,#173651,#173652,
#173653,#173654,#173655,#173656,#173657,#173658,#173659,#173660,#173661,
#173662,#173663,#173664,#173665,#173666,#173667,#173668,#173669,#173670,
#173671,#173672,#173673,#173674,#173675,#173676,#173677,#173678,#173679,
#173680,#173681,#173682,#173683,#173684,#173685,#173686,#173687,#173688,
#173689,#173690,#173691,#173692,#173693,#173694,#173695,#173696,#173697,
#173698,#173699),.UNSPECIFIED.,.F.,.F.,(4,2,2,2,2,2,2,2,2,2,2,2,2,2,2,2,
2,2,2,2,2,2,2,2,2,2,2,2,2,2,2,2,2,2,2,2,2,2,2,2,2,2,2,2,2,2,2,2,2,2,2,2,
2,2,2,2,2,2,2,2,2,2,2,2,2,2,2,2,2,2,2,2,2,2,2,2,2,2,2,2,2,2,2,2,2,2,2,2,
2,2,2,2,4),(0.000200536233982881,0.138417303990259,0.172812251864514,0.189055178724505,
0.201663628280664,0.215622323018577,0.238795084007953,0.324791897898088,
0.349164011317468,0.483038165431939,0.529190380219428,0.558082580182329,
0.568846010764633,0.576158804245789,0.583816249184777,0.596196363279018,
0.635879329593167,0.793951507471554,0.910369046537782,0.934492994205679,
0.94865676861636,0.961225662802842,0.977111037346156,1.0096123392182,1.24008206304933,
1.3058522261296,1.34258968533793,1.35371178764923,1.36072973518842,1.36741786276578,
1.37571719549323,1.39663294066603,1.51392738001782,1.61206476455402,1.72656329446571,
1.75086856488995,1.76507508092252,1.77763803902874,1.79345806928563,1.82566447178002,
1.9713069348334,2.03119738309361,2.12142743581017,2.13636698783731,2.14458225005192,
2.15168618158042,2.16100026055674,2.18205518653002,2.28996921622105,2.37950931646946,
2.48292581799482,2.50643889609789,2.52047141804266,2.53306459706185,2.5491740066023,
2.58285221788166,2.75592853625272,2.891621210336,2.91699655937253,2.92668873863429,
2.93340629854986,2.94050355968752,2.95198503164026,2.98830085870527,3.14322440438076,
3.27340149106296,3.31308653581341,3.33026555465513,3.34300828421071,3.3565533039302,
3.37780663550806,3.44338973399375,3.61294020032678,3.66745629889736,3.70008460904966,
3.71123548842394,3.71862697381515,3.72526996051674,3.73633943994479,3.76590845038749,
3.91302234215016,4.03116695838225,4.06893198951861,4.08576711212521,4.09845597275285,
4.11213655269138,4.13401086864785,4.20431447764165,4.37437172967117,4.47886302722555,
4.49351606379445,4.50130236743711,4.50400203993545),.UNSPECIFIED.);
#30181=B_SPLINE_CURVE_WITH_KNOTS('',3,(#173703,#173704,#173705,#173706,
#173707,#173708),.UNSPECIFIED.,.F.,.F.,(4,2,4),(-0.262354516905103,-0.131154285438883,
-9.9978299089587E-7),.UNSPECIFIED.);
#30182=B_SPLINE_CURVE_WITH_KNOTS('',3,(#173710,#173711,#173712,#173713,
#173714,#173715,#173716,#173717,#173718,#173719,#173720,#173721,#173722,
#173723,#173724,#173725),.UNSPECIFIED.,.F.,.F.,(4,2,2,2,2,2,2,4),(9.99999994500671E-7,
0.369172740514888,0.675655915500258,1.11184046459798,1.56416421463315,2.08483397497198,
2.35023008390774,2.63088244313733),.UNSPECIFIED.);
#30183=B_SPLINE_CURVE_WITH_KNOTS('',3,(#173727,#173728,#173729,#173730,
#173731,#173732,#173733,#173734,#173735,#173736,#173737,#173738,#173739,
#173740,#173741,#173742,#173743,#173744,#173745,#173746,#173747,#173748),
 .UNSPECIFIED.,.F.,.F.,(4,2,2,2,2,2,2,2,2,2,4),(2.63088244313733,2.69546818234403,
3.0348688318089,3.19115119671758,3.55687823384515,3.99038170602948,4.20896941662107,
4.74902248620587,5.2734511797038,5.85070004788538,6.57223423227542),
 .UNSPECIFIED.);
#30184=B_SPLINE_CURVE_WITH_KNOTS('',3,(#173752,#173753,#173754,#173755,
#173756,#173757,#173758,#173759,#173760,#173761,#173762,#173763,#173764,
#173765,#173766,#173767,#173768,#173769,#173770,#173771,#173772,#173773,
#173774,#173775),.UNSPECIFIED.,.F.,.F.,(4,2,2,2,2,2,2,2,2,2,2,4),(2.75893124092028,
3.47129380746993,3.91475560027265,4.62575754639855,5.13958137759193,5.62273924852717,
6.07205236472011,6.47892216149857,6.92327779350677,7.28438064116319,7.53542186624699,
7.78890090561998),.UNSPECIFIED.);
#30185=B_SPLINE_CURVE_WITH_KNOTS('',3,(#173779,#173780,#173781,#173782,
#173783,#173784,#173785,#173786,#173787,#173788,#173789,#173790,#173791,
#173792),.UNSPECIFIED.,.F.,.F.,(4,2,2,2,2,2,4),(9.99999998254383E-7,0.400379609020636,
0.849460616516701,1.36345993017091,1.96278107846063,2.643590982597,2.75893124092028),
 .UNSPECIFIED.);
#30186=B_SPLINE_CURVE_WITH_KNOTS('',3,(#173827,#173828,#173829,#173830,
#173831,#173832,#173833,#173834,#173835,#173836,#173837,#173838,#173839,
#173840,#173841,#173842,#173843,#173844),.UNSPECIFIED.,.F.,.F.,(4,2,2,2,
2,2,2,2,4),(0.00026697786525906,0.248328138175261,0.378660605109992,0.616962714032332,
1.00025039751551,1.28920300639177,1.42688012206986,1.9141195649657,2.27710571623716),
 .UNSPECIFIED.);
#30187=B_SPLINE_CURVE_WITH_KNOTS('',3,(#173845,#173846,#173847,#173848,
#173849,#173850,#173851,#173852,#173853,#173854,#173855,#173856,#173857,
#173858,#173859,#173860,#173861,#173862,#173863,#173864,#173865,#173866,
#173867,#173868,#173869,#173870,#173871,#173872,#173873,#173874,#173875,
#173876,#173877,#173878),.UNSPECIFIED.,.F.,.F.,(4,2,2,2,2,2,2,2,2,2,2,2,
2,2,2,2,4),(1.00000001235279E-6,0.284067726320766,0.475326776009137,0.748904955936679,
1.14607740629631,1.50603295057684,1.93520778592777,2.3935701797541,2.90506409166115,
3.44391786134405,3.87621012480206,4.36338426004738,4.55553335566627,5.1694239011698,
5.65334987446971,5.87721795904605,5.94644245477199),.UNSPECIFIED.);
#30188=B_SPLINE_CURVE_WITH_KNOTS('',3,(#173881,#173882,#173883,#173884,
#173885,#173886,#173887,#173888,#173889,#173890,#173891,#173892,#173893,
#173894,#173895,#173896,#173897,#173898,#173899,#173900,#173901,#173902,
#173903,#173904,#173905,#173906,#173907,#173908,#173909,#173910,#173911,
#173912,#173913,#173914),.UNSPECIFIED.,.F.,.F.,(4,2,2,2,2,2,2,2,2,2,2,2,
2,2,2,2,4),(2.42138039423514,2.94917661332815,3.69054276678486,4.50082126956817,
5.42793599331964,6.36346209958375,7.33447465668507,7.84009893881512,9.16241399297696,
10.3457374091789,11.9263428378431,13.3309430649595,14.0568928218673,15.8227739100455,
17.3107175510575,19.078104485536,20.8484436842247),.UNSPECIFIED.);
#30189=B_SPLINE_CURVE_WITH_KNOTS('',3,(#173915,#173916,#173917,#173918,
#173919,#173920,#173921,#173922,#173923,#173924,#173925,#173926,#173927,
#173928,#173929,#173930,#173931,#173932),.UNSPECIFIED.,.F.,.F.,(4,2,2,2,
2,2,2,2,4),(-3.11844708417124,-2.64468204992212,-2.24234014729625,-1.61104523883494,
-1.0918992231367,-0.789389280194095,-0.622416825135047,-0.261781713236578,
-9.99995018347022E-7),.UNSPECIFIED.);
#30190=B_SPLINE_CURVE_WITH_KNOTS('',3,(#173933,#173934,#173935,#173936,
#173937,#173938,#173939,#173940,#173941,#173942,#173943,#173944,#173945,
#173946),.UNSPECIFIED.,.F.,.F.,(4,2,2,2,2,2,4),(9.99999998881322E-7,0.263909788184675,
0.673262348384023,1.16230828562023,1.70456174986609,2.30630414009246,2.42138039423514),
 .UNSPECIFIED.);
#30191=B_SPLINE_CURVE_WITH_KNOTS('',3,(#173951,#173952,#173953,#173954,
#173955,#173956,#173957,#173958,#173959,#173960,#173961,#173962,#173963,
#173964,#173965,#173966,#173967,#173968,#173969,#173970,#173971,#173972,
#173973,#173974,#173975,#173976,#173977,#173978,#173979,#173980,#173981,
#173982,#173983,#173984,#173985,#173986,#173987,#173988,#173989,#173990,
#173991,#173992,#173993,#173994),.UNSPECIFIED.,.F.,.F.,(4,2,2,2,2,2,2,2,
2,2,2,2,2,2,2,2,2,2,2,2,2,4),(-0.918151647035043,-0.917455501213576,-0.910381510809376,
-0.898993721060337,-0.859445308085101,-0.784707091077987,-0.585182429345266,
-0.554177150673725,-0.538389469005455,-0.525829981835348,-0.51159222440807,
-0.487088487493674,-0.387504063757192,-0.286760142516632,-0.202034274519989,
-0.184112852766584,-0.175292583613589,-0.16822888003932,-0.159455088186085,
-0.141770058164199,-0.118131103261592,-9.99999999917733E-7),
 .UNSPECIFIED.);
#30192=B_SPLINE_CURVE_WITH_KNOTS('',3,(#173995,#173996,#173997,#173998,
#173999,#174000,#174001,#174002,#174003,#174004,#174005,#174006,#174007,
#174008,#174009,#174010,#174011,#174012,#174013,#174014,#174015,#174016,
#174017,#174018),.UNSPECIFIED.,.F.,.F.,(4,2,2,2,2,2,2,2,2,2,2,4),(-21.2972205327464,
-21.2900945455965,-21.2827776382084,-21.2687259488357,-21.2442239997285,
-21.1220249620756,-21.0309934027925,-20.990754061758,-20.9453911008694,
-20.917065047827,-20.9069670168058,-20.9006012202032),.UNSPECIFIED.);
#30193=B_SPLINE_CURVE_WITH_KNOTS('',3,(#174020,#174021,#174022,#174023,
#174024,#174025,#174026,#174027,#174028,#174029,#174030,#174031,#174032,
#174033,#174034,#174035,#174036,#174037,#174038,#174039),.UNSPECIFIED.,
 .F.,.F.,(4,2,2,2,2,2,2,2,2,4),(-0.634450996246336,-0.622865914713776,-0.599688377221672,
-0.517041024851767,-0.319266063390083,-0.277934609428317,-0.248507740710781,
-0.217016410888511,-0.184161387630576,-1.00000001346245E-6),
 .UNSPECIFIED.);
#31187=CIRCLE('',#80524,9.35);
#31188=CIRCLE('',#80531,9.35);
#31189=CIRCLE('',#80533,9.49999999999999);
#31190=CIRCLE('',#80541,9.49999999999999);
#31191=CIRCLE('',#80543,10.);
#31192=CIRCLE('',#80549,10.25);
#31193=CIRCLE('',#80556,7.25);
#31194=CIRCLE('',#80558,10.25);
#31195=CIRCLE('',#80560,9.25);
#31196=CIRCLE('',#80561,9.25);
#31197=CIRCLE('',#80562,9.25);
#31198=CIRCLE('',#80564,11.);
#31199=CIRCLE('',#80565,11.);
#31200=CIRCLE('',#80567,9.15);
#31201=CIRCLE('',#80568,9.15);
#31202=CIRCLE('',#80570,10.);
#31203=CIRCLE('',#80572,9.35);
#31204=CIRCLE('',#80574,9.50000000000001);
#31205=CIRCLE('',#80575,91.074321383489);
#31206=CIRCLE('',#80577,7.75);
#31207=CIRCLE('',#80578,7.75);
#31208=CIRCLE('',#80579,7.75);
#31209=CIRCLE('',#80581,6.5);
#31210=CIRCLE('',#80582,6.5);
#31211=CIRCLE('',#80584,6.75);
#31212=CIRCLE('',#80585,0.25);
#31213=CIRCLE('',#80587,0.5);
#31214=CIRCLE('',#80588,8.25);
#31215=CIRCLE('',#80590,4.);
#31216=CIRCLE('',#80591,4.);
#31217=CIRCLE('',#80593,9.49999999999999);
#31218=CIRCLE('',#80595,9.25);
#31219=CIRCLE('',#80602,4.);
#31220=CIRCLE('',#80603,4.);
#34623=VERTEX_POINT('',#161939);
#34624=VERTEX_POINT('',#161940);
#34625=VERTEX_POINT('',#161942);
#34626=VERTEX_POINT('',#162145);
#34627=VERTEX_POINT('',#162328);
#34628=VERTEX_POINT('',#162329);
#34629=VERTEX_POINT('',#162746);
#34630=VERTEX_POINT('',#162955);
#34631=VERTEX_POINT('',#163164);
#34632=VERTEX_POINT('',#163165);
#34633=VERTEX_POINT('',#163570);
#34634=VERTEX_POINT('',#163571);
#34635=VERTEX_POINT('',#163773);
#34636=VERTEX_POINT('',#163991);
#34637=VERTEX_POINT('',#163992);
#34638=VERTEX_POINT('',#164419);
#34639=VERTEX_POINT('',#164420);
#34640=VERTEX_POINT('',#164422);
#34641=VERTEX_POINT('',#164831);
#34642=VERTEX_POINT('',#164832);
#34643=VERTEX_POINT('',#164834);
#34644=VERTEX_POINT('',#164973);
#34645=VERTEX_POINT('',#165104);
#34646=VERTEX_POINT('',#165105);
#34647=VERTEX_POINT('',#165634);
#34648=VERTEX_POINT('',#165635);
#34649=VERTEX_POINT('',#166148);
#34650=VERTEX_POINT('',#166149);
#34651=VERTEX_POINT('',#166151);
#34652=VERTEX_POINT('',#166412);
#34653=VERTEX_POINT('',#166684);
#34654=VERTEX_POINT('',#166685);
#34655=VERTEX_POINT('',#167208);
#34656=VERTEX_POINT('',#167209);
#34657=VERTEX_POINT('',#167728);
#34658=VERTEX_POINT('',#167729);
#34659=VERTEX_POINT('',#168254);
#34660=VERTEX_POINT('',#168255);
#34661=VERTEX_POINT('',#168281);
#34662=VERTEX_POINT('',#168282);
#34663=VERTEX_POINT('',#168284);
#34664=VERTEX_POINT('',#168455);
#34665=VERTEX_POINT('',#168628);
#34666=VERTEX_POINT('',#168629);
#34667=VERTEX_POINT('',#169156);
#34668=VERTEX_POINT('',#169157);
#34669=VERTEX_POINT('',#169672);
#34670=VERTEX_POINT('',#169673);
#34671=VERTEX_POINT('',#170190);
#34672=VERTEX_POINT('',#170191);
#34673=VERTEX_POINT('',#170716);
#34674=VERTEX_POINT('',#170717);
#34675=VERTEX_POINT('',#170719);
#34676=VERTEX_POINT('',#170874);
#34677=VERTEX_POINT('',#171015);
#34678=VERTEX_POINT('',#171016);
#34679=VERTEX_POINT('',#171445);
#34680=VERTEX_POINT('',#171446);
#34681=VERTEX_POINT('',#171889);
#34682=VERTEX_POINT('',#171890);
#34683=VERTEX_POINT('',#172333);
#34684=VERTEX_POINT('',#172548);
#34685=VERTEX_POINT('',#172767);
#34686=VERTEX_POINT('',#172768);
#34687=VERTEX_POINT('',#173203);
#34688=VERTEX_POINT('',#173204);
#34689=VERTEX_POINT('',#173208);
#34690=VERTEX_POINT('',#173212);
#34691=VERTEX_POINT('',#173216);
#34692=VERTEX_POINT('',#173219);
#34693=VERTEX_POINT('',#173223);
#34694=VERTEX_POINT('',#173231);
#34695=VERTEX_POINT('',#173272);
#34696=VERTEX_POINT('',#173293);
#34697=VERTEX_POINT('',#173295);
#34698=VERTEX_POINT('',#173297);
#34699=VERTEX_POINT('',#173301);
#34700=VERTEX_POINT('',#173303);
#34701=VERTEX_POINT('',#173307);
#34702=VERTEX_POINT('',#173309);
#34703=VERTEX_POINT('',#173313);
#34704=VERTEX_POINT('',#173512);
#34705=VERTEX_POINT('',#173701);
#34706=VERTEX_POINT('',#173709);
#34707=VERTEX_POINT('',#173750);
#34708=VERTEX_POINT('',#173751);
#34709=VERTEX_POINT('',#173776);
#34710=VERTEX_POINT('',#173795);
#34711=VERTEX_POINT('',#173796);
#34712=VERTEX_POINT('',#173798);
#34713=VERTEX_POINT('',#173803);
#34714=VERTEX_POINT('',#173805);
#34715=VERTEX_POINT('',#173809);
#34716=VERTEX_POINT('',#173813);
#34717=VERTEX_POINT('',#173817);
#34718=VERTEX_POINT('',#173818);
#34719=VERTEX_POINT('',#173820);
#34720=VERTEX_POINT('',#173822);
#34721=VERTEX_POINT('',#173880);
#34722=VERTEX_POINT('',#173947);
#34723=VERTEX_POINT('',#174617);
#34724=VERTEX_POINT('',#174619);
#34725=VERTEX_POINT('',#174623);
#34726=VERTEX_POINT('',#174625);
#34727=VERTEX_POINT('',#174629);
#34728=VERTEX_POINT('',#174631);
#34729=VERTEX_POINT('',#174635);
#34730=VERTEX_POINT('',#174637);
#34731=VERTEX_POINT('',#174641);
#34732=VERTEX_POINT('',#174643);
#34733=VERTEX_POINT('',#174647);
#34734=VERTEX_POINT('',#174649);
#34735=VERTEX_POINT('',#174658);
#34736=VERTEX_POINT('',#174659);
#34737=VERTEX_POINT('',#174661);
#34738=VERTEX_POINT('',#174663);
#34739=VERTEX_POINT('',#174665);
#34740=VERTEX_POINT('',#174667);
#42806=EDGE_CURVE('',#34623,#34624,#3041,.T.);
#42807=EDGE_CURVE('',#34625,#34623,#30123,.F.);
#42808=EDGE_CURVE('',#34626,#34625,#31187,.T.);
#42809=EDGE_CURVE('',#34624,#34626,#30124,.F.);
#42810=EDGE_CURVE('',#34627,#34628,#3042,.T.);
#42811=EDGE_CURVE('',#34623,#34627,#30125,.F.);
#42812=EDGE_CURVE('',#34628,#34624,#30126,.F.);
#42813=EDGE_CURVE('',#34629,#34628,#30127,.F.);
#42814=EDGE_CURVE('',#34630,#34629,#3043,.T.);
#42815=EDGE_CURVE('',#34627,#34630,#30128,.F.);
#42816=EDGE_CURVE('',#34631,#34632,#3044,.T.);
#42817=EDGE_CURVE('',#34630,#34631,#30129,.F.);
#42818=EDGE_CURVE('',#34632,#34629,#30130,.F.);
#42819=EDGE_CURVE('',#34633,#34634,#3045,.T.);
#42820=EDGE_CURVE('',#34631,#34633,#30131,.F.);
#42821=EDGE_CURVE('',#34635,#34632,#30132,.F.);
#42822=EDGE_CURVE('',#34634,#34635,#30133,.F.);
#42823=EDGE_CURVE('',#34636,#34637,#3046,.T.);
#42824=EDGE_CURVE('',#34633,#34636,#30134,.F.);
#42825=EDGE_CURVE('',#34637,#34634,#30135,.F.);
#42826=EDGE_CURVE('',#34638,#34639,#3047,.T.);
#42827=EDGE_CURVE('',#34640,#34638,#31188,.T.);
#42828=EDGE_CURVE('',#34636,#34640,#30136,.F.);
#42829=EDGE_CURVE('',#34639,#34637,#30137,.F.);
#42830=EDGE_CURVE('',#34641,#34642,#3048,.T.);
#42831=EDGE_CURVE('',#34643,#34641,#30138,.F.);
#42832=EDGE_CURVE('',#34644,#34643,#31189,.T.);
#42833=EDGE_CURVE('',#34642,#34644,#30139,.F.);
#42834=EDGE_CURVE('',#34645,#34646,#3049,.T.);
#42835=EDGE_CURVE('',#34641,#34645,#30140,.F.);
#42836=EDGE_CURVE('',#34646,#34642,#30141,.F.);
#42837=EDGE_CURVE('',#34647,#34648,#3050,.T.);
#42838=EDGE_CURVE('',#34645,#34647,#30142,.F.);
#42839=EDGE_CURVE('',#34648,#34646,#30143,.F.);
#42840=EDGE_CURVE('',#34649,#34650,#3051,.T.);
#42841=EDGE_CURVE('',#34651,#34649,#30144,.F.);
#42842=EDGE_CURVE('',#34647,#34651,#30145,.F.);
#42843=EDGE_CURVE('',#34652,#34648,#30146,.F.);
#42844=EDGE_CURVE('',#34650,#34652,#30147,.F.);
#42845=EDGE_CURVE('',#34653,#34654,#3052,.T.);
#42846=EDGE_CURVE('',#34649,#34653,#30148,.F.);
#42847=EDGE_CURVE('',#34654,#34650,#30149,.F.);
#42848=EDGE_CURVE('',#34655,#34656,#3053,.T.);
#42849=EDGE_CURVE('',#34653,#34655,#30150,.F.);
#42850=EDGE_CURVE('',#34656,#34654,#30151,.F.);
#42851=EDGE_CURVE('',#34657,#34658,#3054,.T.);
#42852=EDGE_CURVE('',#34655,#34657,#30152,.F.);
#42853=EDGE_CURVE('',#34658,#34656,#30153,.F.);
#42854=EDGE_CURVE('',#34659,#34660,#3055,.T.);
#42855=EDGE_CURVE('',#34644,#34659,#30154,.F.);
#42856=EDGE_CURVE('',#34660,#34644,#31190,.T.);
#42857=EDGE_CURVE('',#34661,#34662,#3056,.T.);
#42858=EDGE_CURVE('',#34663,#34661,#30155,.F.);
#42859=EDGE_CURVE('',#34663,#34664,#31191,.T.);
#42860=EDGE_CURVE('',#34662,#34664,#30156,.F.);
#42861=EDGE_CURVE('',#34665,#34666,#3057,.T.);
#42862=EDGE_CURVE('',#34661,#34665,#30157,.F.);
#42863=EDGE_CURVE('',#34666,#34662,#30158,.F.);
#42864=EDGE_CURVE('',#34667,#34668,#3058,.T.);
#42865=EDGE_CURVE('',#34665,#34667,#30159,.F.);
#42866=EDGE_CURVE('',#34668,#34666,#30160,.F.);
#42867=EDGE_CURVE('',#34669,#34670,#3059,.T.);
#42868=EDGE_CURVE('',#34667,#34669,#30161,.F.);
#42869=EDGE_CURVE('',#34670,#34668,#30162,.F.);
#42870=EDGE_CURVE('',#34671,#34672,#3060,.T.);
#42871=EDGE_CURVE('',#34669,#34671,#30163,.F.);
#42872=EDGE_CURVE('',#34672,#34670,#30164,.F.);
#42873=EDGE_CURVE('',#34673,#34674,#3061,.T.);
#42874=EDGE_CURVE('',#34675,#34673,#30165,.F.);
#42875=EDGE_CURVE('',#34675,#34676,#31192,.T.);
#42876=EDGE_CURVE('',#34674,#34676,#30166,.F.);
#42877=EDGE_CURVE('',#34677,#34678,#3062,.T.);
#42878=EDGE_CURVE('',#34673,#34677,#30167,.F.);
#42879=EDGE_CURVE('',#34678,#34674,#30168,.F.);
#42880=EDGE_CURVE('',#34679,#34680,#3063,.T.);
#42881=EDGE_CURVE('',#34677,#34679,#30169,.F.);
#42882=EDGE_CURVE('',#34680,#34678,#30170,.F.);
#42883=EDGE_CURVE('',#34681,#34682,#3064,.T.);
#42884=EDGE_CURVE('',#34679,#34681,#30171,.F.);
#42885=EDGE_CURVE('',#34682,#34680,#30172,.F.);
#42886=EDGE_CURVE('',#34683,#34682,#30173,.F.);
#42887=EDGE_CURVE('',#34684,#34683,#3065,.T.);
#42888=EDGE_CURVE('',#34681,#34684,#30174,.F.);
#42889=EDGE_CURVE('',#34685,#34686,#3066,.T.);
#42890=EDGE_CURVE('',#34684,#34685,#30175,.F.);
#42891=EDGE_CURVE('',#34686,#34683,#30176,.F.);
#42892=EDGE_CURVE('',#34687,#34688,#1770,.T.);
#42893=EDGE_CURVE('',#34688,#34689,#1771,.T.);
#42894=EDGE_CURVE('',#34689,#34690,#1772,.T.);
#42895=EDGE_CURVE('',#34690,#34691,#3067,.T.);
#42896=EDGE_CURVE('',#34691,#34691,#31193,.T.);
#42897=EDGE_CURVE('',#34690,#34692,#1773,.T.);
#42898=EDGE_CURVE('',#34692,#34693,#1774,.T.);
#42899=EDGE_CURVE('',#34693,#34687,#1775,.T.);
#42900=EDGE_CURVE('',#34694,#34686,#30177,.F.);
#42901=EDGE_CURVE('',#34694,#34695,#31194,.T.);
#42902=EDGE_CURVE('',#34685,#34695,#30178,.F.);
#42903=EDGE_CURVE('',#34696,#34696,#31195,.T.);
#42904=EDGE_CURVE('',#34696,#34697,#3068,.T.);
#42905=EDGE_CURVE('',#34697,#34698,#31196,.T.);
#42906=EDGE_CURVE('',#34698,#34697,#31197,.T.);
#42907=EDGE_CURVE('',#34699,#34699,#31198,.T.);
#42908=EDGE_CURVE('',#34699,#34700,#3069,.T.);
#42909=EDGE_CURVE('',#34700,#34700,#31199,.T.);
#42910=EDGE_CURVE('',#34701,#34701,#31200,.T.);
#42911=EDGE_CURVE('',#34701,#34702,#3070,.T.);
#42912=EDGE_CURVE('',#34702,#34702,#31201,.T.);
#42913=EDGE_CURVE('',#34703,#34672,#30179,.F.);
#42914=EDGE_CURVE('',#34703,#34704,#31202,.T.);
#42915=EDGE_CURVE('',#34671,#34704,#30180,.F.);
#42916=EDGE_CURVE('',#34638,#34705,#31203,.T.);
#42917=EDGE_CURVE('',#34695,#34705,#30181,.T.);
#42918=EDGE_CURVE('',#34706,#34694,#30182,.F.);
#42919=EDGE_CURVE('',#34706,#34698,#3071,.T.);
#42920=EDGE_CURVE('',#34640,#34706,#30183,.F.);
#42921=EDGE_CURVE('',#34707,#34708,#30184,.F.);
#42922=EDGE_CURVE('',#34707,#34709,#31204,.T.);
#42923=EDGE_CURVE('',#34664,#34709,#31205,.T.);
#42924=EDGE_CURVE('',#34708,#34663,#30185,.F.);
#42925=EDGE_CURVE('',#34708,#34701,#3072,.T.);
#42926=EDGE_CURVE('',#34710,#34711,#31206,.T.);
#42927=EDGE_CURVE('',#34711,#34712,#3073,.T.);
#42928=EDGE_CURVE('',#34712,#34712,#31207,.T.);
#42929=EDGE_CURVE('',#34711,#34710,#31208,.T.);
#42930=EDGE_CURVE('',#34713,#34713,#31209,.T.);
#42931=EDGE_CURVE('',#34713,#34714,#3074,.T.);
#42932=EDGE_CURVE('',#34714,#34714,#31210,.T.);
#42933=EDGE_CURVE('',#34715,#34715,#31211,.T.);
#42934=EDGE_CURVE('',#34715,#34713,#31212,.T.);
#42935=EDGE_CURVE('',#34710,#34716,#31213,.T.);
#42936=EDGE_CURVE('',#34716,#34716,#31214,.T.);
#42937=EDGE_CURVE('',#34717,#34718,#31215,.T.);
#42938=EDGE_CURVE('',#34717,#34719,#3075,.T.);
#42939=EDGE_CURVE('',#34720,#34719,#31216,.T.);
#42940=EDGE_CURVE('',#34718,#34720,#3076,.T.);
#42941=EDGE_CURVE('',#34643,#34660,#31217,.T.);
#42942=EDGE_CURVE('',#34704,#34643,#30186,.F.);
#42943=EDGE_CURVE('',#34659,#34703,#30187,.F.);
#42944=EDGE_CURVE('',#34626,#34721,#30188,.F.);
#42945=EDGE_CURVE('',#34676,#34625,#30189,.T.);
#42946=EDGE_CURVE('',#34721,#34675,#30190,.F.);
#42947=EDGE_CURVE('',#34721,#34722,#3077,.T.);
#42948=EDGE_CURVE('',#34722,#34722,#31218,.T.);
#42949=EDGE_CURVE('',#34709,#34658,#30191,.F.);
#42950=EDGE_CURVE('',#34657,#34707,#30192,.F.);
#42951=EDGE_CURVE('',#34705,#34639,#30193,.F.);
#42952=EDGE_CURVE('',#34723,#34717,#3078,.T.);
#42953=EDGE_CURVE('',#34723,#34724,#3079,.T.);
#42954=EDGE_CURVE('',#34719,#34724,#3080,.T.);
#42955=EDGE_CURVE('',#34725,#34723,#3081,.T.);
#42956=EDGE_CURVE('',#34725,#34726,#3082,.T.);
#42957=EDGE_CURVE('',#34724,#34726,#3083,.T.);
#42958=EDGE_CURVE('',#34727,#34725,#3084,.T.);
#42959=EDGE_CURVE('',#34727,#34728,#3085,.T.);
#42960=EDGE_CURVE('',#34726,#34728,#3086,.T.);
#42961=EDGE_CURVE('',#34729,#34727,#31219,.T.);
#42962=EDGE_CURVE('',#34729,#34730,#3087,.T.);
#42963=EDGE_CURVE('',#34728,#34730,#31220,.T.);
#42964=EDGE_CURVE('',#34731,#34729,#3088,.T.);
#42965=EDGE_CURVE('',#34731,#34732,#3089,.T.);
#42966=EDGE_CURVE('',#34730,#34732,#3090,.T.);
#42967=EDGE_CURVE('',#34733,#34731,#3091,.T.);
#42968=EDGE_CURVE('',#34733,#34734,#3092,.T.);
#42969=EDGE_CURVE('',#34732,#34734,#3093,.T.);
#42970=EDGE_CURVE('',#34718,#34733,#3094,.T.);
#42971=EDGE_CURVE('',#34734,#34720,#3095,.T.);
#42972=EDGE_CURVE('',#34735,#34736,#3096,.T.);
#42973=EDGE_CURVE('',#34737,#34735,#3097,.T.);
#42974=EDGE_CURVE('',#34738,#34737,#3098,.T.);
#42975=EDGE_CURVE('',#34739,#34738,#3099,.T.);
#42976=EDGE_CURVE('',#34740,#34739,#3100,.T.);
#42977=EDGE_CURVE('',#34736,#34740,#3101,.T.);
#42978=EDGE_CURVE('',#34738,#34690,#3102,.T.);
#42979=EDGE_CURVE('',#34739,#34689,#3103,.T.);
#42980=EDGE_CURVE('',#34740,#34688,#3104,.T.);
#42981=EDGE_CURVE('',#34736,#34687,#3105,.T.);
#42982=EDGE_CURVE('',#34735,#34693,#3106,.T.);
#42983=EDGE_CURVE('',#34737,#34692,#3107,.T.);
#55947=ORIENTED_EDGE('',*,*,#42806,.F.);
#55948=ORIENTED_EDGE('',*,*,#42807,.F.);
#55949=ORIENTED_EDGE('',*,*,#42808,.F.);
#55950=ORIENTED_EDGE('',*,*,#42809,.F.);
#55951=ORIENTED_EDGE('',*,*,#42810,.F.);
#55952=ORIENTED_EDGE('',*,*,#42811,.F.);
#55953=ORIENTED_EDGE('',*,*,#42806,.T.);
#55954=ORIENTED_EDGE('',*,*,#42812,.F.);
#55955=ORIENTED_EDGE('',*,*,#42810,.T.);
#55956=ORIENTED_EDGE('',*,*,#42813,.F.);
#55957=ORIENTED_EDGE('',*,*,#42814,.F.);
#55958=ORIENTED_EDGE('',*,*,#42815,.F.);
#55959=ORIENTED_EDGE('',*,*,#42816,.F.);
#55960=ORIENTED_EDGE('',*,*,#42817,.F.);
#55961=ORIENTED_EDGE('',*,*,#42814,.T.);
#55962=ORIENTED_EDGE('',*,*,#42818,.F.);
#55963=ORIENTED_EDGE('',*,*,#42819,.F.);
#55964=ORIENTED_EDGE('',*,*,#42820,.F.);
#55965=ORIENTED_EDGE('',*,*,#42816,.T.);
#55966=ORIENTED_EDGE('',*,*,#42821,.F.);
#55967=ORIENTED_EDGE('',*,*,#42822,.F.);
#55968=ORIENTED_EDGE('',*,*,#42823,.F.);
#55969=ORIENTED_EDGE('',*,*,#42824,.F.);
#55970=ORIENTED_EDGE('',*,*,#42819,.T.);
#55971=ORIENTED_EDGE('',*,*,#42825,.F.);
#55972=ORIENTED_EDGE('',*,*,#42826,.F.);
#55973=ORIENTED_EDGE('',*,*,#42827,.F.);
#55974=ORIENTED_EDGE('',*,*,#42828,.F.);
#55975=ORIENTED_EDGE('',*,*,#42823,.T.);
#55976=ORIENTED_EDGE('',*,*,#42829,.F.);
#55977=ORIENTED_EDGE('',*,*,#42830,.F.);
#55978=ORIENTED_EDGE('',*,*,#42831,.F.);
#55979=ORIENTED_EDGE('',*,*,#42832,.F.);
#55980=ORIENTED_EDGE('',*,*,#42833,.F.);
#55981=ORIENTED_EDGE('',*,*,#42834,.F.);
#55982=ORIENTED_EDGE('',*,*,#42835,.F.);
#55983=ORIENTED_EDGE('',*,*,#42830,.T.);
#55984=ORIENTED_EDGE('',*,*,#42836,.F.);
#55985=ORIENTED_EDGE('',*,*,#42837,.F.);
#55986=ORIENTED_EDGE('',*,*,#42838,.F.);
#55987=ORIENTED_EDGE('',*,*,#42834,.T.);
#55988=ORIENTED_EDGE('',*,*,#42839,.F.);
#55989=ORIENTED_EDGE('',*,*,#42840,.F.);
#55990=ORIENTED_EDGE('',*,*,#42841,.F.);
#55991=ORIENTED_EDGE('',*,*,#42842,.F.);
#55992=ORIENTED_EDGE('',*,*,#42837,.T.);
#55993=ORIENTED_EDGE('',*,*,#42843,.F.);
#55994=ORIENTED_EDGE('',*,*,#42844,.F.);
#55995=ORIENTED_EDGE('',*,*,#42845,.F.);
#55996=ORIENTED_EDGE('',*,*,#42846,.F.);
#55997=ORIENTED_EDGE('',*,*,#42840,.T.);
#55998=ORIENTED_EDGE('',*,*,#42847,.F.);
#55999=ORIENTED_EDGE('',*,*,#42848,.F.);
#56000=ORIENTED_EDGE('',*,*,#42849,.F.);
#56001=ORIENTED_EDGE('',*,*,#42845,.T.);
#56002=ORIENTED_EDGE('',*,*,#42850,.F.);
#56003=ORIENTED_EDGE('',*,*,#42851,.F.);
#56004=ORIENTED_EDGE('',*,*,#42852,.F.);
#56005=ORIENTED_EDGE('',*,*,#42848,.T.);
#56006=ORIENTED_EDGE('',*,*,#42853,.F.);
#56007=ORIENTED_EDGE('',*,*,#42854,.F.);
#56008=ORIENTED_EDGE('',*,*,#42855,.F.);
#56009=ORIENTED_EDGE('',*,*,#42856,.F.);
#56010=ORIENTED_EDGE('',*,*,#42857,.F.);
#56011=ORIENTED_EDGE('',*,*,#42858,.F.);
#56012=ORIENTED_EDGE('',*,*,#42859,.T.);
#56013=ORIENTED_EDGE('',*,*,#42860,.F.);
#56014=ORIENTED_EDGE('',*,*,#42861,.F.);
#56015=ORIENTED_EDGE('',*,*,#42862,.F.);
#56016=ORIENTED_EDGE('',*,*,#42857,.T.);
#56017=ORIENTED_EDGE('',*,*,#42863,.F.);
#56018=ORIENTED_EDGE('',*,*,#42864,.F.);
#56019=ORIENTED_EDGE('',*,*,#42865,.F.);
#56020=ORIENTED_EDGE('',*,*,#42861,.T.);
#56021=ORIENTED_EDGE('',*,*,#42866,.F.);
#56022=ORIENTED_EDGE('',*,*,#42867,.F.);
#56023=ORIENTED_EDGE('',*,*,#42868,.F.);
#56024=ORIENTED_EDGE('',*,*,#42864,.T.);
#56025=ORIENTED_EDGE('',*,*,#42869,.F.);
#56026=ORIENTED_EDGE('',*,*,#42870,.F.);
#56027=ORIENTED_EDGE('',*,*,#42871,.F.);
#56028=ORIENTED_EDGE('',*,*,#42867,.T.);
#56029=ORIENTED_EDGE('',*,*,#42872,.F.);
#56030=ORIENTED_EDGE('',*,*,#42873,.F.);
#56031=ORIENTED_EDGE('',*,*,#42874,.F.);
#56032=ORIENTED_EDGE('',*,*,#42875,.T.);
#56033=ORIENTED_EDGE('',*,*,#42876,.F.);
#56034=ORIENTED_EDGE('',*,*,#42877,.F.);
#56035=ORIENTED_EDGE('',*,*,#42878,.F.);
#56036=ORIENTED_EDGE('',*,*,#42873,.T.);
#56037=ORIENTED_EDGE('',*,*,#42879,.F.);
#56038=ORIENTED_EDGE('',*,*,#42880,.F.);
#56039=ORIENTED_EDGE('',*,*,#42881,.F.);
#56040=ORIENTED_EDGE('',*,*,#42877,.T.);
#56041=ORIENTED_EDGE('',*,*,#42882,.F.);
#56042=ORIENTED_EDGE('',*,*,#42883,.F.);
#56043=ORIENTED_EDGE('',*,*,#42884,.F.);
#56044=ORIENTED_EDGE('',*,*,#42880,.T.);
#56045=ORIENTED_EDGE('',*,*,#42885,.F.);
#56046=ORIENTED_EDGE('',*,*,#42886,.F.);
#56047=ORIENTED_EDGE('',*,*,#42887,.F.);
#56048=ORIENTED_EDGE('',*,*,#42888,.F.);
#56049=ORIENTED_EDGE('',*,*,#42883,.T.);
#56050=ORIENTED_EDGE('',*,*,#42889,.F.);
#56051=ORIENTED_EDGE('',*,*,#42890,.F.);
#56052=ORIENTED_EDGE('',*,*,#42887,.T.);
#56053=ORIENTED_EDGE('',*,*,#42891,.F.);
#56054=ORIENTED_EDGE('',*,*,#42892,.T.);
#56055=ORIENTED_EDGE('',*,*,#42893,.T.);
#56056=ORIENTED_EDGE('',*,*,#42894,.T.);
#56057=ORIENTED_EDGE('',*,*,#42895,.T.);
#56058=ORIENTED_EDGE('',*,*,#42896,.F.);
#56059=ORIENTED_EDGE('',*,*,#42895,.F.);
#56060=ORIENTED_EDGE('',*,*,#42897,.T.);
#56061=ORIENTED_EDGE('',*,*,#42898,.T.);
#56062=ORIENTED_EDGE('',*,*,#42899,.T.);
#56063=ORIENTED_EDGE('',*,*,#42889,.T.);
#56064=ORIENTED_EDGE('',*,*,#42900,.F.);
#56065=ORIENTED_EDGE('',*,*,#42901,.T.);
#56066=ORIENTED_EDGE('',*,*,#42902,.F.);
#56067=ORIENTED_EDGE('',*,*,#42903,.F.);
#56068=ORIENTED_EDGE('',*,*,#42904,.T.);
#56069=ORIENTED_EDGE('',*,*,#42905,.T.);
#56070=ORIENTED_EDGE('',*,*,#42906,.T.);
#56071=ORIENTED_EDGE('',*,*,#42904,.F.);
#56072=ORIENTED_EDGE('',*,*,#42907,.F.);
#56073=ORIENTED_EDGE('',*,*,#42908,.T.);
#56074=ORIENTED_EDGE('',*,*,#42909,.T.);
#56075=ORIENTED_EDGE('',*,*,#42908,.F.);
#56076=ORIENTED_EDGE('',*,*,#42910,.F.);
#56077=ORIENTED_EDGE('',*,*,#42911,.T.);
#56078=ORIENTED_EDGE('',*,*,#42912,.T.);
#56079=ORIENTED_EDGE('',*,*,#42911,.F.);
#56080=ORIENTED_EDGE('',*,*,#42870,.T.);
#56081=ORIENTED_EDGE('',*,*,#42913,.F.);
#56082=ORIENTED_EDGE('',*,*,#42914,.T.);
#56083=ORIENTED_EDGE('',*,*,#42915,.F.);
#56084=ORIENTED_EDGE('',*,*,#42827,.T.);
#56085=ORIENTED_EDGE('',*,*,#42916,.T.);
#56086=ORIENTED_EDGE('',*,*,#42917,.F.);
#56087=ORIENTED_EDGE('',*,*,#42901,.F.);
#56088=ORIENTED_EDGE('',*,*,#42918,.F.);
#56089=ORIENTED_EDGE('',*,*,#42919,.T.);
#56090=ORIENTED_EDGE('',*,*,#42905,.F.);
#56091=ORIENTED_EDGE('',*,*,#42906,.F.);
#56092=ORIENTED_EDGE('',*,*,#42919,.F.);
#56093=ORIENTED_EDGE('',*,*,#42920,.F.);
#56094=ORIENTED_EDGE('',*,*,#42921,.F.);
#56095=ORIENTED_EDGE('',*,*,#42922,.T.);
#56096=ORIENTED_EDGE('',*,*,#42923,.F.);
#56097=ORIENTED_EDGE('',*,*,#42859,.F.);
#56098=ORIENTED_EDGE('',*,*,#42924,.F.);
#56099=ORIENTED_EDGE('',*,*,#42925,.T.);
#56100=ORIENTED_EDGE('',*,*,#42910,.T.);
#56101=ORIENTED_EDGE('',*,*,#42925,.F.);
#56102=ORIENTED_EDGE('',*,*,#42926,.T.);
#56103=ORIENTED_EDGE('',*,*,#42927,.T.);
#56104=ORIENTED_EDGE('',*,*,#42928,.T.);
#56105=ORIENTED_EDGE('',*,*,#42927,.F.);
#56106=ORIENTED_EDGE('',*,*,#42929,.T.);
#56107=ORIENTED_EDGE('',*,*,#42930,.T.);
#56108=ORIENTED_EDGE('',*,*,#42931,.T.);
#56109=ORIENTED_EDGE('',*,*,#42932,.T.);
#56110=ORIENTED_EDGE('',*,*,#42931,.F.);
#56111=ORIENTED_EDGE('',*,*,#42933,.F.);
#56112=ORIENTED_EDGE('',*,*,#42934,.T.);
#56113=ORIENTED_EDGE('',*,*,#42930,.F.);
#56114=ORIENTED_EDGE('',*,*,#42934,.F.);
#56115=ORIENTED_EDGE('',*,*,#42926,.F.);
#56116=ORIENTED_EDGE('',*,*,#42935,.T.);
#56117=ORIENTED_EDGE('',*,*,#42936,.F.);
#56118=ORIENTED_EDGE('',*,*,#42935,.F.);
#56119=ORIENTED_EDGE('',*,*,#42929,.F.);
#56120=ORIENTED_EDGE('',*,*,#42937,.F.);
#56121=ORIENTED_EDGE('',*,*,#42938,.T.);
#56122=ORIENTED_EDGE('',*,*,#42939,.F.);
#56123=ORIENTED_EDGE('',*,*,#42940,.F.);
#56124=ORIENTED_EDGE('',*,*,#42854,.T.);
#56125=ORIENTED_EDGE('',*,*,#42941,.F.);
#56126=ORIENTED_EDGE('',*,*,#42942,.F.);
#56127=ORIENTED_EDGE('',*,*,#42914,.F.);
#56128=ORIENTED_EDGE('',*,*,#42943,.F.);
#56129=ORIENTED_EDGE('',*,*,#42944,.F.);
#56130=ORIENTED_EDGE('',*,*,#42808,.T.);
#56131=ORIENTED_EDGE('',*,*,#42945,.F.);
#56132=ORIENTED_EDGE('',*,*,#42875,.F.);
#56133=ORIENTED_EDGE('',*,*,#42946,.F.);
#56134=ORIENTED_EDGE('',*,*,#42947,.T.);
#56135=ORIENTED_EDGE('',*,*,#42948,.F.);
#56136=ORIENTED_EDGE('',*,*,#42947,.F.);
#56137=ORIENTED_EDGE('',*,*,#42851,.T.);
#56138=ORIENTED_EDGE('',*,*,#42949,.F.);
#56139=ORIENTED_EDGE('',*,*,#42922,.F.);
#56140=ORIENTED_EDGE('',*,*,#42950,.F.);
#56141=ORIENTED_EDGE('',*,*,#42826,.T.);
#56142=ORIENTED_EDGE('',*,*,#42951,.F.);
#56143=ORIENTED_EDGE('',*,*,#42916,.F.);
#56144=ORIENTED_EDGE('',*,*,#42885,.T.);
#56145=ORIENTED_EDGE('',*,*,#42882,.T.);
#56146=ORIENTED_EDGE('',*,*,#42879,.T.);
#56147=ORIENTED_EDGE('',*,*,#42876,.T.);
#56148=ORIENTED_EDGE('',*,*,#42945,.T.);
#56149=ORIENTED_EDGE('',*,*,#42807,.T.);
#56150=ORIENTED_EDGE('',*,*,#42811,.T.);
#56151=ORIENTED_EDGE('',*,*,#42815,.T.);
#56152=ORIENTED_EDGE('',*,*,#42817,.T.);
#56153=ORIENTED_EDGE('',*,*,#42820,.T.);
#56154=ORIENTED_EDGE('',*,*,#42824,.T.);
#56155=ORIENTED_EDGE('',*,*,#42828,.T.);
#56156=ORIENTED_EDGE('',*,*,#42920,.T.);
#56157=ORIENTED_EDGE('',*,*,#42918,.T.);
#56158=ORIENTED_EDGE('',*,*,#42900,.T.);
#56159=ORIENTED_EDGE('',*,*,#42891,.T.);
#56160=ORIENTED_EDGE('',*,*,#42886,.T.);
#56161=ORIENTED_EDGE('',*,*,#42917,.T.);
#56162=ORIENTED_EDGE('',*,*,#42951,.T.);
#56163=ORIENTED_EDGE('',*,*,#42829,.T.);
#56164=ORIENTED_EDGE('',*,*,#42825,.T.);
#56165=ORIENTED_EDGE('',*,*,#42822,.T.);
#56166=ORIENTED_EDGE('',*,*,#42821,.T.);
#56167=ORIENTED_EDGE('',*,*,#42818,.T.);
#56168=ORIENTED_EDGE('',*,*,#42813,.T.);
#56169=ORIENTED_EDGE('',*,*,#42812,.T.);
#56170=ORIENTED_EDGE('',*,*,#42809,.T.);
#56171=ORIENTED_EDGE('',*,*,#42944,.T.);
#56172=ORIENTED_EDGE('',*,*,#42946,.T.);
#56173=ORIENTED_EDGE('',*,*,#42874,.T.);
#56174=ORIENTED_EDGE('',*,*,#42878,.T.);
#56175=ORIENTED_EDGE('',*,*,#42881,.T.);
#56176=ORIENTED_EDGE('',*,*,#42884,.T.);
#56177=ORIENTED_EDGE('',*,*,#42888,.T.);
#56178=ORIENTED_EDGE('',*,*,#42890,.T.);
#56179=ORIENTED_EDGE('',*,*,#42902,.T.);
#56180=ORIENTED_EDGE('',*,*,#42921,.T.);
#56181=ORIENTED_EDGE('',*,*,#42924,.T.);
#56182=ORIENTED_EDGE('',*,*,#42858,.T.);
#56183=ORIENTED_EDGE('',*,*,#42862,.T.);
#56184=ORIENTED_EDGE('',*,*,#42865,.T.);
#56185=ORIENTED_EDGE('',*,*,#42868,.T.);
#56186=ORIENTED_EDGE('',*,*,#42871,.T.);
#56187=ORIENTED_EDGE('',*,*,#42915,.T.);
#56188=ORIENTED_EDGE('',*,*,#42942,.T.);
#56189=ORIENTED_EDGE('',*,*,#42831,.T.);
#56190=ORIENTED_EDGE('',*,*,#42835,.T.);
#56191=ORIENTED_EDGE('',*,*,#42838,.T.);
#56192=ORIENTED_EDGE('',*,*,#42842,.T.);
#56193=ORIENTED_EDGE('',*,*,#42841,.T.);
#56194=ORIENTED_EDGE('',*,*,#42846,.T.);
#56195=ORIENTED_EDGE('',*,*,#42849,.T.);
#56196=ORIENTED_EDGE('',*,*,#42852,.T.);
#56197=ORIENTED_EDGE('',*,*,#42950,.T.);
#56198=ORIENTED_EDGE('',*,*,#42923,.T.);
#56199=ORIENTED_EDGE('',*,*,#42949,.T.);
#56200=ORIENTED_EDGE('',*,*,#42853,.T.);
#56201=ORIENTED_EDGE('',*,*,#42850,.T.);
#56202=ORIENTED_EDGE('',*,*,#42847,.T.);
#56203=ORIENTED_EDGE('',*,*,#42844,.T.);
#56204=ORIENTED_EDGE('',*,*,#42843,.T.);
#56205=ORIENTED_EDGE('',*,*,#42839,.T.);
#56206=ORIENTED_EDGE('',*,*,#42836,.T.);
#56207=ORIENTED_EDGE('',*,*,#42833,.T.);
#56208=ORIENTED_EDGE('',*,*,#42855,.T.);
#56209=ORIENTED_EDGE('',*,*,#42943,.T.);
#56210=ORIENTED_EDGE('',*,*,#42913,.T.);
#56211=ORIENTED_EDGE('',*,*,#42872,.T.);
#56212=ORIENTED_EDGE('',*,*,#42869,.T.);
#56213=ORIENTED_EDGE('',*,*,#42866,.T.);
#56214=ORIENTED_EDGE('',*,*,#42863,.T.);
#56215=ORIENTED_EDGE('',*,*,#42860,.T.);
#56216=ORIENTED_EDGE('',*,*,#42938,.F.);
#56217=ORIENTED_EDGE('',*,*,#42952,.F.);
#56218=ORIENTED_EDGE('',*,*,#42953,.T.);
#56219=ORIENTED_EDGE('',*,*,#42954,.F.);
#56220=ORIENTED_EDGE('',*,*,#42953,.F.);
#56221=ORIENTED_EDGE('',*,*,#42955,.F.);
#56222=ORIENTED_EDGE('',*,*,#42956,.T.);
#56223=ORIENTED_EDGE('',*,*,#42957,.F.);
#56224=ORIENTED_EDGE('',*,*,#42956,.F.);
#56225=ORIENTED_EDGE('',*,*,#42958,.F.);
#56226=ORIENTED_EDGE('',*,*,#42959,.T.);
#56227=ORIENTED_EDGE('',*,*,#42960,.F.);
#56228=ORIENTED_EDGE('',*,*,#42959,.F.);
#56229=ORIENTED_EDGE('',*,*,#42961,.F.);
#56230=ORIENTED_EDGE('',*,*,#42962,.T.);
#56231=ORIENTED_EDGE('',*,*,#42963,.F.);
#56232=ORIENTED_EDGE('',*,*,#42962,.F.);
#56233=ORIENTED_EDGE('',*,*,#42964,.F.);
#56234=ORIENTED_EDGE('',*,*,#42965,.T.);
#56235=ORIENTED_EDGE('',*,*,#42966,.F.);
#56236=ORIENTED_EDGE('',*,*,#42965,.F.);
#56237=ORIENTED_EDGE('',*,*,#42967,.F.);
#56238=ORIENTED_EDGE('',*,*,#42968,.T.);
#56239=ORIENTED_EDGE('',*,*,#42969,.F.);
#56240=ORIENTED_EDGE('',*,*,#42968,.F.);
#56241=ORIENTED_EDGE('',*,*,#42970,.F.);
#56242=ORIENTED_EDGE('',*,*,#42940,.T.);
#56243=ORIENTED_EDGE('',*,*,#42971,.F.);
#56244=ORIENTED_EDGE('',*,*,#42932,.F.);
#56245=ORIENTED_EDGE('',*,*,#42937,.T.);
#56246=ORIENTED_EDGE('',*,*,#42970,.T.);
#56247=ORIENTED_EDGE('',*,*,#42967,.T.);
#56248=ORIENTED_EDGE('',*,*,#42964,.T.);
#56249=ORIENTED_EDGE('',*,*,#42961,.T.);
#56250=ORIENTED_EDGE('',*,*,#42958,.T.);
#56251=ORIENTED_EDGE('',*,*,#42955,.T.);
#56252=ORIENTED_EDGE('',*,*,#42952,.T.);
#56253=ORIENTED_EDGE('',*,*,#42928,.F.);
#56254=ORIENTED_EDGE('',*,*,#42933,.T.);
#56255=ORIENTED_EDGE('',*,*,#42972,.F.);
#56256=ORIENTED_EDGE('',*,*,#42973,.F.);
#56257=ORIENTED_EDGE('',*,*,#42974,.F.);
#56258=ORIENTED_EDGE('',*,*,#42975,.F.);
#56259=ORIENTED_EDGE('',*,*,#42976,.F.);
#56260=ORIENTED_EDGE('',*,*,#42977,.F.);
#56261=ORIENTED_EDGE('',*,*,#42969,.T.);
#56262=ORIENTED_EDGE('',*,*,#42971,.T.);
#56263=ORIENTED_EDGE('',*,*,#42939,.T.);
#56264=ORIENTED_EDGE('',*,*,#42954,.T.);
#56265=ORIENTED_EDGE('',*,*,#42957,.T.);
#56266=ORIENTED_EDGE('',*,*,#42960,.T.);
#56267=ORIENTED_EDGE('',*,*,#42963,.T.);
#56268=ORIENTED_EDGE('',*,*,#42966,.T.);
#56269=ORIENTED_EDGE('',*,*,#42975,.T.);
#56270=ORIENTED_EDGE('',*,*,#42978,.T.);
#56271=ORIENTED_EDGE('',*,*,#42894,.F.);
#56272=ORIENTED_EDGE('',*,*,#42979,.F.);
#56273=ORIENTED_EDGE('',*,*,#42976,.T.);
#56274=ORIENTED_EDGE('',*,*,#42979,.T.);
#56275=ORIENTED_EDGE('',*,*,#42893,.F.);
#56276=ORIENTED_EDGE('',*,*,#42980,.F.);
#56277=ORIENTED_EDGE('',*,*,#42977,.T.);
#56278=ORIENTED_EDGE('',*,*,#42980,.T.);
#56279=ORIENTED_EDGE('',*,*,#42892,.F.);
#56280=ORIENTED_EDGE('',*,*,#42981,.F.);
#56281=ORIENTED_EDGE('',*,*,#42972,.T.);
#56282=ORIENTED_EDGE('',*,*,#42981,.T.);
#56283=ORIENTED_EDGE('',*,*,#42899,.F.);
#56284=ORIENTED_EDGE('',*,*,#42982,.F.);
#56285=ORIENTED_EDGE('',*,*,#42973,.T.);
#56286=ORIENTED_EDGE('',*,*,#42982,.T.);
#56287=ORIENTED_EDGE('',*,*,#42898,.F.);
#56288=ORIENTED_EDGE('',*,*,#42983,.F.);
#56289=ORIENTED_EDGE('',*,*,#42978,.F.);
#56290=ORIENTED_EDGE('',*,*,#42974,.T.);
#56291=ORIENTED_EDGE('',*,*,#42983,.T.);
#56292=ORIENTED_EDGE('',*,*,#42897,.F.);
#56293=ORIENTED_EDGE('',*,*,#42832,.T.);
#56294=ORIENTED_EDGE('',*,*,#42941,.T.);
#56295=ORIENTED_EDGE('',*,*,#42856,.T.);
#56296=ORIENTED_EDGE('',*,*,#42936,.T.);
#56297=ORIENTED_EDGE('',*,*,#42909,.F.);
#56298=ORIENTED_EDGE('',*,*,#42903,.T.);
#56299=ORIENTED_EDGE('',*,*,#42907,.T.);
#56300=ORIENTED_EDGE('',*,*,#42912,.F.);
#56301=ORIENTED_EDGE('',*,*,#42948,.T.);
#56302=ORIENTED_EDGE('',*,*,#42896,.T.);
#76031=ADVANCED_FACE('',(#20601),#2170,.T.);
#76032=ADVANCED_FACE('',(#20602),#2171,.T.);
#76033=ADVANCED_FACE('',(#20603),#2172,.T.);
#76034=ADVANCED_FACE('',(#20604),#2173,.T.);
#76035=ADVANCED_FACE('',(#20605),#2174,.T.);
#76036=ADVANCED_FACE('',(#20606),#2175,.T.);
#76037=ADVANCED_FACE('',(#20607),#2176,.T.);
#76038=ADVANCED_FACE('',(#20608),#2177,.T.);
#76039=ADVANCED_FACE('',(#20609),#2178,.T.);
#76040=ADVANCED_FACE('',(#20610),#2179,.T.);
#76041=ADVANCED_FACE('',(#20611),#2180,.T.);
#76042=ADVANCED_FACE('',(#20612),#2181,.T.);
#76043=ADVANCED_FACE('',(#20613),#2182,.T.);
#76044=ADVANCED_FACE('',(#20614),#2183,.T.);
#76045=ADVANCED_FACE('',(#20615),#1933,.T.);
#76046=ADVANCED_FACE('',(#20616),#2184,.T.);
#76047=ADVANCED_FACE('',(#20617),#2185,.T.);
#76048=ADVANCED_FACE('',(#20618),#2186,.T.);
#76049=ADVANCED_FACE('',(#20619),#2187,.T.);
#76050=ADVANCED_FACE('',(#20620),#2188,.T.);
#76051=ADVANCED_FACE('',(#20621),#2189,.T.);
#76052=ADVANCED_FACE('',(#20622),#2190,.T.);
#76053=ADVANCED_FACE('',(#20623),#2191,.T.);
#76054=ADVANCED_FACE('',(#20624),#2192,.T.);
#76055=ADVANCED_FACE('',(#20625),#2193,.T.);
#76056=ADVANCED_FACE('',(#20626),#2194,.T.);
#76057=ADVANCED_FACE('',(#20627),#1934,.F.);
#76058=ADVANCED_FACE('',(#20628),#2195,.T.);
#76059=ADVANCED_FACE('',(#20629),#2196,.T.);
#76060=ADVANCED_FACE('',(#20630),#2197,.T.);
#76061=ADVANCED_FACE('',(#20631),#2198,.T.);
#76062=ADVANCED_FACE('',(#20632),#2199,.T.);
#76063=ADVANCED_FACE('',(#20633),#1935,.T.);
#76064=ADVANCED_FACE('',(#20634),#1936,.T.);
#76065=ADVANCED_FACE('',(#20635),#2200,.F.);
#76066=ADVANCED_FACE('',(#20636),#2201,.F.);
#76067=ADVANCED_FACE('',(#20637),#1886,.T.);
#76068=ADVANCED_FACE('',(#20638),#1887,.T.);
#76069=ADVANCED_FACE('',(#20639),#2202,.F.);
#76070=ADVANCED_FACE('',(#20640),#1937,.T.);
#76071=ADVANCED_FACE('',(#20641),#1938,.T.);
#76072=ADVANCED_FACE('',(#20642),#2203,.T.);
#76073=ADVANCED_FACE('',(#20643),#2204,.T.);
#76074=ADVANCED_FACE('',(#20644),#179,.F.);
#76075=ADVANCED_FACE('',(#20645),#180,.F.);
#76076=ADVANCED_FACE('',(#20646),#181,.F.);
#76077=ADVANCED_FACE('',(#20647),#182,.F.);
#76078=ADVANCED_FACE('',(#20648),#16943,.F.);
#76079=ADVANCED_FACE('',(#20649),#16944,.F.);
#76080=ADVANCED_FACE('',(#20650),#16945,.F.);
#76081=ADVANCED_FACE('',(#20651),#2205,.F.);
#76082=ADVANCED_FACE('',(#20652),#16946,.F.);
#76083=ADVANCED_FACE('',(#20653),#16947,.F.);
#76084=ADVANCED_FACE('',(#20654),#16948,.F.);
#76085=ADVANCED_FACE('',(#20655,#275),#16949,.F.);
#76086=ADVANCED_FACE('',(#20656,#276),#16950,.F.);
#76087=ADVANCED_FACE('',(#20657,#277),#16951,.F.);
#76088=ADVANCED_FACE('',(#20658),#16952,.T.);
#76089=ADVANCED_FACE('',(#20659),#16953,.T.);
#76090=ADVANCED_FACE('',(#20660),#16954,.T.);
#76091=ADVANCED_FACE('',(#20661),#16955,.T.);
#76092=ADVANCED_FACE('',(#20662),#16956,.T.);
#76093=ADVANCED_FACE('',(#20663),#16957,.T.);
#76094=ADVANCED_FACE('',(#20664,#278),#16958,.T.);
#76095=ADVANCED_FACE('',(#20665,#279),#16959,.T.);
#76096=ADVANCED_FACE('',(#20666,#280),#16960,.T.);
#76097=ADVANCED_FACE('',(#20667,#281),#16961,.T.);
#79324=CLOSED_SHELL('',(#76031,#76032,#76033,#76034,#76035,#76036,#76037,
#76038,#76039,#76040,#76041,#76042,#76043,#76044,#76045,#76046,#76047,#76048,
#76049,#76050,#76051,#76052,#76053,#76054,#76055,#76056,#76057,#76058,#76059,
#76060,#76061,#76062,#76063,#76064,#76065,#76066,#76067,#76068,#76069,#76070,
#76071,#76072,#76073,#76074,#76075,#76076,#76077,#76078,#76079,#76080,#76081,
#76082,#76083,#76084,#76085,#76086,#76087,#76088,#76089,#76090,#76091,#76092,
#76093,#76094,#76095,#76096,#76097));
#80522=AXIS2_PLACEMENT_3D('',#161937,#88584,#88585);
#80523=AXIS2_PLACEMENT_3D('',#161938,#88586,#88587);
#80524=AXIS2_PLACEMENT_3D('',#162146,#88589,#88590);
#80525=AXIS2_PLACEMENT_3D('',#162327,#88591,#88592);
#80526=AXIS2_PLACEMENT_3D('',#162745,#88594,#88595);
#80527=AXIS2_PLACEMENT_3D('',#163163,#88597,#88598);
#80528=AXIS2_PLACEMENT_3D('',#163569,#88600,#88601);
#80529=AXIS2_PLACEMENT_3D('',#163990,#88603,#88604);
#80530=AXIS2_PLACEMENT_3D('',#164418,#88606,#88607);
#80531=AXIS2_PLACEMENT_3D('',#164423,#88609,#88610);
#80532=AXIS2_PLACEMENT_3D('',#164830,#88611,#88612);
#80533=AXIS2_PLACEMENT_3D('',#164974,#88614,#88615);
#80534=AXIS2_PLACEMENT_3D('',#165103,#88616,#88617);
#80535=AXIS2_PLACEMENT_3D('',#165633,#88619,#88620);
#80536=AXIS2_PLACEMENT_3D('',#166147,#88622,#88623);
#80537=AXIS2_PLACEMENT_3D('',#166683,#88625,#88626);
#80538=AXIS2_PLACEMENT_3D('',#167207,#88628,#88629);
#80539=AXIS2_PLACEMENT_3D('',#167727,#88631,#88632);
#80540=AXIS2_PLACEMENT_3D('',#168253,#88634,#88635);
#80541=AXIS2_PLACEMENT_3D('',#168279,#88637,#88638);
#80542=AXIS2_PLACEMENT_3D('',#168280,#88639,#88640);
#80543=AXIS2_PLACEMENT_3D('',#168456,#88642,#88643);
#80544=AXIS2_PLACEMENT_3D('',#168627,#88644,#88645);
#80545=AXIS2_PLACEMENT_3D('',#169155,#88647,#88648);
#80546=AXIS2_PLACEMENT_3D('',#169671,#88650,#88651);
#80547=AXIS2_PLACEMENT_3D('',#170189,#88653,#88654);
#80548=AXIS2_PLACEMENT_3D('',#170715,#88656,#88657);
#80549=AXIS2_PLACEMENT_3D('',#170875,#88659,#88660);
#80550=AXIS2_PLACEMENT_3D('',#171014,#88661,#88662);
#80551=AXIS2_PLACEMENT_3D('',#171444,#88664,#88665);
#80552=AXIS2_PLACEMENT_3D('',#171888,#88667,#88668);
#80553=AXIS2_PLACEMENT_3D('',#172332,#88670,#88671);
#80554=AXIS2_PLACEMENT_3D('',#172766,#88673,#88674);
#80555=AXIS2_PLACEMENT_3D('',#173202,#88676,#88677);
#80556=AXIS2_PLACEMENT_3D('',#173218,#88679,#88680);
#80557=AXIS2_PLACEMENT_3D('',#173230,#88681,#88682);
#80558=AXIS2_PLACEMENT_3D('',#173273,#88683,#88684);
#80559=AXIS2_PLACEMENT_3D('',#173292,#88685,#88686);
#80560=AXIS2_PLACEMENT_3D('',#173294,#88687,#88688);
#80561=AXIS2_PLACEMENT_3D('',#173298,#88690,#88691);
#80562=AXIS2_PLACEMENT_3D('',#173299,#88692,#88693);
#80563=AXIS2_PLACEMENT_3D('',#173300,#88694,#88695);
#80564=AXIS2_PLACEMENT_3D('',#173302,#88696,#88697);
#80565=AXIS2_PLACEMENT_3D('',#173305,#88699,#88700);
#80566=AXIS2_PLACEMENT_3D('',#173306,#88701,#88702);
#80567=AXIS2_PLACEMENT_3D('',#173308,#88703,#88704);
#80568=AXIS2_PLACEMENT_3D('',#173311,#88706,#88707);
#80569=AXIS2_PLACEMENT_3D('',#173312,#88708,#88709);
#80570=AXIS2_PLACEMENT_3D('',#173513,#88710,#88711);
#80571=AXIS2_PLACEMENT_3D('',#173700,#88712,#88713);
#80572=AXIS2_PLACEMENT_3D('',#173702,#88714,#88715);
#80573=AXIS2_PLACEMENT_3D('',#173749,#88717,#88718);
#80574=AXIS2_PLACEMENT_3D('',#173777,#88719,#88720);
#80575=AXIS2_PLACEMENT_3D('',#173778,#88721,#88722);
#80576=AXIS2_PLACEMENT_3D('',#173794,#88724,#88725);
#80577=AXIS2_PLACEMENT_3D('',#173797,#88726,#88727);
#80578=AXIS2_PLACEMENT_3D('',#173800,#88729,#88730);
#80579=AXIS2_PLACEMENT_3D('',#173801,#88731,#88732);
#80580=AXIS2_PLACEMENT_3D('',#173802,#88733,#88734);
#80581=AXIS2_PLACEMENT_3D('',#173804,#88735,#88736);
#80582=AXIS2_PLACEMENT_3D('',#173807,#88738,#88739);
#80583=AXIS2_PLACEMENT_3D('',#173808,#88740,#88741);
#80584=AXIS2_PLACEMENT_3D('',#173810,#88742,#88743);
#80585=AXIS2_PLACEMENT_3D('',#173811,#88744,#88745);
#80586=AXIS2_PLACEMENT_3D('',#173812,#88746,#88747);
#80587=AXIS2_PLACEMENT_3D('',#173814,#88748,#88749);
#80588=AXIS2_PLACEMENT_3D('',#173815,#88750,#88751);
#80589=AXIS2_PLACEMENT_3D('',#173816,#88752,#88753);
#80590=AXIS2_PLACEMENT_3D('',#173819,#88754,#88755);
#80591=AXIS2_PLACEMENT_3D('',#173823,#88757,#88758);
#80592=AXIS2_PLACEMENT_3D('',#173825,#88760,#88761);
#80593=AXIS2_PLACEMENT_3D('',#173826,#88762,#88763);
#80594=AXIS2_PLACEMENT_3D('',#173879,#88764,#88765);
#80595=AXIS2_PLACEMENT_3D('',#173949,#88767,#88768);
#80596=AXIS2_PLACEMENT_3D('',#173950,#88769,#88770);
#80597=AXIS2_PLACEMENT_3D('',#174019,#88771,#88772);
#80598=AXIS2_PLACEMENT_3D('',#174616,#88773,#88774);
#80599=AXIS2_PLACEMENT_3D('',#174622,#88778,#88779);
#80600=AXIS2_PLACEMENT_3D('',#174628,#88783,#88784);
#80601=AXIS2_PLACEMENT_3D('',#174634,#88788,#88789);
#80602=AXIS2_PLACEMENT_3D('',#174636,#88790,#88791);
#80603=AXIS2_PLACEMENT_3D('',#174639,#88793,#88794);
#80604=AXIS2_PLACEMENT_3D('',#174640,#88795,#88796);
#80605=AXIS2_PLACEMENT_3D('',#174646,#88800,#88801);
#80606=AXIS2_PLACEMENT_3D('',#174652,#88805,#88806);
#80607=AXIS2_PLACEMENT_3D('',#174655,#88809,#88810);
#80608=AXIS2_PLACEMENT_3D('',#174656,#88811,#88812);
#80609=AXIS2_PLACEMENT_3D('',#174657,#88813,#88814);
#80610=AXIS2_PLACEMENT_3D('',#174670,#88821,#88822);
#80611=AXIS2_PLACEMENT_3D('',#174673,#88825,#88826);
#80612=AXIS2_PLACEMENT_3D('',#174675,#88828,#88829);
#80613=AXIS2_PLACEMENT_3D('',#174677,#88831,#88832);
#80614=AXIS2_PLACEMENT_3D('',#174679,#88834,#88835);
#80615=AXIS2_PLACEMENT_3D('',#174681,#88837,#88838);
#80616=AXIS2_PLACEMENT_3D('',#174682,#88839,#88840);
#80617=AXIS2_PLACEMENT_3D('',#174683,#88841,#88842);
#80618=AXIS2_PLACEMENT_3D('',#174684,#88843,#88844);
#80619=AXIS2_PLACEMENT_3D('',#174685,#88845,#88846);
#88584=DIRECTION('axis',(0.,0.,1.));
#88585=DIRECTION('refdir',(1.,0.,0.));
#88586=DIRECTION('center_axis',(0.173648177666903,0.,0.984807753012213));
#88587=DIRECTION('ref_axis',(0.984807753012213,0.,-0.173648177666903));
#88588=DIRECTION('',(-0.173648177666903,0.,-0.984807753012213));
#88589=DIRECTION('center_axis',(-0.173648177666903,0.,-0.984807753012213));
#88590=DIRECTION('ref_axis',(0.984807753012213,0.,-0.173648177666903));
#88591=DIRECTION('center_axis',(0.173648177666903,0.,0.984807753012213));
#88592=DIRECTION('ref_axis',(0.984807753012213,0.,-0.173648177666903));
#88593=DIRECTION('',(-0.173648177666903,0.,-0.984807753012213));
#88594=DIRECTION('center_axis',(0.173648177666903,0.,0.984807753012213));
#88595=DIRECTION('ref_axis',(0.984807753012213,0.,-0.173648177666903));
#88596=DIRECTION('',(-0.173648177666903,0.,-0.984807753012213));
#88597=DIRECTION('center_axis',(0.173648177666903,0.,0.984807753012213));
#88598=DIRECTION('ref_axis',(0.984807753012213,0.,-0.173648177666903));
#88599=DIRECTION('',(-0.173648177666903,0.,-0.984807753012213));
#88600=DIRECTION('center_axis',(0.173648177666903,0.,0.984807753012213));
#88601=DIRECTION('ref_axis',(0.984807753012213,0.,-0.173648177666903));
#88602=DIRECTION('',(-0.173648177666903,0.,-0.984807753012213));
#88603=DIRECTION('center_axis',(0.173648177666903,0.,0.984807753012213));
#88604=DIRECTION('ref_axis',(0.984807753012213,0.,-0.173648177666903));
#88605=DIRECTION('',(-0.173648177666903,0.,-0.984807753012213));
#88606=DIRECTION('center_axis',(0.173648177666903,0.,0.984807753012213));
#88607=DIRECTION('ref_axis',(0.984807753012213,0.,-0.173648177666903));
#88608=DIRECTION('',(-0.173648177666903,0.,-0.984807753012213));
#88609=DIRECTION('center_axis',(0.173648177666903,0.,0.984807753012213));
#88610=DIRECTION('ref_axis',(-0.984807753012213,0.,0.173648177666903));
#88611=DIRECTION('center_axis',(-0.173648177666902,0.,-0.984807753012213));
#88612=DIRECTION('ref_axis',(-0.984807753012213,0.,0.173648177666902));
#88613=DIRECTION('',(0.173648177666902,0.,0.984807753012213));
#88614=DIRECTION('center_axis',(0.173648177666902,0.,0.984807753012213));
#88615=DIRECTION('ref_axis',(0.984807753012213,0.,-0.173648177666902));
#88616=DIRECTION('center_axis',(-0.173648177666902,0.,-0.984807753012213));
#88617=DIRECTION('ref_axis',(-0.984807753012213,0.,0.173648177666902));
#88618=DIRECTION('',(0.173648177666902,0.,0.984807753012213));
#88619=DIRECTION('center_axis',(-0.173648177666902,0.,-0.984807753012213));
#88620=DIRECTION('ref_axis',(-0.984807753012213,0.,0.173648177666902));
#88621=DIRECTION('',(0.173648177666902,0.,0.984807753012213));
#88622=DIRECTION('center_axis',(-0.173648177666902,0.,-0.984807753012213));
#88623=DIRECTION('ref_axis',(-0.984807753012213,0.,0.173648177666902));
#88624=DIRECTION('',(0.173648177666902,0.,0.984807753012213));
#88625=DIRECTION('center_axis',(-0.173648177666902,0.,-0.984807753012213));
#88626=DIRECTION('ref_axis',(-0.984807753012213,0.,0.173648177666902));
#88627=DIRECTION('',(0.173648177666902,0.,0.984807753012213));
#88628=DIRECTION('center_axis',(-0.173648177666902,0.,-0.984807753012213));
#88629=DIRECTION('ref_axis',(-0.984807753012213,0.,0.173648177666902));
#88630=DIRECTION('',(0.173648177666902,0.,0.984807753012213));
#88631=DIRECTION('center_axis',(-0.173648177666902,0.,-0.984807753012213));
#88632=DIRECTION('ref_axis',(-0.984807753012213,0.,0.173648177666902));
#88633=DIRECTION('',(0.173648177666902,0.,0.984807753012213));
#88634=DIRECTION('center_axis',(-0.173648177666902,0.,-0.984807753012213));
#88635=DIRECTION('ref_axis',(-0.984807753012213,0.,0.173648177666902));
#88636=DIRECTION('',(-0.573576435615923,8.65956055458343E-17,0.81915204480373));
#88637=DIRECTION('center_axis',(0.173648177666902,0.,0.984807753012213));
#88638=DIRECTION('ref_axis',(0.984807753012213,0.,-0.173648177666902));
#88639=DIRECTION('center_axis',(0.173648177666903,0.,0.984807753012213));
#88640=DIRECTION('ref_axis',(0.984807753012213,0.,-0.173648177666903));
#88641=DIRECTION('',(-0.173648177666903,0.,-0.984807753012213));
#88642=DIRECTION('center_axis',(0.173648177666903,0.,0.984807753012213));
#88643=DIRECTION('ref_axis',(-0.984807753012213,0.,0.173648177666903));
#88644=DIRECTION('center_axis',(0.173648177666903,0.,0.984807753012213));
#88645=DIRECTION('ref_axis',(0.984807753012213,0.,-0.173648177666903));
#88646=DIRECTION('',(-0.173648177666903,0.,-0.984807753012213));
#88647=DIRECTION('center_axis',(0.173648177666903,0.,0.984807753012213));
#88648=DIRECTION('ref_axis',(0.984807753012213,0.,-0.173648177666903));
#88649=DIRECTION('',(-0.173648177666903,0.,-0.984807753012213));
#88650=DIRECTION('center_axis',(0.173648177666903,0.,0.984807753012213));
#88651=DIRECTION('ref_axis',(0.984807753012213,0.,-0.173648177666903));
#88652=DIRECTION('',(-0.173648177666903,0.,-0.984807753012213));
#88653=DIRECTION('center_axis',(0.173648177666903,0.,0.984807753012213));
#88654=DIRECTION('ref_axis',(0.984807753012213,0.,-0.173648177666903));
#88655=DIRECTION('',(-0.173648177666903,0.,-0.984807753012213));
#88656=DIRECTION('center_axis',(0.173648177666902,0.,0.984807753012213));
#88657=DIRECTION('ref_axis',(0.984807753012213,0.,-0.173648177666902));
#88658=DIRECTION('',(-0.173648177666902,0.,-0.984807753012213));
#88659=DIRECTION('center_axis',(0.173648177666902,0.,0.984807753012213));
#88660=DIRECTION('ref_axis',(-0.984807753012213,0.,0.173648177666902));
#88661=DIRECTION('center_axis',(0.173648177666902,0.,0.984807753012213));
#88662=DIRECTION('ref_axis',(0.984807753012213,0.,-0.173648177666902));
#88663=DIRECTION('',(-0.173648177666902,0.,-0.984807753012213));
#88664=DIRECTION('center_axis',(0.173648177666902,0.,0.984807753012213));
#88665=DIRECTION('ref_axis',(0.984807753012213,0.,-0.173648177666902));
#88666=DIRECTION('',(-0.173648177666902,0.,-0.984807753012213));
#88667=DIRECTION('center_axis',(0.173648177666902,0.,0.984807753012213));
#88668=DIRECTION('ref_axis',(0.984807753012213,0.,-0.173648177666902));
#88669=DIRECTION('',(-0.173648177666902,0.,-0.984807753012213));
#88670=DIRECTION('center_axis',(0.173648177666902,0.,0.984807753012213));
#88671=DIRECTION('ref_axis',(0.984807753012213,0.,-0.173648177666902));
#88672=DIRECTION('',(-0.173648177666902,0.,-0.984807753012213));
#88673=DIRECTION('center_axis',(0.173648177666902,0.,0.984807753012213));
#88674=DIRECTION('ref_axis',(0.984807753012213,0.,-0.173648177666902));
#88675=DIRECTION('',(-0.173648177666902,0.,-0.984807753012213));
#88676=DIRECTION('center_axis',(-0.173648177666902,0.,-0.984807753012213));
#88677=DIRECTION('ref_axis',(-0.984807753012213,0.,0.173648177666902));
#88678=DIRECTION('',(0.766044442349839,-1.0605752379922E-16,-0.642787610603163));
#88679=DIRECTION('center_axis',(0.173648177666903,0.,0.984807753012213));
#88680=DIRECTION('ref_axis',(-0.984807753012213,0.,0.173648177666903));
#88681=DIRECTION('center_axis',(0.173648177666902,0.,0.984807753012213));
#88682=DIRECTION('ref_axis',(0.984807753012213,0.,-0.173648177666902));
#88683=DIRECTION('center_axis',(-0.173648177666902,0.,-0.984807753012213));
#88684=DIRECTION('ref_axis',(0.984807753012213,0.,-0.173648177666902));
#88685=DIRECTION('center_axis',(0.173648177666902,0.,0.984807753012213));
#88686=DIRECTION('ref_axis',(0.984807753012213,0.,-0.173648177666902));
#88687=DIRECTION('center_axis',(0.173648177666902,0.,0.984807753012213));
#88688=DIRECTION('ref_axis',(0.984807753012213,0.,-0.173648177666902));
#88689=DIRECTION('',(-0.173648177666902,0.,-0.984807753012213));
#88690=DIRECTION('center_axis',(0.173648177666902,0.,0.984807753012213));
#88691=DIRECTION('ref_axis',(0.984807753012213,0.,-0.173648177666902));
#88692=DIRECTION('center_axis',(0.173648177666902,0.,0.984807753012213));
#88693=DIRECTION('ref_axis',(0.984807753012213,0.,-0.173648177666902));
#88694=DIRECTION('center_axis',(0.173648177666902,0.,0.984807753012213));
#88695=DIRECTION('ref_axis',(0.984807753012213,0.,-0.173648177666902));
#88696=DIRECTION('center_axis',(0.173648177666902,0.,0.984807753012213));
#88697=DIRECTION('ref_axis',(0.984807753012213,0.,-0.173648177666902));
#88698=DIRECTION('',(-0.173648177666902,0.,-0.984807753012213));
#88699=DIRECTION('center_axis',(0.173648177666902,0.,0.984807753012213));
#88700=DIRECTION('ref_axis',(0.984807753012213,0.,-0.173648177666902));
#88701=DIRECTION('center_axis',(0.173648177666903,0.,0.984807753012213));
#88702=DIRECTION('ref_axis',(0.984807753012213,0.,-0.173648177666903));
#88703=DIRECTION('center_axis',(0.173648177666903,0.,0.984807753012213));
#88704=DIRECTION('ref_axis',(0.984807753012213,0.,-0.173648177666903));
#88705=DIRECTION('',(-0.173648177666903,0.,-0.984807753012213));
#88706=DIRECTION('center_axis',(0.173648177666903,0.,0.984807753012213));
#88707=DIRECTION('ref_axis',(0.984807753012213,0.,-0.173648177666903));
#88708=DIRECTION('center_axis',(0.173648177666903,0.,0.984807753012213));
#88709=DIRECTION('ref_axis',(0.984807753012213,0.,-0.173648177666903));
#88710=DIRECTION('center_axis',(-0.173648177666903,0.,-0.984807753012213));
#88711=DIRECTION('ref_axis',(0.984807753012213,0.,-0.173648177666903));
#88712=DIRECTION('center_axis',(-0.173648177666902,0.,-0.984807753012213));
#88713=DIRECTION('ref_axis',(-0.984807753012213,0.,0.173648177666902));
#88714=DIRECTION('center_axis',(0.173648177666903,0.,0.984807753012213));
#88715=DIRECTION('ref_axis',(-0.984807753012213,0.,0.173648177666903));
#88716=DIRECTION('',(-0.766044442349838,1.0605752379922E-16,0.642787610603164));
#88717=DIRECTION('center_axis',(0.173648177666902,0.,0.984807753012213));
#88718=DIRECTION('ref_axis',(0.984807753012213,0.,-0.173648177666902));
#88719=DIRECTION('center_axis',(-0.173648177666902,0.,-0.984807753012213));
#88720=DIRECTION('ref_axis',(0.984807753012213,0.,-0.173648177666902));
#88721=DIRECTION('center_axis',(-0.119891710860469,0.417487739272624,0.900738566524152));
#88722=DIRECTION('ref_axis',(0.837183562575301,0.530176150202612,-0.1343016467139));
#88723=DIRECTION('',(0.766044442349838,1.0605752379922E-16,-0.642787610603164));
#88724=DIRECTION('center_axis',(-0.173648177666902,0.,-0.984807753012213));
#88725=DIRECTION('ref_axis',(-0.984807753012213,0.,0.173648177666902));
#88726=DIRECTION('center_axis',(0.173648177666902,0.,0.984807753012213));
#88727=DIRECTION('ref_axis',(0.984807753012213,0.,-0.173648177666902));
#88728=DIRECTION('',(-0.173648177666902,0.,-0.984807753012213));
#88729=DIRECTION('center_axis',(-0.173648177666902,0.,-0.984807753012213));
#88730=DIRECTION('ref_axis',(-0.984807753012213,0.,0.173648177666902));
#88731=DIRECTION('center_axis',(0.173648177666902,0.,0.984807753012213));
#88732=DIRECTION('ref_axis',(0.984807753012213,0.,-0.173648177666902));
#88733=DIRECTION('center_axis',(-0.173648177666902,0.,-0.984807753012213));
#88734=DIRECTION('ref_axis',(-0.984807753012213,0.,0.173648177666902));
#88735=DIRECTION('center_axis',(0.173648177666902,0.,0.984807753012213));
#88736=DIRECTION('ref_axis',(-0.984807753012213,0.,0.173648177666902));
#88737=DIRECTION('',(-0.173648177666902,0.,-0.984807753012213));
#88738=DIRECTION('center_axis',(-0.173648177666902,0.,-0.984807753012213));
#88739=DIRECTION('ref_axis',(-0.984807753012213,0.,0.173648177666902));
#88740=DIRECTION('center_axis',(-0.173648177666902,0.,-0.984807753012213));
#88741=DIRECTION('ref_axis',(-0.984807753012213,0.,0.173648177666902));
#88742=DIRECTION('center_axis',(-0.173648177666902,0.,-0.984807753012213));
#88743=DIRECTION('ref_axis',(-0.984807753012213,0.,0.173648177666902));
#88744=DIRECTION('center_axis',(-1.2060416625019E-16,-1.,2.12657684957543E-17));
#88745=DIRECTION('ref_axis',(0.984807753012213,-1.22464679914735E-16,-0.173648177666903));
#88746=DIRECTION('center_axis',(0.173648177666903,0.,0.984807753012213));
#88747=DIRECTION('ref_axis',(0.984807753012213,0.,-0.173648177666903));
#88748=DIRECTION('center_axis',(1.2060416625019E-16,-1.,-2.12657684957544E-17));
#88749=DIRECTION('ref_axis',(-0.984807753012213,-1.22464679914735E-16,0.173648177666903));
#88750=DIRECTION('center_axis',(-0.173648177666902,0.,-0.984807753012213));
#88751=DIRECTION('ref_axis',(0.984807753012213,0.,-0.173648177666902));
#88752=DIRECTION('center_axis',(-0.173648177666904,0.,-0.984807753012213));
#88753=DIRECTION('ref_axis',(-0.984807753012213,0.,0.173648177666904));
#88754=DIRECTION('center_axis',(-0.173648177666902,0.,-0.984807753012213));
#88755=DIRECTION('ref_axis',(-0.984807753012213,0.,0.173648177666902));
#88756=DIRECTION('',(-0.173648177666902,0.,-0.984807753012213));
#88757=DIRECTION('center_axis',(0.173648177666902,0.,0.984807753012213));
#88758=DIRECTION('ref_axis',(0.984807753012213,0.,-0.173648177666902));
#88759=DIRECTION('',(-0.173648177666902,0.,-0.984807753012213));
#88760=DIRECTION('center_axis',(-0.173648177666902,0.,-0.984807753012213));
#88761=DIRECTION('ref_axis',(-0.984807753012213,0.,0.173648177666902));
#88762=DIRECTION('center_axis',(0.173648177666902,0.,0.984807753012213));
#88763=DIRECTION('ref_axis',(0.984807753012213,0.,-0.173648177666902));
#88764=DIRECTION('center_axis',(0.173648177666902,0.,0.984807753012213));
#88765=DIRECTION('ref_axis',(0.984807753012213,0.,-0.173648177666902));
#88766=DIRECTION('',(0.573576435615923,8.65956055458343E-17,-0.81915204480373));
#88767=DIRECTION('center_axis',(-0.173648177666902,0.,-0.984807753012213));
#88768=DIRECTION('ref_axis',(-0.984807753012213,0.,0.173648177666902));
#88769=DIRECTION('center_axis',(-0.173648177666902,0.,-0.984807753012213));
#88770=DIRECTION('ref_axis',(-0.984807753012213,0.,0.173648177666902));
#88771=DIRECTION('center_axis',(0.173648177666903,0.,0.984807753012213));
#88772=DIRECTION('ref_axis',(0.984807753012213,0.,-0.173648177666903));
#88773=DIRECTION('center_axis',(-0.984807753012213,-1.65054501924843E-16,
0.173648177666902));
#88774=DIRECTION('ref_axis',(-1.67600733666031E-16,1.,-4.61841862597087E-33));
#88775=DIRECTION('',(-1.62546953165154E-16,1.,2.86614134749672E-17));
#88776=DIRECTION('',(-0.173648177666902,0.,-0.984807753012213));
#88777=DIRECTION('',(1.62546953165154E-16,-1.,-2.86614134749672E-17));
#88778=DIRECTION('center_axis',(3.41673825694851E-16,-1.,-6.02463140718734E-17));
#88779=DIRECTION('ref_axis',(-1.26946471329372E-48,6.02463140718734E-17,
-1.));
#88780=DIRECTION('',(-0.984807753012213,-3.46944695195361E-16,0.173648177666902));
#88781=DIRECTION('',(-0.173648177666902,0.,-0.984807753012213));
#88782=DIRECTION('',(0.984807753012213,3.46944695195361E-16,-0.173648177666902));
#88783=DIRECTION('center_axis',(0.984807753012213,4.95163505774528E-16,
-0.173648177666902));
#88784=DIRECTION('ref_axis',(2.57199264728249E-34,-1.,-2.85153298138474E-15));
#88785=DIRECTION('',(4.87640859495463E-16,-1.,-8.59842404249014E-17));
#88786=DIRECTION('',(-0.173648177666902,0.,-0.984807753012213));
#88787=DIRECTION('',(-4.87640859495463E-16,1.,8.59842404249014E-17));
#88788=DIRECTION('center_axis',(-0.173648177666904,0.,-0.984807753012213));
#88789=DIRECTION('ref_axis',(0.984807753012213,-1.22464679914735E-16,-0.173648177666904));
#88790=DIRECTION('center_axis',(-0.173648177666902,0.,-0.984807753012213));
#88791=DIRECTION('ref_axis',(-0.984807753012213,0.,0.173648177666902));
#88792=DIRECTION('',(-0.173648177666902,0.,-0.984807753012213));
#88793=DIRECTION('center_axis',(0.173648177666902,0.,0.984807753012213));
#88794=DIRECTION('ref_axis',(0.984807753012213,0.,-0.173648177666902));
#88795=DIRECTION('center_axis',(0.984807753012213,4.95163505774529E-16,
-0.173648177666902));
#88796=DIRECTION('ref_axis',(-2.6719634195278E-33,-1.,-2.85153298138475E-15));
#88797=DIRECTION('',(4.87640859495464E-16,-1.,-8.59842404249016E-17));
#88798=DIRECTION('',(-0.173648177666902,0.,-0.984807753012213));
#88799=DIRECTION('',(-4.87640859495464E-16,1.,8.59842404249016E-17));
#88800=DIRECTION('center_axis',(0.,1.,0.));
#88801=DIRECTION('ref_axis',(1.,0.,0.));
#88802=DIRECTION('',(0.984807753012213,0.,-0.173648177666902));
#88803=DIRECTION('',(-0.173648177666902,0.,-0.984807753012213));
#88804=DIRECTION('',(-0.984807753012213,0.,0.173648177666902));
#88805=DIRECTION('center_axis',(-0.984807753012213,-1.65054501924843E-16,
0.173648177666902));
#88806=DIRECTION('ref_axis',(-1.67600733666031E-16,1.,-4.61841862597087E-33));
#88807=DIRECTION('',(-1.62546953165154E-16,1.,2.86614134749672E-17));
#88808=DIRECTION('',(1.62546953165154E-16,-1.,-2.86614134749672E-17));
#88809=DIRECTION('center_axis',(-0.173648177666902,0.,-0.984807753012213));
#88810=DIRECTION('ref_axis',(-0.984807753012213,0.,0.173648177666902));
#88811=DIRECTION('center_axis',(-0.173648177666902,0.,-0.984807753012213));
#88812=DIRECTION('ref_axis',(-0.984807753012213,0.,0.173648177666902));
#88813=DIRECTION('center_axis',(0.173648177666902,0.,0.984807753012213));
#88814=DIRECTION('ref_axis',(0.,-1.,0.));
#88815=DIRECTION('',(-0.492403876506108,-0.866025403784438,0.0868240888334514));
#88816=DIRECTION('',(-0.984807753012213,1.12673594905287E-15,0.173648177666902));
#88817=DIRECTION('',(-0.492403876506106,0.866025403784439,0.0868240888334511));
#88818=DIRECTION('',(0.492403876506108,0.866025403784438,-0.0868240888334516));
#88819=DIRECTION('',(0.984807753012213,-3.63059361361481E-15,-0.173648177666902));
#88820=DIRECTION('',(0.492403876506104,-0.86602540378444,-0.0868240888334507));
#88821=DIRECTION('center_axis',(-0.852868531952447,0.5,0.150383733180411));
#88822=DIRECTION('ref_axis',(0.173648177666903,1.44229019851021E-17,0.984807753012213));
#88823=DIRECTION('',(-0.173648177666902,0.,-0.984807753012213));
#88824=DIRECTION('',(-0.173648177666902,0.,-0.984807753012213));
#88825=DIRECTION('center_axis',(3.57543673872449E-15,1.,-6.30445964853305E-16));
#88826=DIRECTION('ref_axis',(1.,-3.57543673872449E-15,0.));
#88827=DIRECTION('',(-0.173648177666902,0.,-0.984807753012213));
#88828=DIRECTION('center_axis',(0.852868531952448,0.499999999999999,-0.150383733180411));
#88829=DIRECTION('ref_axis',(-2.28442492313379E-17,-0.288022074947211,-0.957623769725409));
#88830=DIRECTION('',(-0.173648177666902,0.,-0.984807753012213));
#88831=DIRECTION('center_axis',(0.852868531952447,-0.5,-0.150383733180411));
#88832=DIRECTION('ref_axis',(3.00594623393023E-17,0.28802207494721,-0.95762376972541));
#88833=DIRECTION('',(-0.173648177666902,0.,-0.984807753012213));
#88834=DIRECTION('center_axis',(-1.10961829822484E-15,-1.,1.95655644264819E-16));
#88835=DIRECTION('ref_axis',(-1.,1.10961829822484E-15,0.));
#88836=DIRECTION('',(-0.173648177666902,0.,-0.984807753012213));
#88837=DIRECTION('center_axis',(-0.852868531952448,-0.5,0.150383733180411));
#88838=DIRECTION('ref_axis',(-0.505751557519974,0.862679176789449,-2.10183654596508E-18));
#88839=DIRECTION('center_axis',(0.173648177666902,0.,0.984807753012213));
#88840=DIRECTION('ref_axis',(0.,-1.,0.));
#88841=DIRECTION('center_axis',(-0.173648177666902,0.,-0.984807753012213));
#88842=DIRECTION('ref_axis',(-0.984807753012213,0.,0.173648177666902));
#88843=DIRECTION('center_axis',(0.173648177666902,0.,0.984807753012213));
#88844=DIRECTION('ref_axis',(0.,-1.,0.));
#88845=DIRECTION('center_axis',(-0.173648177666902,0.,-0.984807753012213));
#88846=DIRECTION('ref_axis',(-0.984807753012213,0.,0.173648177666902));
#161937=CARTESIAN_POINT('',(0.,0.,0.));
#161938=CARTESIAN_POINT('Origin',(69.6316151486327,0.,39.48523201752));
#161939=CARTESIAN_POINT('',(60.7509621221957,-3.44669050145648E-10,42.9650499797481));
#161940=CARTESIAN_POINT('',(60.7214966333422,3.40933537909693E-10,42.7979428885072));
#161941=CARTESIAN_POINT('',(60.4236626579685,-1.14504475720278E-15,41.1088424787055));
#161942=CARTESIAN_POINT('',(60.5714935155857,-0.705868838664094,41.7935745386541));
#161943=CARTESIAN_POINT('Ctrl Pts',(60.7509621221957,-6.89336955246539E-10,
42.9650499797481));
#161944=CARTESIAN_POINT('Ctrl Pts',(60.7509192031534,0.0120680173491838,
42.9648065737692));
#161945=CARTESIAN_POINT('Ctrl Pts',(60.7508994186887,0.0241361063428439,
42.96455982129));
#161946=CARTESIAN_POINT('Ctrl Pts',(60.7509193101621,0.0958428707922907,
42.9630736605288));
#161947=CARTESIAN_POINT('Ctrl Pts',(60.7515007820804,0.155478294986578,
42.9617554993892));
#161948=CARTESIAN_POINT('Ctrl Pts',(60.754942510561,0.334556620519833,42.9575432330028));
#161949=CARTESIAN_POINT('Ctrl Pts',(60.7595036052643,0.453948384734824,
42.9543953553669));
#161950=CARTESIAN_POINT('Ctrl Pts',(60.7761155798191,0.744414997430842,
42.9458647746078));
#161951=CARTESIAN_POINT('Ctrl Pts',(60.7905600076925,0.915297994496103,
42.9401071896087));
#161952=CARTESIAN_POINT('Ctrl Pts',(60.8626996834541,1.55969457761938,42.9154058445961));
#161953=CARTESIAN_POINT('Ctrl Pts',(60.9514830621024,2.02878367975059,42.8912541139455));
#161954=CARTESIAN_POINT('Ctrl Pts',(61.140937930544,2.73404032296258,42.8441574965815));
#161955=CARTESIAN_POINT('Ctrl Pts',(61.2166183987511,2.97638533949813,42.8259430647652));
#161956=CARTESIAN_POINT('Ctrl Pts',(61.3422630634123,3.32828801944589,42.7963719282893));
#161957=CARTESIAN_POINT('Ctrl Pts',(61.3847590529975,3.44050722830918,42.7864610538548));
#161958=CARTESIAN_POINT('Ctrl Pts',(61.4650274392059,3.64085176615261,42.7678894161257));
#161959=CARTESIAN_POINT('Ctrl Pts',(61.5020312261378,3.72928033930315,42.7593781410615));
#161960=CARTESIAN_POINT('Ctrl Pts',(61.5858627862495,3.92133306634782,42.7402000390631));
#161961=CARTESIAN_POINT('Ctrl Pts',(61.633227706131,4.02469541713465,42.7294290408078));
#161962=CARTESIAN_POINT('Ctrl Pts',(61.7850227016679,4.34069982736551,42.6951025985516));
#161963=CARTESIAN_POINT('Ctrl Pts',(61.8955736633756,4.55016508923581,42.6703616834911));
#161964=CARTESIAN_POINT('Ctrl Pts',(62.2085970580832,5.09246338308113,42.6010177453807));
#161965=CARTESIAN_POINT('Ctrl Pts',(62.4239847327386,5.41698247219077,42.55397076249));
#161966=CARTESIAN_POINT('Ctrl Pts',(62.8230995667586,5.94344979920006,42.4683579672737));
#161967=CARTESIAN_POINT('Ctrl Pts',(62.9967249163264,6.15269287100585,42.4315333194129));
#161968=CARTESIAN_POINT('Ctrl Pts',(63.2337305219164,6.41395454682262,42.3820007440121));
#161969=CARTESIAN_POINT('Ctrl Pts',(63.2890445087411,6.47333535521729,42.3704888463692));
#161970=CARTESIAN_POINT('Ctrl Pts',(63.3832206556822,6.57179445517716,42.3509777556499));
#161971=CARTESIAN_POINT('Ctrl Pts',(63.4216679290422,6.61127438489082,42.3430367156097));
#161972=CARTESIAN_POINT('Ctrl Pts',(63.508142132914,6.69848978811027,42.3252314279585));
#161973=CARTESIAN_POINT('Ctrl Pts',(63.5563430576768,6.74604201438635,42.3153431000304));
#161974=CARTESIAN_POINT('Ctrl Pts',(63.717708750903,6.90175862618079,42.2823464393979));
#161975=CARTESIAN_POINT('Ctrl Pts',(63.8330769073322,7.00753318140895,42.2589265241842));
#161976=CARTESIAN_POINT('Ctrl Pts',(64.1504342055915,7.28392522625757,42.1948375781707));
#161977=CARTESIAN_POINT('Ctrl Pts',(64.3570988832823,7.44877621875393,42.1534482115999));
#161978=CARTESIAN_POINT('Ctrl Pts',(64.9248827829799,7.86287678721484,42.0401538531613));
#161979=CARTESIAN_POINT('Ctrl Pts',(65.2970184001635,8.09529916140208,41.9662963731654));
#161980=CARTESIAN_POINT('Ctrl Pts',(65.8052692357616,8.36403058803541,41.8652218846133));
#161981=CARTESIAN_POINT('Ctrl Pts',(65.9280048808312,8.42541753420482,41.8408020108882));
#161982=CARTESIAN_POINT('Ctrl Pts',(66.1394944607363,8.52528278825529,41.7986890799829));
#161983=CARTESIAN_POINT('Ctrl Pts',(66.2275835933159,8.56517237738903,41.7811384899616));
#161984=CARTESIAN_POINT('Ctrl Pts',(66.4106265233465,8.64456456372195,41.7446458447544));
#161985=CARTESIAN_POINT('Ctrl Pts',(66.5056461828842,8.68387380520613,41.7256891366925));
#161986=CARTESIAN_POINT('Ctrl Pts',(66.7617895279916,8.78477571199218,41.6745509061279));
#161987=CARTESIAN_POINT('Ctrl Pts',(66.9239946192751,8.84338317505211,41.642128104044));
#161988=CARTESIAN_POINT('Ctrl Pts',(67.2980024243152,8.96656188810169,41.5672892164927));
#161989=CARTESIAN_POINT('Ctrl Pts',(67.5106660255118,9.0280470415826,41.5246776526347));
#161990=CARTESIAN_POINT('Ctrl Pts',(67.9981555852028,9.14977251804245,41.4269437337242));
#161991=CARTESIAN_POINT('Ctrl Pts',(68.2739360465121,9.20508480570872,41.3716133115562));
#161992=CARTESIAN_POINT('Ctrl Pts',(68.8571890355632,9.29391505157166,41.2547772168552));
#161993=CARTESIAN_POINT('Ctrl Pts',(69.1647254071317,9.32467141193665,41.1932766810052));
#161994=CARTESIAN_POINT('Ctrl Pts',(69.5647089889984,9.3439623287347,41.1137500170015));
#161995=CARTESIAN_POINT('Ctrl Pts',(69.6562243240114,9.34697706212247,41.0955861650997));
#161996=CARTESIAN_POINT('Ctrl Pts',(69.8013386906838,9.34954143049101,41.0668464675245));
#161997=CARTESIAN_POINT('Ctrl Pts',(69.8549111944427,9.3500097683724,41.0562499923985));
#161998=CARTESIAN_POINT('Ctrl Pts',(69.9624342094911,9.34998985422666,41.0350125729487));
#161999=CARTESIAN_POINT('Ctrl Pts',(70.0163826392544,9.34949496796775,41.0243722134257));
#162000=CARTESIAN_POINT('Ctrl Pts',(70.1637306170531,9.34681879104554,40.9953469065423));
#162001=CARTESIAN_POINT('Ctrl Pts',(70.2571117094745,9.34366884165001,40.9769922278763));
#162002=CARTESIAN_POINT('Ctrl Pts',(70.6773069937479,9.3229461074411,40.8945362718053));
#162003=CARTESIAN_POINT('Ctrl Pts',(71.0031659378946,9.28902180796155,40.8309570144352));
#162004=CARTESIAN_POINT('Ctrl Pts',(71.8674102576155,9.15116326016299,40.662325578389));
#162005=CARTESIAN_POINT('Ctrl Pts',(72.3995994001381,9.01576763460601,40.5584222401047));
#162006=CARTESIAN_POINT('Ctrl Pts',(73.0476815844185,8.78648593714721,40.4304890949787));
#162007=CARTESIAN_POINT('Ctrl Pts',(73.1777328614347,8.73707433129832,40.4047472757752));
#162008=CARTESIAN_POINT('Ctrl Pts',(73.3956105142267,8.64849654971577,40.3614910708849));
#162009=CARTESIAN_POINT('Ctrl Pts',(73.484032373736,8.61089910502389,40.343899276431));
#162010=CARTESIAN_POINT('Ctrl Pts',(73.6649595495966,8.53054732173658,40.3078240856901));
#162011=CARTESIAN_POINT('Ctrl Pts',(73.7573777406432,8.4876244032667,40.2893532515719));
#162012=CARTESIAN_POINT('Ctrl Pts',(74.0004265282063,8.36972470535843,40.2406604292785));
#162013=CARTESIAN_POINT('Ctrl Pts',(74.1497584237987,8.29208704341949,40.2106215816142));
#162014=CARTESIAN_POINT('Ctrl Pts',(74.3981966281126,8.15402855962329,40.1604500397329));
#162015=CARTESIAN_POINT('Ctrl Pts',(74.4984336502322,8.0957921161285,40.1401514742407));
#162016=CARTESIAN_POINT('Ctrl Pts',(74.9481911429238,7.82287096350835,40.0488374021029));
#162017=CARTESIAN_POINT('Ctrl Pts',(75.2843906030439,7.58645787724419,39.9798997485762));
#162018=CARTESIAN_POINT('Ctrl Pts',(75.7911853466634,7.17657396715865,39.8754833888091));
#162019=CARTESIAN_POINT('Ctrl Pts',(75.9725038848175,7.01774795338829,39.8380182132098));
#162020=CARTESIAN_POINT('Ctrl Pts',(76.2051496289845,6.79727004618545,39.7899602723674));
#162021=CARTESIAN_POINT('Ctrl Pts',(76.2620722196148,6.74191519448013,39.7782029879682));
#162022=CARTESIAN_POINT('Ctrl Pts',(76.3571718770091,6.64702290325669,39.7585707422223));
#162023=CARTESIAN_POINT('Ctrl Pts',(76.3957140468795,6.60787434334059,39.7506174578851));
#162024=CARTESIAN_POINT('Ctrl Pts',(76.4817438056552,6.5189226116427,39.7328737856309));
#162025=CARTESIAN_POINT('Ctrl Pts',(76.5290332059677,6.46892525082887,39.7231256672476));
#162026=CARTESIAN_POINT('Ctrl Pts',(76.6874077606057,6.29770311810571,39.690484170149));
#162027=CARTESIAN_POINT('Ctrl Pts',(76.795877004395,6.17399840367566,39.668137262632));
#162028=CARTESIAN_POINT('Ctrl Pts',(77.0857415310214,5.82513715987257,39.6083099896063));
#162029=CARTESIAN_POINT('Ctrl Pts',(77.2601226654631,5.59416944127951,39.5721887525485));
#162030=CARTESIAN_POINT('Ctrl Pts',(77.6515396006687,5.02212018218087,39.4902450361049));
#162031=CARTESIAN_POINT('Ctrl Pts',(77.8578449431254,4.67415547923311,39.4462921317525));
#162032=CARTESIAN_POINT('Ctrl Pts',(78.1046014984847,4.18871023810343,39.3920498018891));
#162033=CARTESIAN_POINT('Ctrl Pts',(78.1652837158995,4.06238592074089,39.3785453154062));
#162034=CARTESIAN_POINT('Ctrl Pts',(78.2631915831818,3.84626793852728,39.3564489184212));
#162035=CARTESIAN_POINT('Ctrl Pts',(78.3018888151383,3.75719145402448,39.3476241340115));
#162036=CARTESIAN_POINT('Ctrl Pts',(78.3789448603873,3.57199554854562,39.3298527285725));
#162037=CARTESIAN_POINT('Ctrl Pts',(78.4171123309928,3.47580805464009,39.3209367916894));
#162038=CARTESIAN_POINT('Ctrl Pts',(78.5141091029915,3.21905713401295,39.2979627927361));
#162039=CARTESIAN_POINT('Ctrl Pts',(78.5701699844634,3.05745132674366,39.2843453283008));
#162040=CARTESIAN_POINT('Ctrl Pts',(78.7155991001841,2.59812914572263,39.2479997830359));
#162041=CARTESIAN_POINT('Ctrl Pts',(78.7947105803263,2.29727335994955,39.2269254188885));
#162042=CARTESIAN_POINT('Ctrl Pts',(78.9676427614793,1.47685659793284,39.1769607291523));
#162043=CARTESIAN_POINT('Ctrl Pts',(79.0331076349819,0.952189915331092,
39.1528860741283));
#162044=CARTESIAN_POINT('Ctrl Pts',(79.0584314102317,0.334455309251635,
39.1348128756305));
#162045=CARTESIAN_POINT('Ctrl Pts',(79.0608456650541,0.244315143102979,
39.1324313915528));
#162046=CARTESIAN_POINT('Ctrl Pts',(79.0626614058751,0.100181503155015,
39.129042836859));
#162047=CARTESIAN_POINT('Ctrl Pts',(79.06288328759,0.0462077443700452,39.1278679029619));
#162048=CARTESIAN_POINT('Ctrl Pts',(79.0624040527268,-0.0634553533171274,
39.1256746394488));
#162049=CARTESIAN_POINT('Ctrl Pts',(79.0616733962745,-0.119142365220631,
39.12466236035));
#162050=CARTESIAN_POINT('Ctrl Pts',(79.0582951870379,-0.27354429590103,
39.1221316435911));
#162051=CARTESIAN_POINT('Ctrl Pts',(79.0546026174417,-0.372232464434601,
39.1208270165568));
#162052=CARTESIAN_POINT('Ctrl Pts',(79.0424605751304,-0.601370998227225,
39.1185009079195));
#162053=CARTESIAN_POINT('Ctrl Pts',(79.0328599279125,-0.731741890152604,
39.1177077803513));
#162054=CARTESIAN_POINT('Ctrl Pts',(78.986046386072,-1.22772338659078,39.1166269345832));
#162055=CARTESIAN_POINT('Ctrl Pts',(78.9303567892656,-1.59125959251295,
39.1198472086018));
#162056=CARTESIAN_POINT('Ctrl Pts',(78.7686414432441,-2.34953855474448,
39.1342001747182));
#162057=CARTESIAN_POINT('Ctrl Pts',(78.657917495894,-2.74248264257331,39.1461433744119));
#162058=CARTESIAN_POINT('Ctrl Pts',(78.4781970545509,-3.25155709505892,
39.1672246498674));
#162059=CARTESIAN_POINT('Ctrl Pts',(78.4315853149677,-3.375252006404,39.1728042309735));
#162060=CARTESIAN_POINT('Ctrl Pts',(78.3462069440908,-3.58815734979082,
39.1831984435764));
#162061=CARTESIAN_POINT('Ctrl Pts',(78.3086271336934,-3.67783015233958,
39.1878250506795));
#162062=CARTESIAN_POINT('Ctrl Pts',(78.2268128667642,-3.86488574142884,
39.19799958543));
#162063=CARTESIAN_POINT('Ctrl Pts',(78.1822950065419,-3.96212685525035,
39.2035926000933));
#162064=CARTESIAN_POINT('Ctrl Pts',(78.0535514226896,-4.23114731727244,
39.2199194829015));
#162065=CARTESIAN_POINT('Ctrl Pts',(77.9657471341904,-4.40112023962495,
39.2312221766895));
#162066=CARTESIAN_POINT('Ctrl Pts',(77.7444449990251,-4.79927820762073,
39.2601108414533));
#162067=CARTESIAN_POINT('Ctrl Pts',(77.6064098334748,-5.02469947435709,
39.2784322307871));
#162068=CARTESIAN_POINT('Ctrl Pts',(77.19973334068,-5.63000120720818,39.3333862918379));
#162069=CARTESIAN_POINT('Ctrl Pts',(76.9122235887559,-5.99598527899814,
39.373244174817));
#162070=CARTESIAN_POINT('Ctrl Pts',(76.5419422192553,-6.40142050268571,
39.4265192775781));
#162071=CARTESIAN_POINT('Ctrl Pts',(76.4839137265088,-6.46325055282909,
39.4349196139379));
#162072=CARTESIAN_POINT('Ctrl Pts',(76.3863446747382,-6.56442284904681,
39.4491373703105));
#162073=CARTESIAN_POINT('Ctrl Pts',(76.3472706056982,-6.60422189491118,
39.4548555087303));
#162074=CARTESIAN_POINT('Ctrl Pts',(76.2609901857356,-6.69054611573872,
39.4675367622796));
#162075=CARTESIAN_POINT('Ctrl Pts',(76.2136431890314,-6.73692078537221,
39.4745300494353));
#162076=CARTESIAN_POINT('Ctrl Pts',(76.0608825130346,-6.88339300460807,
39.4971912394676));
#162077=CARTESIAN_POINT('Ctrl Pts',(75.9536540435158,-6.98150601388505,
39.5132440086012));
#162078=CARTESIAN_POINT('Ctrl Pts',(75.6692571413004,-7.22975679850689,
39.5561046507005));
#162079=CARTESIAN_POINT('Ctrl Pts',(75.4887461962047,-7.37579187955797,
39.5835819795774));
#162080=CARTESIAN_POINT('Ctrl Pts',(74.9035266768229,-7.81395952585248,
39.6731189579654));
#162081=CARTESIAN_POINT('Ctrl Pts',(74.4809154638828,-8.0800089184283,39.738385719014));
#162082=CARTESIAN_POINT('Ctrl Pts',(73.9196702373565,-8.37272654588218,
39.824788668525));
#162083=CARTESIAN_POINT('Ctrl Pts',(73.7988255123913,-8.43241287021897,
39.8433809212834));
#162084=CARTESIAN_POINT('Ctrl Pts',(73.5889671351575,-8.53038473369496,
39.8756351846373));
#162085=CARTESIAN_POINT('Ctrl Pts',(73.5005690548199,-8.56996321432973,
39.8892118287083));
#162086=CARTESIAN_POINT('Ctrl Pts',(73.3153955474117,-8.64937968836004,
39.9176281211049));
#162087=CARTESIAN_POINT('Ctrl Pts',(73.2185330405093,-8.68897527875358,
39.932479222441));
#162088=CARTESIAN_POINT('Ctrl Pts',(72.9532887314133,-8.79214497941568,
39.9731089000321));
#162089=CARTESIAN_POINT('Ctrl Pts',(72.7837008382284,-8.85242664272219,
39.9990444158494));
#162090=CARTESIAN_POINT('Ctrl Pts',(72.3887303907514,-8.97986140418576,
40.0593643646413));
#162091=CARTESIAN_POINT('Ctrl Pts',(72.1623350021658,-9.04340297899018,
40.0938768823119));
#162092=CARTESIAN_POINT('Ctrl Pts',(71.617239510483,-9.17399727929768,40.1769217691508));
#162093=CARTESIAN_POINT('Ctrl Pts',(71.2969423699594,-9.23288913498765,
40.2256738259159));
#162094=CARTESIAN_POINT('Ctrl Pts',(70.7033554107673,-9.30959810348645,
40.3163214480786));
#162095=CARTESIAN_POINT('Ctrl Pts',(70.4310517712827,-9.33245101807529,
40.3580215670076));
#162096=CARTESIAN_POINT('Ctrl Pts',(70.0799811772284,-9.34612410411519,
40.4121596413414));
#162097=CARTESIAN_POINT('Ctrl Pts',(70.001735239084,-9.34816517330635,40.4242500444604));
#162098=CARTESIAN_POINT('Ctrl Pts',(69.8725958771397,-9.3498737679233,40.4442521743555));
#162099=CARTESIAN_POINT('Ctrl Pts',(69.8217112419767,-9.35012180670517,
40.4521459348212));
#162100=CARTESIAN_POINT('Ctrl Pts',(69.7125019630862,-9.34974153666798,
40.4691163164953));
#162101=CARTESIAN_POINT('Ctrl Pts',(69.6541811516513,-9.34897972012343,
40.4781960324333));
#162102=CARTESIAN_POINT('Ctrl Pts',(69.4812061468428,-9.34506246656331,
40.5051693708976));
#162103=CARTESIAN_POINT('Ctrl Pts',(69.3666051402666,-9.34030547782814,
40.5230967975248));
#162104=CARTESIAN_POINT('Ctrl Pts',(69.0899791244209,-9.32359642814478,
40.5664658603422));
#162105=CARTESIAN_POINT('Ctrl Pts',(68.9281266169439,-9.30947603019504,
40.5919200340261));
#162106=CARTESIAN_POINT('Ctrl Pts',(68.4535834696805,-9.25528136736339,
40.6666497535579));
#162107=CARTESIAN_POINT('Ctrl Pts',(68.1424690042874,-9.20332329564257,
40.7157652313149));
#162108=CARTESIAN_POINT('Ctrl Pts',(67.4541103344533,-9.05141408180703,
40.8241020605481));
#162109=CARTESIAN_POINT('Ctrl Pts',(67.079248786922,-8.94319346340559,40.88286021374));
#162110=CARTESIAN_POINT('Ctrl Pts',(66.5890744650842,-8.76715364547078,
40.9589555376969));
#162111=CARTESIAN_POINT('Ctrl Pts',(66.4669152086575,-8.72031254626882,
40.977858292704));
#162112=CARTESIAN_POINT('Ctrl Pts',(66.2565687644482,-8.63446293028694,
41.0102901458141));
#162113=CARTESIAN_POINT('Ctrl Pts',(66.1679313543636,-8.59665178470926,
41.0239198038748));
#162114=CARTESIAN_POINT('Ctrl Pts',(65.9829628097528,-8.5142907182108,41.05228233946));
#162115=CARTESIAN_POINT('Ctrl Pts',(65.8867712277192,-8.46945191562868,
41.0669856909708));
#162116=CARTESIAN_POINT('Ctrl Pts',(65.6204485629991,-8.33966229462194,
41.1075638238008));
#162117=CARTESIAN_POINT('Ctrl Pts',(65.4520932642186,-8.25107386304867,
41.133063066968));
#162118=CARTESIAN_POINT('Ctrl Pts',(65.0574591954392,-8.02758609051135,
41.1924926723887));
#162119=CARTESIAN_POINT('Ctrl Pts',(64.8339111359362,-7.88805833575394,
41.22587649101));
#162120=CARTESIAN_POINT('Ctrl Pts',(64.2352897386876,-7.47793010934565,
41.3146801886983));
#162121=CARTESIAN_POINT('Ctrl Pts',(63.8737831585359,-7.18835011748932,
41.3676081483287));
#162122=CARTESIAN_POINT('Ctrl Pts',(63.4732300941808,-6.81510724127859,
41.4262442735139));
#162123=CARTESIAN_POINT('Ctrl Pts',(63.4121166986949,-6.75658119731008,
41.4351912912859));
#162124=CARTESIAN_POINT('Ctrl Pts',(63.3120719743635,-6.65811700365124,
41.4498486271939));
#162125=CARTESIAN_POINT('Ctrl Pts',(63.2726899351033,-6.61865330596437,
41.4556214666843));
#162126=CARTESIAN_POINT('Ctrl Pts',(63.1872159229516,-6.53144649699522,
41.4681597250115));
#162127=CARTESIAN_POINT('Ctrl Pts',(63.1412742178653,-6.4835585285477,41.474904062577));
#162128=CARTESIAN_POINT('Ctrl Pts',(62.9959937969129,-6.32884420324721,
41.4962373956945));
#162129=CARTESIAN_POINT('Ctrl Pts',(62.8986331836758,-6.22015213650578,
41.5105428502645));
#162130=CARTESIAN_POINT('Ctrl Pts',(62.6520250972985,-5.93149374318229,
41.5467136236367));
#162131=CARTESIAN_POINT('Ctrl Pts',(62.5068781974154,-5.74808174746316,
41.5679366968159));
#162132=CARTESIAN_POINT('Ctrl Pts',(62.0738696639912,-5.15670710711674,
41.630652562326));
#162133=CARTESIAN_POINT('Ctrl Pts',(61.8113955772076,-4.73079800418125,
41.6677164516398));
#162134=CARTESIAN_POINT('Ctrl Pts',(61.5217418649459,-4.16471875358986,
41.7062671022462));
#162135=CARTESIAN_POINT('Ctrl Pts',(61.4624250766333,-4.04235722803926,
41.7140076263576));
#162136=CARTESIAN_POINT('Ctrl Pts',(61.3650484619538,-3.82994348226314,
41.7264252181212));
#162137=CARTESIAN_POINT('Ctrl Pts',(61.3257143237137,-3.74051480215264,
41.7313502454636));
#162138=CARTESIAN_POINT('Ctrl Pts',(61.2467825581074,-3.55325405699004,
41.7410341029529));
#162139=CARTESIAN_POINT('Ctrl Pts',(61.2074208088727,-3.45533516128047,
41.7457474788098));
#162140=CARTESIAN_POINT('Ctrl Pts',(61.1048735628266,-3.18739655600134,
41.7576970162287));
#162141=CARTESIAN_POINT('Ctrl Pts',(61.0449066804154,-3.01616693201691,
41.7643101649349));
#162142=CARTESIAN_POINT('Ctrl Pts',(60.76897626378,-2.14942954181391,41.792733402383));
#162143=CARTESIAN_POINT('Ctrl Pts',(60.6284535303241,-1.43210428208144,
41.7999744970083));
#162144=CARTESIAN_POINT('Ctrl Pts',(60.5714935164259,-0.705868838607116,
41.7935745380961));
#162145=CARTESIAN_POINT('',(64.7021225441964,-7.81768501240386,41.0652331929315));
#162146=CARTESIAN_POINT('Origin',(69.7531688729995,0.,40.1745974446286));
#162147=CARTESIAN_POINT('Ctrl Pts',(64.7021225443845,-7.81768501217606,
41.0652331931716));
#162148=CARTESIAN_POINT('Ctrl Pts',(64.9099291419011,-7.95559121670532,
41.0332711740937));
#162149=CARTESIAN_POINT('Ctrl Pts',(65.1231278425908,-8.08495767398618,
41.0004097291694));
#162150=CARTESIAN_POINT('Ctrl Pts',(65.4716214575531,-8.27753191386777,
40.9467318773754));
#162151=CARTESIAN_POINT('Ctrl Pts',(65.603709879995,-8.3463928018554,40.9263939606144));
#162152=CARTESIAN_POINT('Ctrl Pts',(65.8191483003094,-8.45213403987724,
40.8932548174706));
#162153=CARTESIAN_POINT('Ctrl Pts',(65.901493765702,-8.49104321942166,40.8805955987882));
#162154=CARTESIAN_POINT('Ctrl Pts',(66.0710906980177,-8.56811717995667,
40.8545417556752));
#162155=CARTESIAN_POINT('Ctrl Pts',(66.1583839475758,-8.60616165819395,
40.8411415749923));
#162156=CARTESIAN_POINT('Ctrl Pts',(66.3536718854519,-8.6876826377093,40.8111883826705));
#162157=CARTESIAN_POINT('Ctrl Pts',(66.4619292521254,-8.73047428214599,
40.7946006703207));
#162158=CARTESIAN_POINT('Ctrl Pts',(66.8094118826833,-8.86023810010581,
40.7414125136883));
#162159=CARTESIAN_POINT('Ctrl Pts',(67.0514066100683,-8.93930042173176,
40.7044557862505));
#162160=CARTESIAN_POINT('Ctrl Pts',(67.7571047729953,-9.13776017779192,
40.5968433952722));
#162161=CARTESIAN_POINT('Ctrl Pts',(68.2271730990255,-9.23099027745907,
40.5253868666142));
#162162=CARTESIAN_POINT('Ctrl Pts',(68.8701978555925,-9.3068500034002,40.4271135316917));
#162163=CARTESIAN_POINT('Ctrl Pts',(69.0387136091781,-9.32200436187663,
40.4013064915722));
#162164=CARTESIAN_POINT('Ctrl Pts',(69.3252255904355,-9.33977352546646,
40.3572696612854));
#162165=CARTESIAN_POINT('Ctrl Pts',(69.4430414418329,-9.34479432053206,
40.3391156491253));
#162166=CARTESIAN_POINT('Ctrl Pts',(69.6198086283044,-9.3489025349949,40.3117858493284));
#162167=CARTESIAN_POINT('Ctrl Pts',(69.6787161997998,-9.34970163172074,
40.3026628616066));
#162168=CARTESIAN_POINT('Ctrl Pts',(69.7888923395229,-9.35013034127187,
40.2855673639611));
#162169=CARTESIAN_POINT('Ctrl Pts',(69.8401580478434,-9.34989819149722,
40.2775991082422));
#162170=CARTESIAN_POINT('Ctrl Pts',(69.9688753128024,-9.34823141733855,
40.2575613890772));
#162171=CARTESIAN_POINT('Ctrl Pts',(70.0463135826783,-9.34624290081183,
40.2454783741426));
#162172=CARTESIAN_POINT('Ctrl Pts',(70.3993749270469,-9.3326790162918,40.19028576075));
#162173=CARTESIAN_POINT('Ctrl Pts',(70.6743840483041,-9.30960096897578,
40.1470112001541));
#162174=CARTESIAN_POINT('Ctrl Pts',(71.2703390126847,-9.2322717327853,40.0531019595741));
#162175=CARTESIAN_POINT('Ctrl Pts',(71.590305634569,-9.17324724574807,40.0026016387007));
#162176=CARTESIAN_POINT('Ctrl Pts',(72.1342576688283,-9.04258086023592,
39.9170961119826));
#162177=CARTESIAN_POINT('Ctrl Pts',(72.3598283403125,-8.97914977186504,
39.8817416784996));
#162178=CARTESIAN_POINT('Ctrl Pts',(72.7536004321475,-8.85194623240719,
39.8203334737841));
#162179=CARTESIAN_POINT('Ctrl Pts',(72.9227897736543,-8.79175455627838,
39.7940518883034));
#162180=CARTESIAN_POINT('Ctrl Pts',(73.187586112548,-8.68870822660458,39.7531134933955));
#162181=CARTESIAN_POINT('Ctrl Pts',(73.2843758934491,-8.64912815850986,
39.7381913937325));
#162182=CARTESIAN_POINT('Ctrl Pts',(73.4695020748567,-8.56971438833897,
39.7097354223797));
#162183=CARTESIAN_POINT('Ctrl Pts',(73.5579232081475,-8.53012038003188,
39.6961821917585));
#162184=CARTESIAN_POINT('Ctrl Pts',(73.7679775496655,-8.43205304801048,
39.6640779187476));
#162185=CARTESIAN_POINT('Ctrl Pts',(73.8889993798093,-8.37228111383074,
39.64565720777));
#162186=CARTESIAN_POINT('Ctrl Pts',(74.4485702831968,-8.08046556722084,
39.5608356485478));
#162187=CARTESIAN_POINT('Ctrl Pts',(74.8696942638692,-7.81573964254023,
39.4980731132566));
#162188=CARTESIAN_POINT('Ctrl Pts',(75.454875964055,-7.37857536573221,39.4117729182769));
#162189=CARTESIAN_POINT('Ctrl Pts',(75.6365741059568,-7.23184311479738,
39.3851123634291));
#162190=CARTESIAN_POINT('Ctrl Pts',(75.9225061442735,-6.98254187786002,
39.343228249221));
#162191=CARTESIAN_POINT('Ctrl Pts',(76.0301526622264,-6.88413152250635,
39.3274768518852));
#162192=CARTESIAN_POINT('Ctrl Pts',(76.1833606321964,-6.73729819969614,
39.305043322013));
#162193=CARTESIAN_POINT('Ctrl Pts',(76.2307711450976,-6.69087619095716,
39.298098948135));
#162194=CARTESIAN_POINT('Ctrl Pts',(76.317098467256,-6.60451828615961,39.2854448903652));
#162195=CARTESIAN_POINT('Ctrl Pts',(76.3561589204221,-6.56473437913438,
39.2797151301512));
#162196=CARTESIAN_POINT('Ctrl Pts',(76.4536035861444,-6.46368276944742,
39.2654136889022));
#162197=CARTESIAN_POINT('Ctrl Pts',(76.5115183804176,-6.40196036492774,
39.2569075548689));
#162198=CARTESIAN_POINT('Ctrl Pts',(76.8808383246451,-5.99744671559585,
39.2026671252686));
#162199=CARTESIAN_POINT('Ctrl Pts',(77.1673940716131,-5.63236890441859,
39.160622292212));
#162200=CARTESIAN_POINT('Ctrl Pts',(77.5736339895177,-5.02746590723789,
39.1025512176068));
#162201=CARTESIAN_POINT('Ctrl Pts',(77.7119571976737,-4.80142944591827,
39.0831248645218));
#162202=CARTESIAN_POINT('Ctrl Pts',(77.9336393552404,-4.4023387739747,39.0528268008962));
#162203=CARTESIAN_POINT('Ctrl Pts',(78.0215496001567,-4.23207139359831,
39.0410830962408));
#162204=CARTESIAN_POINT('Ctrl Pts',(78.1504193277892,-3.96270033470048,
39.0243574396474));
#162205=CARTESIAN_POINT('Ctrl Pts',(78.194953326286,-3.86540989880228,39.0186813393949));
#162206=CARTESIAN_POINT('Ctrl Pts',(78.2767867924039,-3.67832186678483,
39.0084620556804));
#162207=CARTESIAN_POINT('Ctrl Pts',(78.3143701387671,-3.58866678618905,
39.0038633281515));
#162208=CARTESIAN_POINT('Ctrl Pts',(78.3997376988653,-3.37590375714255,
38.993651629148));
#162209=CARTESIAN_POINT('Ctrl Pts',(78.4463465042021,-3.25233589412948,
38.9882663416327));
#162210=CARTESIAN_POINT('Ctrl Pts',(78.6212760349658,-2.75753448491971,
38.9688513028008));
#162211=CARTESIAN_POINT('Ctrl Pts',(78.7291329471674,-2.37934168111355,
38.9587759037915));
#162212=CARTESIAN_POINT('Ctrl Pts',(78.8803588050422,-1.6894245788458,38.9484853562719));
#162213=CARTESIAN_POINT('Ctrl Pts',(78.9322711270322,-1.38019536582268,
38.9466867740245));
#162214=CARTESIAN_POINT('Ctrl Pts',(78.9883945982626,-0.901753143507995,
38.9478980353824));
#162215=CARTESIAN_POINT('Ctrl Pts',(79.0035527398303,-0.734046478088404,
38.9490662801639));
#162216=CARTESIAN_POINT('Ctrl Pts',(79.021712735615,-0.448293177242299,
38.9522526504847));
#162217=CARTESIAN_POINT('Ctrl Pts',(79.0269932488723,-0.330427808422369,
38.9539114528656));
#162218=CARTESIAN_POINT('Ctrl Pts',(79.031612637129,-0.153153714515487,
38.9569014565597));
#162219=CARTESIAN_POINT('Ctrl Pts',(79.0325998969399,-0.0937954228283715,
38.9579859742503));
#162220=CARTESIAN_POINT('Ctrl Pts',(79.0333974134861,0.0169279385186524,
38.9601606884374));
#162221=CARTESIAN_POINT('Ctrl Pts',(79.0333482878283,0.0682895297017857,
38.9612299826708));
#162222=CARTESIAN_POINT('Ctrl Pts',(79.0321661367575,0.198021635936845,
38.9640866420856));
#162223=CARTESIAN_POINT('Ctrl Pts',(79.0304765796834,0.276381359886681,
38.9659559926883));
#162224=CARTESIAN_POINT('Ctrl Pts',(79.0183263209127,0.633666418580387,
38.9751601075958));
#162225=CARTESIAN_POINT('Ctrl Pts',(78.9964906347116,0.912015756738901,
38.9842273615322));
#162226=CARTESIAN_POINT('Ctrl Pts',(78.9222459742806,1.51522758868374,39.0084924607264));
#162227=CARTESIAN_POINT('Ctrl Pts',(78.8651299927986,1.83910243806911,39.0244819773412));
#162228=CARTESIAN_POINT('Ctrl Pts',(78.738228402067,2.38963678298835,39.0572660187727));
#162229=CARTESIAN_POINT('Ctrl Pts',(78.6765170601622,2.61791813564908,39.0725671268995));
#162230=CARTESIAN_POINT('Ctrl Pts',(78.5526188365452,3.01636894768214,39.10243812103));
#162231=CARTESIAN_POINT('Ctrl Pts',(78.4939490887731,3.18755085990217,39.1163342253296));
#162232=CARTESIAN_POINT('Ctrl Pts',(78.3934522651991,3.4554322822175,39.139806851963));
#162233=CARTESIAN_POINT('Ctrl Pts',(78.3548402839376,3.55334265931871,39.1487597334953));
#162234=CARTESIAN_POINT('Ctrl Pts',(78.2773489730381,3.74059758915825,39.1666103102783));
#162235=CARTESIAN_POINT('Ctrl Pts',(78.2387049339176,3.83002894642994,39.1754620993184));
#162236=CARTESIAN_POINT('Ctrl Pts',(78.1429709962522,4.04246734706523,39.1972765608363));
#162237=CARTESIAN_POINT('Ctrl Pts',(78.084606054502,4.16484966159054,39.2104865870434));
#162238=CARTESIAN_POINT('Ctrl Pts',(77.799593871057,4.73064365405723,39.274587699024));
#162239=CARTESIAN_POINT('Ctrl Pts',(77.5408584132845,5.15626362949474,39.3317025860928));
#162240=CARTESIAN_POINT('Ctrl Pts',(77.1132252810091,5.74753951385887,39.4239889135004));
#162241=CARTESIAN_POINT('Ctrl Pts',(76.9696401386509,5.93110941779543,39.4546846524212));
#162242=CARTESIAN_POINT('Ctrl Pts',(76.7255830412657,6.21997401145938,39.5062520219091));
#162243=CARTESIAN_POINT('Ctrl Pts',(76.6292193151011,6.32872124860053,39.5264731620379));
#162244=CARTESIAN_POINT('Ctrl Pts',(76.4853992540915,6.48349819894039,39.5564137181252));
#162245=CARTESIAN_POINT('Ctrl Pts',(76.4399244267392,6.53139445419446,39.5658475399373));
#162246=CARTESIAN_POINT('Ctrl Pts',(76.3553175251908,6.61860772924905,39.5833338009163));
#162247=CARTESIAN_POINT('Ctrl Pts',(76.3163360324784,6.65806970019674,39.5913649406049));
#162248=CARTESIAN_POINT('Ctrl Pts',(76.2173125465778,6.75651711073263,39.6117061275029));
#162249=CARTESIAN_POINT('Ctrl Pts',(76.1568198200928,6.81502888792346,39.6240784272744));
#162250=CARTESIAN_POINT('Ctrl Pts',(75.7603141335445,7.18815527664897,39.7048736748925));
#162251=CARTESIAN_POINT('Ctrl Pts',(75.4022350063728,7.47765755901793,39.7764953298718));
#162252=CARTESIAN_POINT('Ctrl Pts',(74.8088414438977,7.88781000732387,39.8946865986885));
#162253=CARTESIAN_POINT('Ctrl Pts',(74.5870866063093,8.0274060971477,39.9387517479531));
#162254=CARTESIAN_POINT('Ctrl Pts',(74.1955604120527,8.25098287144491,40.0165789033074));
#162255=CARTESIAN_POINT('Ctrl Pts',(74.0285217136279,8.33959720428372,40.0497895890592));
#162256=CARTESIAN_POINT('Ctrl Pts',(73.764267943593,8.46941388715207,40.1023822276028));
#162257=CARTESIAN_POINT('Ctrl Pts',(73.6688276635238,8.51425702044499,40.1213873714215));
#162258=CARTESIAN_POINT('Ctrl Pts',(73.4853018342307,8.59662186686805,40.1579580924078));
#162259=CARTESIAN_POINT('Ctrl Pts',(73.3973556988506,8.63443279574562,40.1754935984856));
#162260=CARTESIAN_POINT('Ctrl Pts',(73.1886531466785,8.72027658717094,40.2171343876706));
#162261=CARTESIAN_POINT('Ctrl Pts',(73.0674472993297,8.76711237113641,40.2413393450917));
#162262=CARTESIAN_POINT('Ctrl Pts',(72.5821328152752,8.94275033976013,40.338342781684));
#162263=CARTESIAN_POINT('Ctrl Pts',(72.2112304326012,9.05071485767094,40.4126851785677));
#162264=CARTESIAN_POINT('Ctrl Pts',(71.534686762407,9.20141362361004,40.5483505088428));
#162265=CARTESIAN_POINT('Ctrl Pts',(71.2314905750788,9.25284220495611,40.6091652611431));
#162266=CARTESIAN_POINT('Ctrl Pts',(70.7622418829434,9.30791458482255,40.7030133799736));
#162267=CARTESIAN_POINT('Ctrl Pts',(70.5976869651754,9.32264802401544,40.7358711866092));
#162268=CARTESIAN_POINT('Ctrl Pts',(70.3172886761538,9.33998747155943,40.7917033086452));
#162269=CARTESIAN_POINT('Ctrl Pts',(70.2016312674559,9.34490186286306,40.8146873293401));
#162270=CARTESIAN_POINT('Ctrl Pts',(70.0276706962275,9.34893341688283,40.8491664836239));
#162271=CARTESIAN_POINT('Ctrl Pts',(69.9694247596809,9.34971765598558,40.8606955197955));
#162272=CARTESIAN_POINT('Ctrl Pts',(69.8607763742654,9.35012579552253,40.8821685768101));
#162273=CARTESIAN_POINT('Ctrl Pts',(69.8103780187963,9.34989192368821,40.8921157716346));
#162274=CARTESIAN_POINT('Ctrl Pts',(69.6830817400965,9.34823232626495,40.9172095181326));
#162275=CARTESIAN_POINT('Ctrl Pts',(69.6061916781604,9.34624452969243,40.9323385442458));
#162276=CARTESIAN_POINT('Ctrl Pts',(69.255382636236,9.33267699110307,41.0012606129443));
#162277=CARTESIAN_POINT('Ctrl Pts',(68.98198486993,9.30957845371409,41.0546881358325));
#162278=CARTESIAN_POINT('Ctrl Pts',(68.3896824371748,9.23219686380711,41.1703037704086));
#162279=CARTESIAN_POINT('Ctrl Pts',(68.0717424362089,9.17315627498059,41.2322836262543));
#162280=CARTESIAN_POINT('Ctrl Pts',(67.5314335830362,9.04248126521768,41.3379612574257));
#162281=CARTESIAN_POINT('Ctrl Pts',(67.307453715784,8.97906360597333,41.3818733041484));
#162282=CARTESIAN_POINT('Ctrl Pts',(66.9165438949958,8.85188805446307,41.4588234670683));
#162283=CARTESIAN_POINT('Ctrl Pts',(66.7486086226193,8.79170730855993,41.4919852804684));
#162284=CARTESIAN_POINT('Ctrl Pts',(66.4858255752121,8.68867584306493,41.5440724303199));
#162285=CARTESIAN_POINT('Ctrl Pts',(66.3897763281541,8.649097660121,41.5631529198949));
#162286=CARTESIAN_POINT('Ctrl Pts',(66.2060868028911,8.56968420014094,41.599729040958));
#162287=CARTESIAN_POINT('Ctrl Pts',(66.118360409311,8.53008830381383,41.617235444182));
#162288=CARTESIAN_POINT('Ctrl Pts',(65.9099737435583,8.43200938982037,41.6589141325978));
#162289=CARTESIAN_POINT('Ctrl Pts',(65.7899329061692,8.37222704278713,41.6829997361007));
#162290=CARTESIAN_POINT('Ctrl Pts',(65.2353359813671,8.08052596148171,41.794630324685));
#162291=CARTESIAN_POINT('Ctrl Pts',(64.8183762964761,7.81596655159606,41.8796375943263));
#162292=CARTESIAN_POINT('Ctrl Pts',(64.2390400466742,7.37892670577032,41.9986703968613));
#162293=CARTESIAN_POINT('Ctrl Pts',(64.0590538096989,7.23210626661684,42.0357882634628));
#162294=CARTESIAN_POINT('Ctrl Pts',(63.7758740932747,6.98267224975432,42.0942588696114));
#162295=CARTESIAN_POINT('Ctrl Pts',(63.6692877269016,6.88422435624125,42.1162838594886));
#162296=CARTESIAN_POINT('Ctrl Pts',(63.5175972045893,6.73734562877,42.1476136584239));
#162297=CARTESIAN_POINT('Ctrl Pts',(63.4706641079982,6.69091765362099,42.157304812156));
#162298=CARTESIAN_POINT('Ctrl Pts',(63.3852099008563,6.6045555049851,42.1749406313875));
#162299=CARTESIAN_POINT('Ctrl Pts',(63.3465467821001,6.5647734896311,42.1829155949898));
#162300=CARTESIAN_POINT('Ctrl Pts',(63.2501005873297,6.46373696636497,42.2028019537123));
#162301=CARTESIAN_POINT('Ctrl Pts',(63.1927807225319,6.40202806366682,42.2146144594204));
#162302=CARTESIAN_POINT('Ctrl Pts',(62.8272543062874,5.99760384790865,42.2899451208317));
#162303=CARTESIAN_POINT('Ctrl Pts',(62.543649714219,5.63261093300959,42.3484333324682));
#162304=CARTESIAN_POINT('Ctrl Pts',(62.1420331183813,5.02774263907562,42.4328086790844));
#162305=CARTESIAN_POINT('Ctrl Pts',(62.0053609601948,4.80164466135541,42.4618727877515));
#162306=CARTESIAN_POINT('Ctrl Pts',(61.7866246874071,4.40246068513886,42.5092344231956));
#162307=CARTESIAN_POINT('Ctrl Pts',(61.6999817838396,4.23216389745481,42.5282697850598));
#162308=CARTESIAN_POINT('Ctrl Pts',(61.573144348026,3.96275762328901,42.5566329724457));
#162309=CARTESIAN_POINT('Ctrl Pts',(61.5293517709636,3.86546226367517,42.5665313361969));
#162310=CARTESIAN_POINT('Ctrl Pts',(61.4489556442168,3.67837096629996,42.5849175723739));
#162311=CARTESIAN_POINT('Ctrl Pts',(61.4120661141639,3.58871764701531,42.5934503782447));
#162312=CARTESIAN_POINT('Ctrl Pts',(61.3283583596253,3.37596884883982,42.6130508845828));
#162313=CARTESIAN_POINT('Ctrl Pts',(61.2827220644023,3.25241363197094,42.623930598713));
#162314=CARTESIAN_POINT('Ctrl Pts',(61.1119531865601,2.75835602231826,42.6654542945684));
#162315=CARTESIAN_POINT('Ctrl Pts',(61.007311672445,2.38092439142235,42.6928295986166));
#162316=CARTESIAN_POINT('Ctrl Pts',(60.8625199054283,1.69582235897097,42.7346205667345));
#162317=CARTESIAN_POINT('Ctrl Pts',(60.8134966288011,1.39070650910709,42.7505217647879));
#162318=CARTESIAN_POINT('Ctrl Pts',(60.7605733240106,0.913645047299086,
42.7709375909532));
#162319=CARTESIAN_POINT('Ctrl Pts',(60.7463087668312,0.743151767111156,
42.7773610088435));
#162320=CARTESIAN_POINT('Ctrl Pts',(60.7299096178347,0.453262157829723,
42.7867375302493));
#162321=CARTESIAN_POINT('Ctrl Pts',(60.7254110672388,0.334056823156275,
42.7901514675776));
#162322=CARTESIAN_POINT('Ctrl Pts',(60.7220203171114,0.155197480335001,
42.7945890807405));
#162323=CARTESIAN_POINT('Ctrl Pts',(60.7214492321599,0.0955957775431189,
42.7959538955453));
#162324=CARTESIAN_POINT('Ctrl Pts',(60.7214339163937,0.0239934614096055,
42.7974542391796));
#162325=CARTESIAN_POINT('Ctrl Pts',(60.7214539679052,0.0119967102410532,
42.7977009207848));
#162326=CARTESIAN_POINT('Ctrl Pts',(60.7214966333422,6.81868220864142E-10,
42.7979428885072));
#162327=CARTESIAN_POINT('Origin',(69.6316151486327,0.,39.48523201752));
#162328=CARTESIAN_POINT('',(60.959339991465,-1.57574869447161E-5,44.1468196011651));
#162329=CARTESIAN_POINT('',(60.929874446542,4.05628901510058E-10,43.9797121921192));
#162330=CARTESIAN_POINT('',(60.4236626579685,-1.14504475720278E-15,41.1088424787055));
#162331=CARTESIAN_POINT('Ctrl Pts',(60.9593399353935,-7.19695824888743E-14,
44.1468192833488));
#162332=CARTESIAN_POINT('Ctrl Pts',(60.9592011695234,0.039018323097806,
44.1460323029926));
#162333=CARTESIAN_POINT('Ctrl Pts',(60.9593042464182,0.0780364129096037,
44.1452103586968));
#162334=CARTESIAN_POINT('Ctrl Pts',(60.9600768192033,0.165455973684423,
44.1432889493377));
#162335=CARTESIAN_POINT('Ctrl Pts',(60.9608766338813,0.213854746414297,
44.142170326208));
#162336=CARTESIAN_POINT('Ctrl Pts',(60.9649924384163,0.383848718732972,
44.1380441549837));
#162337=CARTESIAN_POINT('Ctrl Pts',(60.9702840870665,0.505376432410811,
44.1347397851575));
#162338=CARTESIAN_POINT('Ctrl Pts',(61.0103947725256,1.14324184570811,44.1154304296644));
#162339=CARTESIAN_POINT('Ctrl Pts',(61.0851820544867,1.65595956485757,44.0930853775808));
#162340=CARTESIAN_POINT('Ctrl Pts',(61.254417884048,2.38999330760417,44.0493671991483));
#162341=CARTESIAN_POINT('Ctrl Pts',(61.3161166739917,2.61819672159879,44.0340696663355));
#162342=CARTESIAN_POINT('Ctrl Pts',(61.4399886201481,3.01653157258925,44.0042054564054));
#162343=CARTESIAN_POINT('Ctrl Pts',(61.4986480887534,3.18767454757481,43.9903119054966));
#162344=CARTESIAN_POINT('Ctrl Pts',(61.5991309158904,3.45551078176694,43.9668426511835));
#162345=CARTESIAN_POINT('Ctrl Pts',(61.6377411246449,3.55341421144728,43.9578902120456));
#162346=CARTESIAN_POINT('Ctrl Pts',(61.7152321514134,3.74066451952898,43.9400397506919));
#162347=CARTESIAN_POINT('Ctrl Pts',(61.7538779760383,3.83009807721125,43.9311875769518));
#162348=CARTESIAN_POINT('Ctrl Pts',(61.849622853789,4.04255604396231,43.909370681766));
#162349=CARTESIAN_POINT('Ctrl Pts',(61.9079976324839,4.1649553813899,43.8961584742693));
#162350=CARTESIAN_POINT('Ctrl Pts',(62.1929017806195,4.73051438383986,43.8320819235754));
#162351=CARTESIAN_POINT('Ctrl Pts',(62.4514798570855,5.15590401043427,43.7750015130925));
#162352=CARTESIAN_POINT('Ctrl Pts',(62.8789950099589,5.747109625867,43.6827388275413));
#162353=CARTESIAN_POINT('Ctrl Pts',(63.0226635000979,5.93080520324176,43.6520248084645));
#162354=CARTESIAN_POINT('Ctrl Pts',(63.2668461916425,6.21983386012601,43.6004304954048));
#162355=CARTESIAN_POINT('Ctrl Pts',(63.3632454332833,6.32862494160068,43.580201788264));
#162356=CARTESIAN_POINT('Ctrl Pts',(63.507108474567,6.48345064180576,43.5502522051747));
#162357=CARTESIAN_POINT('Ctrl Pts',(63.5525889486014,6.53135348063232,43.5408171906781));
#162358=CARTESIAN_POINT('Ctrl Pts',(63.6371998643254,6.61857180536192,43.5233300685671));
#162359=CARTESIAN_POINT('Ctrl Pts',(63.6761795625054,6.65803240109385,43.515299282958));
#162360=CARTESIAN_POINT('Ctrl Pts',(63.7751887497777,6.75646676911935,43.4949609943681));
#162361=CARTESIAN_POINT('Ctrl Pts',(63.8356686779449,6.81496719119529,43.4825912797514));
#162362=CARTESIAN_POINT('Ctrl Pts',(64.2320895852908,7.18802242331507,43.4018130582296));
#162363=CARTESIAN_POINT('Ctrl Pts',(64.5900881648394,7.47747545171792,43.3302071586913));
#162364=CARTESIAN_POINT('Ctrl Pts',(65.1834487745134,7.88764202051685,43.2120221629778));
#162365=CARTESIAN_POINT('Ctrl Pts',(65.4052619474988,8.02728413330826,43.1679454138692));
#162366=CARTESIAN_POINT('Ctrl Pts',(65.7968766236401,8.25092076888774,43.0901006780881));
#162367=CARTESIAN_POINT('Ctrl Pts',(65.963943210823,8.33955259322519,43.0568844591762));
#162368=CARTESIAN_POINT('Ctrl Pts',(66.2282303761327,8.46938804728209,43.0042851860022));
#162369=CARTESIAN_POINT('Ctrl Pts',(66.3236753258305,8.51423411021166,42.9852791167078));
#162370=CARTESIAN_POINT('Ctrl Pts',(66.5072042527139,8.59660154086896,42.948707786122));
#162371=CARTESIAN_POINT('Ctrl Pts',(66.5951487187156,8.63441234394498,42.931172616974));
#162372=CARTESIAN_POINT('Ctrl Pts',(66.8038377792478,8.7202520367896,42.8895345299687));
#162373=CARTESIAN_POINT('Ctrl Pts',(66.9250316375695,8.76708430385657,42.8653319749979));
#162374=CARTESIAN_POINT('Ctrl Pts',(67.4096410303131,8.9424726197836,42.7684695094921));
#162375=CARTESIAN_POINT('Ctrl Pts',(67.7798219999628,9.0502801333161,42.6942721995562));
#162376=CARTESIAN_POINT('Ctrl Pts',(68.4518378808896,9.20014966751034,42.5595149072701));
#162377=CARTESIAN_POINT('Ctrl Pts',(68.7511721451292,9.25119965452689,42.4994748235487));
#162378=CARTESIAN_POINT('Ctrl Pts',(69.2191269334297,9.30685182060255,42.4058770748503));
#162379=CARTESIAN_POINT('Ctrl Pts',(69.3863020010349,9.3220054585555,42.3724928759089));
#162380=CARTESIAN_POINT('Ctrl Pts',(69.6705900515395,9.33977388874443,42.315882417577));
#162381=CARTESIAN_POINT('Ctrl Pts',(69.7875076349303,9.34479450278586,42.292646642121));
#162382=CARTESIAN_POINT('Ctrl Pts',(69.96295926624,9.34890258724526,42.2578708185383));
#162383=CARTESIAN_POINT('Ctrl Pts',(70.0214341345616,9.34970165889319,42.2462961240143));
#162384=CARTESIAN_POINT('Ctrl Pts',(70.130812587057,9.35013033751004,42.2246782297245));
#162385=CARTESIAN_POINT('Ctrl Pts',(70.1817120289497,9.34989817211438,42.2146320107093));
#162386=CARTESIAN_POINT('Ctrl Pts',(70.3095209877298,9.34823134452351,42.1894372159126));
#162387=CARTESIAN_POINT('Ctrl Pts',(70.3864226536441,9.34624277031949,42.1743059193247));
#162388=CARTESIAN_POINT('Ctrl Pts',(70.7370584013524,9.33267907523359,42.1054179630285));
#162389=CARTESIAN_POINT('Ctrl Pts',(71.010272020692,9.30960232183055,42.0520262675107));
#162390=CARTESIAN_POINT('Ctrl Pts',(71.6023944059914,9.23227640381724,41.9364456131107));
#162391=CARTESIAN_POINT('Ctrl Pts',(71.9203369568101,9.17325292138672,41.8744653373229));
#162392=CARTESIAN_POINT('Ctrl Pts',(72.4607344914445,9.04258707399007,41.7687706979663));
#162393=CARTESIAN_POINT('Ctrl Pts',(72.6847984548984,8.9791551477307,41.724842325927));
#162394=CARTESIAN_POINT('Ctrl Pts',(73.0758333745289,8.85194986191113,41.6478677410431));
#162395=CARTESIAN_POINT('Ctrl Pts',(73.2438106486876,8.7917575038101,41.614697707368));
#162396=CARTESIAN_POINT('Ctrl Pts',(73.5066424323439,8.68871024668405,41.5626009701187));
#162397=CARTESIAN_POINT('Ctrl Pts',(73.6026991740363,8.64913006096221,41.5435190163316));
#162398=CARTESIAN_POINT('Ctrl Pts',(73.7863936891685,8.56971627136852,41.5069419436213));
#162399=CARTESIAN_POINT('Ctrl Pts',(73.8741177145433,8.53012238079545,41.4894360347551));
#162400=CARTESIAN_POINT('Ctrl Pts',(74.0824832998574,8.43205577105438,41.4477616179529));
#162401=CARTESIAN_POINT('Ctrl Pts',(74.2025057982643,8.37228448625142,41.4236797390816));
#162402=CARTESIAN_POINT('Ctrl Pts',(74.7573559309023,8.08046183613628,41.3119984478771));
#162403=CARTESIAN_POINT('Ctrl Pts',(75.1745635785788,7.81572557180448,41.2269400662472));
#162404=CARTESIAN_POINT('Ctrl Pts',(75.7539753321687,7.37855356386901,41.1078908311994));
#162405=CARTESIAN_POINT('Ctrl Pts',(75.9338262791899,7.23182678448237,41.0708007567995));
#162406=CARTESIAN_POINT('Ctrl Pts',(76.21682939966,6.98253378605796,41.0123665601668));
#162407=CARTESIAN_POINT('Ctrl Pts',(76.3233685760332,6.88412576028209,40.990351324461));
#162408=CARTESIAN_POINT('Ctrl Pts',(76.4750066279395,6.73729525527626,40.9590323686953));
#162409=CARTESIAN_POINT('Ctrl Pts',(76.5219326386913,6.69087361687547,40.949342680837));
#162410=CARTESIAN_POINT('Ctrl Pts',(76.6073814114384,6.60451597538701,40.9317079882756));
#162411=CARTESIAN_POINT('Ctrl Pts',(76.6460460110928,6.56473195083532,40.9237327221797));
#162412=CARTESIAN_POINT('Ctrl Pts',(76.7425062464142,6.46367940418966,40.9038434734586));
#162413=CARTESIAN_POINT('Ctrl Pts',(76.7998383351589,6.40195616116632,40.8920284514729));
#162414=CARTESIAN_POINT('Ctrl Pts',(77.1654414559112,5.99743685202562,40.8166819796699));
#162415=CARTESIAN_POINT('Ctrl Pts',(77.4490991356294,5.63235364864955,40.7581826986619));
#162416=CARTESIAN_POINT('Ctrl Pts',(77.8507003742193,5.0274484261585,40.6738095502626));
#162417=CARTESIAN_POINT('Ctrl Pts',(77.987322929437,4.80141585042249,40.6447556328777));
#162418=CARTESIAN_POINT('Ctrl Pts',(78.2059947350294,4.40233107207008,40.5974075410352));
#162419=CARTESIAN_POINT('Ctrl Pts',(78.2926188081794,4.23206554937768,40.5783761765879));
#162420=CARTESIAN_POINT('Ctrl Pts',(78.4194360519795,3.96269671506524,40.5500173702641));
#162421=CARTESIAN_POINT('Ctrl Pts',(78.4632254749425,3.86540659021672,40.540119674957));
#162422=CARTESIAN_POINT('Ctrl Pts',(78.5436188144636,3.67831876442622,40.521733999986));
#162423=CARTESIAN_POINT('Ctrl Pts',(78.5805084727915,3.5886635725035,40.5132011246697));
#162424=CARTESIAN_POINT('Ctrl Pts',(78.664220606108,3.37589964412092,40.4935994907015));
#162425=CARTESIAN_POINT('Ctrl Pts',(78.7098606565591,3.25233098193822,40.4827187971432));
#162426=CARTESIAN_POINT('Ctrl Pts',(78.8808972116723,2.75748157894577,40.4411295694266));
#162427=CARTESIAN_POINT('Ctrl Pts',(78.9857056668484,2.37923964034732,40.4137051318709));
#162428=CARTESIAN_POINT('Ctrl Pts',(79.1313804155078,1.68903248615976,40.3716372015968));
#162429=CARTESIAN_POINT('Ctrl Pts',(79.1807987374525,1.37955890879548,40.3555626438913));
#162430=CARTESIAN_POINT('Ctrl Pts',(79.2330867746745,0.901036399115497,
40.3352341776319));
#162431=CARTESIAN_POINT('Ctrl Pts',(79.2469061362153,0.733496976087364,
40.3289604461154));
#162432=CARTESIAN_POINT('Ctrl Pts',(79.2628557554179,0.447992296191848,
40.3197654258101));
#162433=CARTESIAN_POINT('Ctrl Pts',(79.2672442328512,0.330207732233258,
40.3164035776742));
#162434=CARTESIAN_POINT('Ctrl Pts',(79.2705580195277,0.153029291306634,
40.3120168654863));
#162435=CARTESIAN_POINT('Ctrl Pts',(79.2711139470456,0.0936857360576762,
40.310660576402));
#162436=CARTESIAN_POINT('Ctrl Pts',(79.2711184696487,-0.0170278165458702,
40.3083446807105));
#162437=CARTESIAN_POINT('Ctrl Pts',(79.2707059962099,-0.068394340316024,
40.3073566946874));
#162438=CARTESIAN_POINT('Ctrl Pts',(79.2686159971758,-0.198164504203468,
40.3050762702276));
#162439=CARTESIAN_POINT('Ctrl Pts',(79.2663867249648,-0.276557334706842,
40.3038972866039));
#162440=CARTESIAN_POINT('Ctrl Pts',(79.2518252935275,-0.63355012053469,
40.2994091240156));
#162441=CARTESIAN_POINT('Ctrl Pts',(79.2282409446322,-0.911575433521893,
40.2983564799344));
#162442=CARTESIAN_POINT('Ctrl Pts',(79.1502650954314,-1.51447011944969,
40.3009375815794));
#162443=CARTESIAN_POINT('Ctrl Pts',(79.0911512195368,-1.83834904805255,
40.3054425701453));
#162444=CARTESIAN_POINT('Ctrl Pts',(78.9607036614042,-2.38902455281903,
40.318033982787));
#162445=CARTESIAN_POINT('Ctrl Pts',(78.8974583286698,-2.61743978298294,
40.3247637682565));
#162446=CARTESIAN_POINT('Ctrl Pts',(78.7707692099646,-3.01608976400974,
40.3390743896039));
#162447=CARTESIAN_POINT('Ctrl Pts',(78.7108668480139,-3.18733854012721,
40.346084475152));
#162448=CARTESIAN_POINT('Ctrl Pts',(78.608378047351,-3.45529755884479,40.3584021377836));
#162449=CARTESIAN_POINT('Ctrl Pts',(78.5690294674324,-3.55321986489301,
40.3631955836433));
#162450=CARTESIAN_POINT('Ctrl Pts',(78.4901056668316,-3.7404827377327,40.3729250988388));
#162451=CARTESIAN_POINT('Ctrl Pts',(78.4507677608816,-3.82991032402126,
40.3778237504992));
#162452=CARTESIAN_POINT('Ctrl Pts',(78.3533653589933,-4.04231517080979,
40.3900653020223));
#162453=CARTESIAN_POINT('Ctrl Pts',(78.2940192915613,-4.16466829028765,
40.3976116688886));
#162454=CARTESIAN_POINT('Ctrl Pts',(78.0040853101993,-4.7308609468423,40.4348797324491));
#162455=CARTESIAN_POINT('Ctrl Pts',(77.7411480921919,-5.15687198280501,
40.4697383963746));
#162456=CARTESIAN_POINT('Ctrl Pts',(77.3075384551055,-5.74826772979273,
40.5293075740135));
#162457=CARTESIAN_POINT('Ctrl Pts',(77.1622572267894,-5.93162484066259,
40.5495528383983));
#162458=CARTESIAN_POINT('Ctrl Pts',(76.9154969969459,-6.22021157404352,
40.5845379323153));
#162459=CARTESIAN_POINT('Ctrl Pts',(76.8180896171305,-6.32888451799664,
40.5984860770007));
#162460=CARTESIAN_POINT('Ctrl Pts',(76.6727763691276,-6.48357885542733,
40.6195299788531));
#162461=CARTESIAN_POINT('Ctrl Pts',(76.6268271397286,-6.53146394911662,
40.6262170189577));
#162462=CARTESIAN_POINT('Ctrl Pts',(76.5413488926385,-6.6186686696494,40.6387216184551));
#162463=CARTESIAN_POINT('Ctrl Pts',(76.5019683888374,-6.65813297853069,
40.6445077489881));
#162464=CARTESIAN_POINT('Ctrl Pts',(76.401935159927,-6.7566025323501,40.6592649914099));
#162465=CARTESIAN_POINT('Ctrl Pts',(76.3408370992651,-6.81513358485769,
40.668331870445));
#162466=CARTESIAN_POINT('Ctrl Pts',(75.9404576245387,-7.18838755013565,
40.7280452531935));
#162467=CARTESIAN_POINT('Ctrl Pts',(75.579331378679,-7.47797909636203,40.7832361062152));
#162468=CARTESIAN_POINT('Ctrl Pts',(74.9812390012199,-7.88810805242604,
40.8751350827215));
#162469=CARTESIAN_POINT('Ctrl Pts',(74.7578907282277,-8.02762250909813,
40.9095559514904));
#162470=CARTESIAN_POINT('Ctrl Pts',(74.3635161713318,-8.25109308977263,
40.9703078130127));
#162471=CARTESIAN_POINT('Ctrl Pts',(74.1952422766827,-8.33967638575718,
40.9962228767871));
#162472=CARTESIAN_POINT('Ctrl Pts',(73.9289969291622,-8.46945975931981,
41.0371728699192));
#162473=CARTESIAN_POINT('Ctrl Pts',(73.8328206092398,-8.51429769320179,
41.0519550838115));
#162474=CARTESIAN_POINT('Ctrl Pts',(73.6478603502723,-8.59665795442987,
41.0803585146401));
#162475=CARTESIAN_POINT('Ctrl Pts',(73.5592175271624,-8.63446910770138,
41.0939603307918));
#162476=CARTESIAN_POINT('Ctrl Pts',(73.3488351292313,-8.72032017982404,
41.126214951365));
#162477=CARTESIAN_POINT('Ctrl Pts',(73.2266388362571,-8.76716221030664,
41.1449278460924));
#162478=CARTESIAN_POINT('Ctrl Pts',(72.7360783828904,-8.94327028018312,
41.2199661886711));
#162479=CARTESIAN_POINT('Ctrl Pts',(72.360747672531,-9.05153031441586,41.2771711454197));
#162480=CARTESIAN_POINT('Ctrl Pts',(71.6146438540337,-9.21598828431424,
41.3908216282327));
#162481=CARTESIAN_POINT('Ctrl Pts',(71.2450113648896,-9.27401177106631,
41.447099671287));
#162482=CARTESIAN_POINT('Ctrl Pts',(70.7426216104471,-9.32160373129045,
41.5240315512877));
#162483=CARTESIAN_POINT('Ctrl Pts',(70.6120254932216,-9.33115048055859,
41.5440714544694));
#162484=CARTESIAN_POINT('Ctrl Pts',(70.3828688479151,-9.34296033891395,
41.5793431138487));
#162485=CARTESIAN_POINT('Ctrl Pts',(70.2843862065223,-9.34644002596292,
41.594536333219));
#162486=CARTESIAN_POINT('Ctrl Pts',(70.1306539582927,-9.34938334255177,
41.6183219194453));
#162487=CARTESIAN_POINT('Ctrl Pts',(70.0754274562202,-9.3499397919804,41.6268804792593));
#162488=CARTESIAN_POINT('Ctrl Pts',(69.967001283541,-9.35004891768843,41.6437140900858));
#162489=CARTESIAN_POINT('Ctrl Pts',(69.9138038303237,-9.34963765444814,
41.6519878485647));
#162490=CARTESIAN_POINT('Ctrl Pts',(69.7722524177475,-9.34730628279,41.6740374694986));
#162491=CARTESIAN_POINT('Ctrl Pts',(69.6839204605119,-9.34456834027643,
41.6878325046681));
#162492=CARTESIAN_POINT('Ctrl Pts',(69.0699080624955,-9.31660839460732,
41.783915356157));
#162493=CARTESIAN_POINT('Ctrl Pts',(68.5473011312671,-9.2472547137258,41.8666207186992));
#162494=CARTESIAN_POINT('Ctrl Pts',(67.7349761655645,-9.06706731850457,
41.9944599117333));
#162495=CARTESIAN_POINT('Ctrl Pts',(67.4400676372568,-8.98596589100186,
42.0407264249616));
#162496=CARTESIAN_POINT('Ctrl Pts',(66.9887198190538,-8.83719921088504,
42.1110580656074));
#162497=CARTESIAN_POINT('Ctrl Pts',(66.8292750783789,-8.77970378497714,
42.135809458165));
#162498=CARTESIAN_POINT('Ctrl Pts',(66.5758089277539,-8.68029706657569,
42.174979317466));
#162499=CARTESIAN_POINT('Ctrl Pts',(66.4807725337071,-8.64117421924204,
42.1896252236292));
#162500=CARTESIAN_POINT('Ctrl Pts',(66.2977087275427,-8.56220138001157,
42.2177540394568));
#162501=CARTESIAN_POINT('Ctrl Pts',(66.2096157750666,-8.52254263413246,
42.2312520650165));
#162502=CARTESIAN_POINT('Ctrl Pts',(65.9957402744897,-8.42218178350809,
42.2639285618215));
#162503=CARTESIAN_POINT('Ctrl Pts',(65.8706636723969,-8.35998373123995,
42.2829566136051));
#162504=CARTESIAN_POINT('Ctrl Pts',(65.3979336301034,-8.11135839340803,
42.3545672359968));
#162505=CARTESIAN_POINT('Ctrl Pts',(65.0606918978997,-7.90542798625243,
42.404989099112));
#162506=CARTESIAN_POINT('Ctrl Pts',(64.4958575449963,-7.50883378545272,
42.4886322787441));
#162507=CARTESIAN_POINT('Ctrl Pts',(64.2624272784163,-7.32770944102872,
42.5229369039794));
#162508=CARTESIAN_POINT('Ctrl Pts',(63.9111985396855,-7.02726604484864,
42.5744104081198));
#162509=CARTESIAN_POINT('Ctrl Pts',(63.7873850613468,-6.91544450915314,
42.5925266911494));
#162510=CARTESIAN_POINT('Ctrl Pts',(63.6164183557497,-6.75246344023828,
42.6175586793641));
#162511=CARTESIAN_POINT('Ctrl Pts',(63.566750732155,-6.70404297060807,42.6248328376538));
#162512=CARTESIAN_POINT('Ctrl Pts',(63.4785454997894,-6.61610480969267,
42.6377606610672));
#162513=CARTESIAN_POINT('Ctrl Pts',(63.4398115464697,-6.57679402993487,
42.6434416580011));
#162514=CARTESIAN_POINT('Ctrl Pts',(63.3461377269486,-6.48001660749793,
42.6571882414878));
#162515=CARTESIAN_POINT('Ctrl Pts',(63.2915768659843,-6.42218239615651,
42.6652009766809));
#162516=CARTESIAN_POINT('Ctrl Pts',(63.0599241657975,-6.17024356202669,
42.6992227941961));
#162517=CARTESIAN_POINT('Ctrl Pts',(62.8902769064617,-5.96931395311664,
42.724139896814));
#162518=CARTESIAN_POINT('Ctrl Pts',(62.4838819974151,-5.44462052743962,
42.7833655164531));
#162519=CARTESIAN_POINT('Ctrl Pts',(62.2589369410372,-5.11218034067375,
42.815685340908));
#162520=CARTESIAN_POINT('Ctrl Pts',(61.9972718356034,-4.66662169017116,
42.8520069343839));
#162521=CARTESIAN_POINT('Ctrl Pts',(61.9406433965693,-4.56601005140854,
42.8597783710209));
#162522=CARTESIAN_POINT('Ctrl Pts',(61.8058414933842,-4.3158824332008,42.8780324809005));
#162523=CARTESIAN_POINT('Ctrl Pts',(61.72978913071,-4.16524104560711,42.8881105987113));
#162524=CARTESIAN_POINT('Ctrl Pts',(61.6138154578883,-3.91939315977447,
42.9030775538707));
#162525=CARTESIAN_POINT('Ctrl Pts',(61.5713625944114,-3.82545359404603,
42.9084583018507));
#162526=CARTESIAN_POINT('Ctrl Pts',(61.4916526128767,-3.6411126093075,42.9183589384919));
#162527=CARTESIAN_POINT('Ctrl Pts',(61.4542451361088,-3.55079225944025,
42.9229084115732));
#162528=CARTESIAN_POINT('Ctrl Pts',(61.3657429971548,-3.3273940142231,42.933422675009));
#162529=CARTESIAN_POINT('Ctrl Pts',(61.3162337686272,-3.19370041539068,
42.939080352518));
#162530=CARTESIAN_POINT('Ctrl Pts',(61.0655530653476,-2.46690118480169,
42.9664486156816));
#162531=CARTESIAN_POINT('Ctrl Pts',(60.9202954310094,-1.85578835661807,
42.9773142197201));
#162532=CARTESIAN_POINT('Ctrl Pts',(60.7968252928583,-0.94261981963765,
42.9777153545758));
#162533=CARTESIAN_POINT('Ctrl Pts',(60.7709605078862,-0.648742537193085,
42.9755204946933));
#162534=CARTESIAN_POINT('Ctrl Pts',(60.7556501642509,-0.275929395564813,
42.9700738771766));
#162535=CARTESIAN_POINT('Ctrl Pts',(60.7534089544413,-0.197654762270246,
42.968782577162));
#162536=CARTESIAN_POINT('Ctrl Pts',(60.7514966309874,-0.0795781893991349,
42.9666186679888));
#162537=CARTESIAN_POINT('Ctrl Pts',(60.751103630633,-0.0397894807063568,
42.965852513959));
#162538=CARTESIAN_POINT('Ctrl Pts',(60.7509621221957,-6.89336955246539E-10,
42.9650499797481));
#162539=CARTESIAN_POINT('Ctrl Pts',(60.7214966333422,6.81868220864142E-10,
42.7979428885072));
#162540=CARTESIAN_POINT('Ctrl Pts',(60.7216384344148,-0.0398717644279405,
42.7987470823689));
#162541=CARTESIAN_POINT('Ctrl Pts',(60.7220300289147,-0.0797430699037861,
42.7994992074081));
#162542=CARTESIAN_POINT('Ctrl Pts',(60.7239324241189,-0.197976095297675,
42.8015772606206));
#162543=CARTESIAN_POINT('Ctrl Pts',(60.7261587264108,-0.276325270394438,
42.8027559393475));
#162544=CARTESIAN_POINT('Ctrl Pts',(60.7407282582848,-0.633770612581696,
42.8072518609236));
#162545=CARTESIAN_POINT('Ctrl Pts',(60.7643682793433,-0.912290023609129,
42.8083035643672));
#162546=CARTESIAN_POINT('Ctrl Pts',(60.842484874372,-1.51566812981762,42.8057061943277));
#162547=CARTESIAN_POINT('Ctrl Pts',(60.9016403944183,-1.83954063114414,
42.801193935115));
#162548=CARTESIAN_POINT('Ctrl Pts',(61.0321096736188,-2.38999291230631,
42.7885953017863));
#162549=CARTESIAN_POINT('Ctrl Pts',(61.0953196500395,-2.61819641270663,
42.7818680504721));
#162550=CARTESIAN_POINT('Ctrl Pts',(61.2219353950757,-3.01653139225999,
42.7675645244941));
#162551=CARTESIAN_POINT('Ctrl Pts',(61.2818091508149,-3.18767441041751,
42.7605574706621));
#162552=CARTESIAN_POINT('Ctrl Pts',(61.3842590955769,-3.45551069471278,
42.7482442030221));
#162553=CARTESIAN_POINT('Ctrl Pts',(61.423602740362,-3.5534141320965,42.7434512746748));
#162554=CARTESIAN_POINT('Ctrl Pts',(61.5025257040829,-3.74066444530087,
42.7337217294173));
#162555=CARTESIAN_POINT('Ctrl Pts',(61.5418685200311,-3.8300980005415,42.7288224015581));
#162556=CARTESIAN_POINT('Ctrl Pts',(61.6393010804231,-4.04255594558835,
42.7165769017754));
#162557=CARTESIAN_POINT('Ctrl Pts',(61.6986742592231,-4.16495526413319,
42.7090269669468));
#162558=CARTESIAN_POINT('Ctrl Pts',(61.9883121783848,-4.73051452830085,
42.6717962557641));
#162559=CARTESIAN_POINT('Ctrl Pts',(62.2508189167381,-5.15590441137969,
42.6369953616465));
#162560=CARTESIAN_POINT('Ctrl Pts',(62.684107580498,-5.74711010491705,42.5774751123864));
#162561=CARTESIAN_POINT('Ctrl Pts',(62.8296165194742,-5.93080554222332,
42.5571993445042));
#162562=CARTESIAN_POINT('Ctrl Pts',(63.0767193453967,-6.21983401626779,
42.5221667602561));
#162563=CARTESIAN_POINT('Ctrl Pts',(63.1742235866626,-6.32862504888967,
42.5082050502534));
#162564=CARTESIAN_POINT('Ctrl Pts',(63.3196539372216,-6.48345069477836,
42.4871444014065));
#162565=CARTESIAN_POINT('Ctrl Pts',(63.365618561706,-6.53135352627038,42.4804551775611));
#162566=CARTESIAN_POINT('Ctrl Pts',(63.4511077583279,-6.61857184537218,
42.4679490602732));
#162567=CARTESIAN_POINT('Ctrl Pts',(63.4904833855244,-6.65803244263412,
42.462163687978));
#162568=CARTESIAN_POINT('Ctrl Pts',(63.5904777086381,-6.75646682518263,
42.4474122888511));
#162569=CARTESIAN_POINT('Ctrl Pts',(63.6515409567846,-6.81496725990258,
42.4383506625284));
#162570=CARTESIAN_POINT('Ctrl Pts',(64.0516826306627,-7.18802256978761,
42.3786734114279));
#162571=CARTESIAN_POINT('Ctrl Pts',(64.4125820026368,-7.47747565181252,
42.3235182074294));
#162572=CARTESIAN_POINT('Ctrl Pts',(65.0105802740117,-7.88764220478509,
42.2316344892034));
#162573=CARTESIAN_POINT('Ctrl Pts',(65.2340915474207,-8.02728426708803,
42.1971885218025));
#162574=CARTESIAN_POINT('Ctrl Pts',(65.6287133386676,-8.25092083700116,
42.1363985529957));
#162575=CARTESIAN_POINT('Ctrl Pts',(65.7970651629551,-8.33955264215256,
42.1104714554637));
#162576=CARTESIAN_POINT('Ctrl Pts',(66.063403836005,-8.46938807562017,42.0695070758555));
#162577=CARTESIAN_POINT('Ctrl Pts',(66.1595932043114,-8.51423413533653,
42.0547228443441));
#162578=CARTESIAN_POINT('Ctrl Pts',(66.34456211091,-8.59660156315883,42.0263180644849));
#162579=CARTESIAN_POINT('Ctrl Pts',(66.4332002595621,-8.63441236637256,
42.012716954392));
#162580=CARTESIAN_POINT('Ctrl Pts',(66.6435449091828,-8.72025206371114,
41.9804680928254));
#162581=CARTESIAN_POINT('Ctrl Pts',(66.7657076581063,-8.76708433463439,
41.9617603123215));
#162582=CARTESIAN_POINT('Ctrl Pts',(67.2542212081322,-8.9424729192846,41.887034965394));
#162583=CARTESIAN_POINT('Ctrl Pts',(67.6274552913591,-9.05028060184344,
41.8301481628908));
#162584=CARTESIAN_POINT('Ctrl Pts',(68.3050418504365,-9.20015181988067,
41.7269343355587));
#162585=CARTESIAN_POINT('Ctrl Pts',(68.6068668020621,-9.25120264826099,
41.6809740186536));
#162586=CARTESIAN_POINT('Ctrl Pts',(69.0786157844767,-9.30685380816212,
41.6088766939587));
#162587=CARTESIAN_POINT('Ctrl Pts',(69.247122100101,-9.32200665805263,41.5830710879211));
#162588=CARTESIAN_POINT('Ctrl Pts',(69.5336200930502,-9.33977428608612,
41.5390363942365));
#162589=CARTESIAN_POINT('Ctrl Pts',(69.6514314265196,-9.34479470213056,
41.5208830735776));
#162590=CARTESIAN_POINT('Ctrl Pts',(69.8281932716483,-9.34890264439575,
41.4935540956125));
#162591=CARTESIAN_POINT('Ctrl Pts',(69.8871000254112,-9.34970168861369,
41.4844312333286));
#162592=CARTESIAN_POINT('Ctrl Pts',(69.997275621315,-9.35013033339449,41.4673358181496));
#162593=CARTESIAN_POINT('Ctrl Pts',(70.0485416037169,-9.34989815091215,
41.459367518842));
#162594=CARTESIAN_POINT('Ctrl Pts',(70.1772609579311,-9.34823126487482,
41.4393294720256));
#162595=CARTESIAN_POINT('Ctrl Pts',(70.2547010417848,-9.34624262758035,
41.4272461720832));
#162596=CARTESIAN_POINT('Ctrl Pts',(70.6077408026198,-9.33267912822794,
41.3720569225812));
#162597=CARTESIAN_POINT('Ctrl Pts',(70.8827266366174,-9.30960375154021,
41.328786045328));
#162598=CARTESIAN_POINT('Ctrl Pts',(71.4786588249724,-9.23228136575298,
41.2348804135636));
#162599=CARTESIAN_POINT('Ctrl Pts',(71.7986257557919,-9.17325895049772,
41.1843800346556));
#162600=CARTESIAN_POINT('Ctrl Pts',(72.342588590483,-9.04259367473654,41.0988727696695));
#162601=CARTESIAN_POINT('Ctrl Pts',(72.5681695109219,-8.97916085839969,
41.0635167103407));
#162602=CARTESIAN_POINT('Ctrl Pts',(72.9619568538091,-8.85195371743119,
41.0021061027598));
#162603=CARTESIAN_POINT('Ctrl Pts',(73.1311513162953,-8.79176063488057,
40.9758237129305));
#162604=CARTESIAN_POINT('Ctrl Pts',(73.3959535992366,-8.68871239253119,
40.9348843903048));
#162605=CARTESIAN_POINT('Ctrl Pts',(73.4927442937574,-8.64913208185471,
40.9199621468301));
#162606=CARTESIAN_POINT('Ctrl Pts',(73.6778710827111,-8.56971827161967,
40.8915060770526));
#162607=CARTESIAN_POINT('Ctrl Pts',(73.7662919262214,-8.53012450610539,
40.8779528882343));
#162608=CARTESIAN_POINT('Ctrl Pts',(73.9763436929254,-8.43205866358636,
40.8458490021002));
#162609=CARTESIAN_POINT('Ctrl Pts',(74.0973632826702,-8.37228806856663,
40.8274286267294));
#162610=CARTESIAN_POINT('Ctrl Pts',(74.6569649524157,-8.080457877396,40.7426023721919));
#162611=CARTESIAN_POINT('Ctrl Pts',(75.0781191308368,-7.81571063575195,
40.6798354029987));
#162612=CARTESIAN_POINT('Ctrl Pts',(75.6633100798418,-7.3785304193032,40.5935339536315));
#162613=CARTESIAN_POINT('Ctrl Pts',(75.8449917672632,-7.23180944833177,
40.5668758260354));
#162614=CARTESIAN_POINT('Ctrl Pts',(76.1309023198231,-6.98252519568258,
40.5249948655329));
#162615=CARTESIAN_POINT('Ctrl Pts',(76.2385430941341,-6.88411964298136,
40.509244308298));
#162616=CARTESIAN_POINT('Ctrl Pts',(76.3917446776339,-6.73729212935453,
40.4868117128442));
#162617=CARTESIAN_POINT('Ctrl Pts',(76.4391543278598,-6.69087088411331,
40.4798674649997));
#162618=CARTESIAN_POINT('Ctrl Pts',(76.525480988506,-6.60451352214671,40.4672135035835));
#162619=CARTESIAN_POINT('Ctrl Pts',(76.5645416220102,-6.5647293728129,40.4614837165617));
#162620=CARTESIAN_POINT('Ctrl Pts',(76.6619879975111,-6.46367583140274,
40.4471820237762));
#162621=CARTESIAN_POINT('Ctrl Pts',(76.7199042802555,-6.40195169814966,
40.4386756707877));
#162622=CARTESIAN_POINT('Ctrl Pts',(77.0892337656632,-5.99742636585881,
40.3844338402149));
#162623=CARTESIAN_POINT('Ctrl Pts',(77.3757961496233,-5.63233742154819,
40.3423880478601));
#162624=CARTESIAN_POINT('Ctrl Pts',(77.7820342517149,-5.02742982705434,
40.284317357488));
#162625=CARTESIAN_POINT('Ctrl Pts',(77.9203513171859,-4.80140138535834,
40.2648919103462));
#162626=CARTESIAN_POINT('Ctrl Pts',(78.142025478371,-4.40232287747439,40.2345949898328));
#162627=CARTESIAN_POINT('Ctrl Pts',(78.2299333856523,-4.23205933128081,
40.2228516143285));
#162628=CARTESIAN_POINT('Ctrl Pts',(78.3588006025984,-3.96269286383592,
40.2061262997943));
#162629=CARTESIAN_POINT('Ctrl Pts',(78.4033342095557,-3.86540306993304,
40.2004502548094));
#162630=CARTESIAN_POINT('Ctrl Pts',(78.4851673309505,-3.6783154635528,40.1902310233285));
#162631=CARTESIAN_POINT('Ctrl Pts',(78.5227506950441,-3.5886601531748,40.185632298419));
#162632=CARTESIAN_POINT('Ctrl Pts',(78.6081188072846,-3.37589526788816,
40.1754205456761));
#162633=CARTESIAN_POINT('Ctrl Pts',(78.6547280866305,-3.2523257553825,40.1700352135047));
#162634=CARTESIAN_POINT('Ctrl Pts',(78.8296919525895,-2.7574251485224,40.1506164171643));
#162635=CARTESIAN_POINT('Ctrl Pts',(78.9375706290344,-2.37913078600191,
40.1405396493626));
#162636=CARTESIAN_POINT('Ctrl Pts',(79.088903231862,-1.68861472449073,40.1302445082864));
#162637=CARTESIAN_POINT('Ctrl Pts',(79.1408640991085,-1.37888099422469,
40.1284493686468));
#162638=CARTESIAN_POINT('Ctrl Pts',(79.1969131225495,-0.900273005267662,
40.1296765040502));
#162639=CARTESIAN_POINT('Ctrl Pts',(79.2120166812241,-0.732911620517043,
40.1308460556071));
#162640=CARTESIAN_POINT('Ctrl Pts',(79.2301201692722,-0.44767165747966,
40.1340304238583));
#162641=CARTESIAN_POINT('Ctrl Pts',(79.2353864904712,-0.329973162623383,
40.1356878913297));
#162642=CARTESIAN_POINT('Ctrl Pts',(79.2399953393638,-0.152896613307061,
40.1386753662714));
#162643=CARTESIAN_POINT('Ctrl Pts',(79.2409805733825,-0.0935687617643085,
40.1397595508864));
#162644=CARTESIAN_POINT('Ctrl Pts',(79.2417756441276,0.0171343571310466,
40.141934201697));
#162645=CARTESIAN_POINT('Ctrl Pts',(79.2417253579129,0.0685061561100905,
40.1430038747896));
#162646=CARTESIAN_POINT('Ctrl Pts',(79.2405393723288,0.198316966753727,
40.145862727036));
#162647=CARTESIAN_POINT('Ctrl Pts',(79.2388456017844,0.276745149006882,
40.1477341199066));
#162648=CARTESIAN_POINT('Ctrl Pts',(79.2266958131471,0.633535895710569,
40.1569280019748));
#162649=CARTESIAN_POINT('Ctrl Pts',(79.2049162706054,0.911324727069258,
40.1659752389582));
#162650=CARTESIAN_POINT('Ctrl Pts',(79.1308201840326,1.51398763254161,40.1902043929339));
#162651=CARTESIAN_POINT('Ctrl Pts',(79.0737472684379,1.83786918713272,40.2061862422928));
#162652=CARTESIAN_POINT('Ctrl Pts',(78.9468693572766,2.38863464562249,40.238969619491));
#162653=CARTESIAN_POINT('Ctrl Pts',(78.8851227375613,2.61713516379628,40.2542807779887));
#162654=CARTESIAN_POINT('Ctrl Pts',(78.7611506449948,3.01591201382421,40.2841708442066));
#162655=CARTESIAN_POINT('Ctrl Pts',(78.7024520071846,3.18720337326598,40.2980741250929));
#162656=CARTESIAN_POINT('Ctrl Pts',(78.6019158418613,3.45521180937599,40.3215562307497));
#162657=CARTESIAN_POINT('Ctrl Pts',(78.5632988779197,3.55314171169037,40.3305103558352));
#162658=CARTESIAN_POINT('Ctrl Pts',(78.4858067582838,3.74040964736682,40.3483612592754));
#162659=CARTESIAN_POINT('Ctrl Pts',(78.447167727716,3.82983483705147,40.3572119692471));
#162660=CARTESIAN_POINT('Ctrl Pts',(78.3514644851321,4.04221834449071,40.3790196025696));
#162661=CARTESIAN_POINT('Ctrl Pts',(78.2931271441464,4.1645528950215,40.392223508447));
#162662=CARTESIAN_POINT('Ctrl Pts',(78.0078168789051,4.73099632096374,40.4563924015339));
#162663=CARTESIAN_POINT('Ctrl Pts',(77.7486463102321,5.15725351885749,40.5136026126321));
#162664=CARTESIAN_POINT('Ctrl Pts',(77.3206863283474,5.74872508394364,40.6059544544084));
#162665=CARTESIAN_POINT('Ctrl Pts',(77.1773309737015,5.93194861083004,40.6365997975087));
#162666=CARTESIAN_POINT('Ctrl Pts',(76.9336201816306,6.22036087167446,40.6880928754681));
#162667=CARTESIAN_POINT('Ctrl Pts',(76.8373544512968,6.3289871416315,40.7082931366534));
#162668=CARTESIAN_POINT('Ctrl Pts',(76.6936529888984,6.48362957351238,40.7382087838804));
#162669=CARTESIAN_POINT('Ctrl Pts',(76.6481937521214,6.53150765128335,40.7476393126656));
#162670=CARTESIAN_POINT('Ctrl Pts',(76.5635979181965,6.61870699883652,40.765123199216));
#162671=CARTESIAN_POINT('Ctrl Pts',(76.5246114549889,6.6581727814448,40.7731553197284));
#162672=CARTESIAN_POINT('Ctrl Pts',(76.42554841298,6.75665627434309,40.7935045246291));
#162673=CARTESIAN_POINT('Ctrl Pts',(76.365020286901,6.81519945853294,40.8058839748086));
#162674=CARTESIAN_POINT('Ctrl Pts',(75.9682628387157,7.18853890110204,40.8867298339253));
#162675=CARTESIAN_POINT('Ctrl Pts',(75.6099413168321,7.47819094610091,40.9583989267173));
#162676=CARTESIAN_POINT('Ctrl Pts',(75.0164451385431,7.88830547926034,41.0766097788688));
#162677=CARTESIAN_POINT('Ctrl Pts',(74.7948623202521,8.02776587685847,41.1206407226464));
#162678=CARTESIAN_POINT('Ctrl Pts',(74.4035970694484,8.25116612362197,41.1984160313323));
#162679=CARTESIAN_POINT('Ctrl Pts',(74.2366406441687,8.33972885840696,41.2316103939958));
#162680=CARTESIAN_POINT('Ctrl Pts',(73.9724853929517,8.46949016407435,41.2841834598402));
#162681=CARTESIAN_POINT('Ctrl Pts',(73.8770588907614,8.51432465271073,41.3031858730203));
#162682=CARTESIAN_POINT('Ctrl Pts',(73.6935421918448,8.59668187653807,41.3397547972023));
#162683=CARTESIAN_POINT('Ctrl Pts',(73.6055911216708,8.6344931792924,41.3572912992539));
#162684=CARTESIAN_POINT('Ctrl Pts',(73.3968487110747,8.72034908048617,41.3989400714942));
#162685=CARTESIAN_POINT('Ctrl Pts',(73.275607447426,8.76719525347616,41.4231521258974));
#162686=CARTESIAN_POINT('Ctrl Pts',(72.574617214981,9.0208638598537,41.5632644553005));
#162687=CARTESIAN_POINT('Ctrl Pts',(71.9767364706905,9.17050628970856,41.6833724546721));
#162688=CARTESIAN_POINT('Ctrl Pts',(71.0605389639956,9.302462670435,41.8668469884975));
#162689=CARTESIAN_POINT('Ctrl Pts',(70.7503863685099,9.33082130257006,41.9288338080033));
#162690=CARTESIAN_POINT('Ctrl Pts',(70.3616206038549,9.34610747581579,42.0060488675217));
#162691=CARTESIAN_POINT('Ctrl Pts',(70.2838490857534,9.3481559056644,42.0214710740909));
#162692=CARTESIAN_POINT('Ctrl Pts',(70.1550292026933,9.3498779470537,42.0469678176833));
#162693=CARTESIAN_POINT('Ctrl Pts',(70.103995200586,9.35012613747574,42.0570560550074));
#162694=CARTESIAN_POINT('Ctrl Pts',(69.9948658587416,9.34972886556506,42.0785990170841));
#162695=CARTESIAN_POINT('Ctrl Pts',(69.9367731595113,9.34895511508475,42.0900496851414));
#162696=CARTESIAN_POINT('Ctrl Pts',(69.7638200971652,9.34497721317344,42.1240962240466));
#162697=CARTESIAN_POINT('Ctrl Pts',(69.6489993353937,9.34013691494601,42.1466410601758));
#162698=CARTESIAN_POINT('Ctrl Pts',(69.0774723064133,9.30507980673145,42.2586587084679));
#162699=CARTESIAN_POINT('Ctrl Pts',(68.6232402608495,9.24228285780664,42.3470761869048));
#162700=CARTESIAN_POINT('Ctrl Pts',(67.9097657366036,9.08761369718184,42.4864526113399));
#162701=CARTESIAN_POINT('Ctrl Pts',(67.6466408188795,9.01799933247026,42.5379587645335));
#162702=CARTESIAN_POINT('Ctrl Pts',(67.1986103290881,8.87754214742544,42.6260568050637));
#162703=CARTESIAN_POINT('Ctrl Pts',(67.0121825414998,8.81232188638436,42.662836411051));
#162704=CARTESIAN_POINT('Ctrl Pts',(66.728038619582,8.70235398408323,42.7191261300139));
#162705=CARTESIAN_POINT('Ctrl Pts',(66.6287691797809,8.66189476760856,42.7388362275856));
#162706=CARTESIAN_POINT('Ctrl Pts',(66.4426518696476,8.58215867571236,42.7758791117684));
#162707=CARTESIAN_POINT('Ctrl Pts',(66.3556629009143,8.54325654964305,42.7932299775245));
#162708=CARTESIAN_POINT('Ctrl Pts',(66.1567159347037,8.45049602794896,42.8330003126373));
#162709=CARTESIAN_POINT('Ctrl Pts',(66.0452084712299,8.39568989749394,42.8553567766661));
#162710=CARTESIAN_POINT('Ctrl Pts',(65.6229818730283,8.17729419685852,42.9402596343588));
#162711=CARTESIAN_POINT('Ctrl Pts',(65.3205300337658,7.99793250742827,43.0016157665991));
#162712=CARTESIAN_POINT('Ctrl Pts',(64.7884762975327,7.6393216831459,43.1103061647294));
#162713=CARTESIAN_POINT('Ctrl Pts',(64.555693728138,7.46576680244353,43.158148893338));
#162714=CARTESIAN_POINT('Ctrl Pts',(64.2114205164163,7.18271738907033,43.2291182656743));
#162715=CARTESIAN_POINT('Ctrl Pts',(64.0939653786711,7.08105623785201,43.2533706087492));
#162716=CARTESIAN_POINT('Ctrl Pts',(63.8963763295433,6.9011005782983,43.294184314751));
#162717=CARTESIAN_POINT('Ctrl Pts',(63.8150213561381,6.82425344368051,43.310993443668));
#162718=CARTESIAN_POINT('Ctrl Pts',(63.6919449074068,6.70369342141377,43.3364095731042));
#162719=CARTESIAN_POINT('Ctrl Pts',(63.6492442092956,6.66103935392175,43.3452249930653));
#162720=CARTESIAN_POINT('Ctrl Pts',(63.57114551021,6.58148589477237,43.3613393772631));
#162721=CARTESIAN_POINT('Ctrl Pts',(63.5356326743738,6.54470786424593,43.3686632462788));
#162722=CARTESIAN_POINT('Ctrl Pts',(63.4369578602142,6.44081106525514,43.3890072143525));
#162723=CARTESIAN_POINT('Ctrl Pts',(63.3744753284755,6.37302697174889,43.4018825145351));
#162724=CARTESIAN_POINT('Ctrl Pts',(62.9245911232204,5.87013140533381,43.4946014586895));
#162725=CARTESIAN_POINT('Ctrl Pts',(62.5771960843905,5.39953375183719,43.5663550871684));
#162726=CARTESIAN_POINT('Ctrl Pts',(62.1328993282683,4.66149157098412,43.6609930536785));
#162727=CARTESIAN_POINT('Ctrl Pts',(62.0006027829755,4.41783077096674,43.689663020243));
#162728=CARTESIAN_POINT('Ctrl Pts',(61.8273239479175,4.06180653540181,43.7281170695393));
#162729=CARTESIAN_POINT('Ctrl Pts',(61.7774167554764,3.95410969139709,43.7393179233123));
#162730=CARTESIAN_POINT('Ctrl Pts',(61.6909444996785,3.75781204027258,43.7589693305781));
#162731=CARTESIAN_POINT('Ctrl Pts',(61.6536697688438,3.66955354728717,43.767531938949));
#162732=CARTESIAN_POINT('Ctrl Pts',(61.5747152591317,3.47431233467679,43.7858808266835));
#162733=CARTESIAN_POINT('Ctrl Pts',(61.5336302005733,3.3670972434828,43.795572422956));
#162734=CARTESIAN_POINT('Ctrl Pts',(61.4129137765412,3.03391629715225,43.8245141112171));
#162735=CARTESIAN_POINT('Ctrl Pts',(61.3399215869271,2.80555942747109,43.8427060213208));
#162736=CARTESIAN_POINT('Ctrl Pts',(61.1478459981525,2.11476964681497,43.8928282132079));
#162737=CARTESIAN_POINT('Ctrl Pts',(61.0550132523352,1.64554609932949,43.9204740621124));
#162738=CARTESIAN_POINT('Ctrl Pts',(60.9650196414983,0.897656868935989,
43.9537948646728));
#162739=CARTESIAN_POINT('Ctrl Pts',(60.9440265815614,0.622880758051866,
43.9637898398989));
#162740=CARTESIAN_POINT('Ctrl Pts',(60.9324293229476,0.2703185580429,43.9735323750012));
#162741=CARTESIAN_POINT('Ctrl Pts',(60.930828393121,0.193089743113393,43.9754774660033));
#162742=CARTESIAN_POINT('Ctrl Pts',(60.9298340898521,0.0772323930014838,
43.9781056196507));
#162743=CARTESIAN_POINT('Ctrl Pts',(60.9297371095531,0.0386165506464322,
43.9789333153312));
#162744=CARTESIAN_POINT('Ctrl Pts',(60.929874446542,8.11258948064874E-10,
43.9797121921192));
#162745=CARTESIAN_POINT('Origin',(69.6316151486327,0.,39.48523201752));
#162746=CARTESIAN_POINT('',(61.1382522597423,4.12137457381009E-10,45.1614814957336));
#162747=CARTESIAN_POINT('Ctrl Pts',(60.929874446542,8.11258948064874E-10,
43.9797121921192));
#162748=CARTESIAN_POINT('Ctrl Pts',(60.9299209905546,-0.0130872904938113,
43.9799761563382));
#162749=CARTESIAN_POINT('Ctrl Pts',(60.9299944473541,-0.0261746630590688,
43.9802345133084));
#162750=CARTESIAN_POINT('Ctrl Pts',(60.9305559774722,-0.0993897649537978,
43.9816486104862));
#162751=CARTESIAN_POINT('Ctrl Pts',(60.9315852892579,-0.159513992332572,
43.982692009763));
#162752=CARTESIAN_POINT('Ctrl Pts',(60.9364306606604,-0.341809524564983,
43.9855054951462));
#162753=CARTESIAN_POINT('Ctrl Pts',(60.9420263308532,-0.463925828462389,
43.9869132467927));
#162754=CARTESIAN_POINT('Ctrl Pts',(60.9799098776731,-1.04561529117158,
43.9914366266648));
#162755=CARTESIAN_POINT('Ctrl Pts',(61.0431576532714,-1.50257128455147,
43.9885089622415));
#162756=CARTESIAN_POINT('Ctrl Pts',(61.196879571955,-2.22243779266736,43.9748496701503));
#162757=CARTESIAN_POINT('Ctrl Pts',(61.2661133174162,-2.48915851556593,
43.9677287404019));
#162758=CARTESIAN_POINT('Ctrl Pts',(61.4055601963188,-2.9437454262255,43.9522029832889));
#162759=CARTESIAN_POINT('Ctrl Pts',(61.4702990586768,-3.13312396700213,
43.9446837347049));
#162760=CARTESIAN_POINT('Ctrl Pts',(61.579433859146,-3.42203165118672,43.9316138872546));
#162761=CARTESIAN_POINT('Ctrl Pts',(61.6196278176574,-3.5231133364541,43.9267308865454));
#162762=CARTESIAN_POINT('Ctrl Pts',(61.6988604458934,-3.71275113994098,
43.9169840127456));
#162763=CARTESIAN_POINT('Ctrl Pts',(61.7375328853101,-3.80144771614833,
43.9121779867711));
#162764=CARTESIAN_POINT('Ctrl Pts',(61.8297962834592,-4.00446676402548,
43.9006050073493));
#162765=CARTESIAN_POINT('Ctrl Pts',(61.884329831056,-4.11833143294669,43.8936883991611));
#162766=CARTESIAN_POINT('Ctrl Pts',(62.1054104245539,-4.55707892433642,
43.8653597829873));
#162767=CARTESIAN_POINT('Ctrl Pts',(62.2884387343257,-4.87312033652459,
43.8413251412708));
#162768=CARTESIAN_POINT('Ctrl Pts',(62.6778694553592,-5.46351443548356,
43.7888796392884));
#162769=CARTESIAN_POINT('Ctrl Pts',(62.881887916305,-5.73878786888306,43.7608591053587));
#162770=CARTESIAN_POINT('Ctrl Pts',(63.2153108346265,-6.14073293624203,
43.713894031657));
#162771=CARTESIAN_POINT('Ctrl Pts',(63.3342233444991,-6.27595708622766,
43.6969434999822));
#162772=CARTESIAN_POINT('Ctrl Pts',(63.5053464971005,-6.45960618691284,
43.6722085539644));
#162773=CARTESIAN_POINT('Ctrl Pts',(63.5543718618513,-6.51103393484578,
43.6650850600835));
#162774=CARTESIAN_POINT('Ctrl Pts',(63.6423912783223,-6.60128743304134,
43.6522244252394));
#162775=CARTESIAN_POINT('Ctrl Pts',(63.6811540387599,-6.64033917557308,
43.6465364309264));
#162776=CARTESIAN_POINT('Ctrl Pts',(63.7751379313936,-6.7333678802849,43.6326887798273));
#162777=CARTESIAN_POINT('Ctrl Pts',(63.8306816255785,-6.7870013250239,43.6244596838027));
#162778=CARTESIAN_POINT('Ctrl Pts',(64.0574006426934,-7.00055418815421,
43.5907106399741));
#162779=CARTESIAN_POINT('Ctrl Pts',(64.23381449234,-7.15460938819779,43.5640917397328));
#162780=CARTESIAN_POINT('Ctrl Pts',(64.4387743268022,-7.32037836359001,
43.5329262104701));
#162781=CARTESIAN_POINT('Ctrl Pts',(64.4618758988748,-7.33888065488118,
43.5294101374525));
#162782=CARTESIAN_POINT('Ctrl Pts',(64.8000552846765,-7.60708765833748,
43.4778943578133));
#162783=CARTESIAN_POINT('Ctrl Pts',(65.130663091225,-7.83595319738631,43.4269882590408));
#162784=CARTESIAN_POINT('Ctrl Pts',(65.5735765519539,-8.10161883412052,
43.3587624512361));
#162785=CARTESIAN_POINT('Ctrl Pts',(65.6733443395827,-8.1589490318013,43.3433911670074));
#162786=CARTESIAN_POINT('Ctrl Pts',(65.9212273984341,-8.29527941565562,
43.3052113253201));
#162787=CARTESIAN_POINT('Ctrl Pts',(66.0704591653968,-8.37211542221084,
43.2822364845605));
#162788=CARTESIAN_POINT('Ctrl Pts',(66.3138799281448,-8.48913397973545,
43.2448053664669));
#162789=CARTESIAN_POINT('Ctrl Pts',(66.4068054954676,-8.53191079111141,
43.2305260637269));
#162790=CARTESIAN_POINT('Ctrl Pts',(66.5890746599304,-8.61215429028374,
43.2025417815083));
#162791=CARTESIAN_POINT('Ctrl Pts',(66.6783365977451,-8.6497771458296,43.1888480763197));
#162792=CARTESIAN_POINT('Ctrl Pts',(66.8989574384825,-8.73868145263042,
43.1550316990218));
#162793=CARTESIAN_POINT('Ctrl Pts',(67.0309241653182,-8.78835710903653,
43.1348292584908));
#162794=CARTESIAN_POINT('Ctrl Pts',(67.6754425725245,-9.01415018605229,
43.0362797978487));
#162795=CARTESIAN_POINT('Ctrl Pts',(68.2015559974568,-9.14755460333897,
42.9562636022572));
#162796=CARTESIAN_POINT('Ctrl Pts',(69.0683843604958,-9.28715555386641,
42.824099270753));
#162797=CARTESIAN_POINT('Ctrl Pts',(69.4032683390661,-9.32228499097896,
42.7729429953026));
#162798=CARTESIAN_POINT('Ctrl Pts',(69.8339477564941,-9.34355427816323,
42.7066326470644));
#162799=CARTESIAN_POINT('Ctrl Pts',(69.9287245686482,-9.34675724005849,
42.6920073526985));
#162800=CARTESIAN_POINT('Ctrl Pts',(70.0780057445542,-9.34947685933313,
42.6689065932717));
#162801=CARTESIAN_POINT('Ctrl Pts',(70.1324901543966,-9.34998193955134,
42.6604617326749));
#162802=CARTESIAN_POINT('Ctrl Pts',(70.2408015793297,-9.35001689752974,
42.6436436275921));
#162803=CARTESIAN_POINT('Ctrl Pts',(70.2946264739995,-9.34955842850146,
42.6352710140456));
#162804=CARTESIAN_POINT('Ctrl Pts',(70.4399786476469,-9.3470350419613,42.6126257770812));
#162805=CARTESIAN_POINT('Ctrl Pts',(70.5314808258624,-9.34406951025991,
42.5983323429549));
#162806=CARTESIAN_POINT('Ctrl Pts',(71.1304282734307,-9.31563482140017,
42.5045823007641));
#162807=CARTESIAN_POINT('Ctrl Pts',(71.6349727166656,-9.24921818447463,
42.4247596900784));
#162808=CARTESIAN_POINT('Ctrl Pts',(72.4435959916688,-9.0732689185424,42.297474096908));
#162809=CARTESIAN_POINT('Ctrl Pts',(72.7518943480205,-8.98907594780427,
42.2490940805023));
#162810=CARTESIAN_POINT('Ctrl Pts',(73.2154763833307,-8.83603995490335,
42.1768605165121));
#162811=CARTESIAN_POINT('Ctrl Pts',(73.3741840651771,-8.77875008434609,
42.1522248331894));
#162812=CARTESIAN_POINT('Ctrl Pts',(73.6267919481791,-8.67961847217282,
42.1131889577929));
#162813=CARTESIAN_POINT('Ctrl Pts',(73.7216948123277,-8.64052966017992,
42.0985641035961));
#162814=CARTESIAN_POINT('Ctrl Pts',(73.9046859122112,-8.56155209937364,
42.0704472852389));
#162815=CARTESIAN_POINT('Ctrl Pts',(73.9928371042674,-8.52184828206404,
42.0569407723782));
#162816=CARTESIAN_POINT('Ctrl Pts',(74.2071893565151,-8.42121418381412,
42.0241925826026));
#162817=CARTESIAN_POINT('Ctrl Pts',(74.3326759785512,-8.35877049744099,
42.00510312317));
#162818=CARTESIAN_POINT('Ctrl Pts',(74.7859639522824,-8.12017141745381,
41.9364421263923));
#162819=CARTESIAN_POINT('Ctrl Pts',(75.1046785679339,-7.92698624263095,
41.8887545848755));
#162820=CARTESIAN_POINT('Ctrl Pts',(75.6663076405106,-7.53839863897533,
41.8054984011143));
#162821=CARTESIAN_POINT('Ctrl Pts',(75.9126352417361,-7.34900968334908,
41.7692840913695));
#162822=CARTESIAN_POINT('Ctrl Pts',(76.2795040988533,-7.03643446154255,
41.7155123374961));
#162823=CARTESIAN_POINT('Ctrl Pts',(76.4068203834193,-6.92173455258275,
41.6968836145567));
#162824=CARTESIAN_POINT('Ctrl Pts',(76.5815792670809,-6.75530631922667,
41.6712967221839));
#162825=CARTESIAN_POINT('Ctrl Pts',(76.6316925978708,-6.70649115315063,
41.6639574359783));
#162826=CARTESIAN_POINT('Ctrl Pts',(76.7202981554453,-6.61820890004091,
41.650971208612));
#162827=CARTESIAN_POINT('Ctrl Pts',(76.7589965028812,-6.57895958902068,
41.6452955940362));
#162828=CARTESIAN_POINT('Ctrl Pts',(76.852064834678,-6.48287184147069,41.6316381285602));
#162829=CARTESIAN_POINT('Ctrl Pts',(76.9060701671541,-6.42568035877447,
41.6237071242845));
#162830=CARTESIAN_POINT('Ctrl Pts',(77.1285637878929,-6.18399693051358,
41.5910305509958));
#162831=CARTESIAN_POINT('Ctrl Pts',(77.290382709765,-5.99337779251858,41.567261853574));
#162832=CARTESIAN_POINT('Ctrl Pts',(77.6978206354888,-5.47245776213364,
41.5078315652562));
#162833=CARTESIAN_POINT('Ctrl Pts',(77.9297592054409,-5.13190989184838,
41.4744621993957));
#162834=CARTESIAN_POINT('Ctrl Pts',(78.1981728666291,-4.67625446679963,
41.4371742514691));
#162835=CARTESIAN_POINT('Ctrl Pts',(78.2556511865557,-4.57439393170683,
41.4292803215586));
#162836=CARTESIAN_POINT('Ctrl Pts',(78.3920767067075,-4.32177106537669,
41.410794422422));
#162837=CARTESIAN_POINT('Ctrl Pts',(78.4688829512352,-4.16987133210278,
41.4006106551626));
#162838=CARTESIAN_POINT('Ctrl Pts',(78.5856855705646,-3.92251602092376,
41.3855305229244));
#162839=CARTESIAN_POINT('Ctrl Pts',(78.6282759314851,-3.82835982540036,
41.3801301387383));
#162840=CARTESIAN_POINT('Ctrl Pts',(78.7080868822639,-3.64394167841615,
41.3702129906535));
#162841=CARTESIAN_POINT('Ctrl Pts',(78.7454694341236,-3.55376602715356,
41.365664387133));
#162842=CARTESIAN_POINT('Ctrl Pts',(78.8336590320809,-3.33138650378868,
41.3551813586886));
#162843=CARTESIAN_POINT('Ctrl Pts',(78.8829151606207,-3.19857984561665,
41.349547363618));
#162844=CARTESIAN_POINT('Ctrl Pts',(79.1104129561395,-2.5403701156978,41.3246749076488));
#162845=CARTESIAN_POINT('Ctrl Pts',(79.2454394496049,-2.00089460340364,
41.3138032124655));
#162846=CARTESIAN_POINT('Ctrl Pts',(79.3851840669939,-1.12154875001106,
41.3098978866272));
#162847=CARTESIAN_POINT('Ctrl Pts',(79.4202271830719,-0.787861633838131,
41.3114882719926));
#162848=CARTESIAN_POINT('Ctrl Pts',(79.4423995195219,-0.357782861416539,
41.317082592239));
#162849=CARTESIAN_POINT('Ctrl Pts',(79.4458699131387,-0.262444002311809,
41.3185448251693));
#162850=CARTESIAN_POINT('Ctrl Pts',(79.4490650384667,-0.1120659896724,41.3211886110961));
#162851=CARTESIAN_POINT('Ctrl Pts',(79.4497533589494,-0.0570512986255439,
41.3222269714023));
#162852=CARTESIAN_POINT('Ctrl Pts',(79.450141429027,0.0458317549567954,
41.3242988653224));
#162853=CARTESIAN_POINT('Ctrl Pts',(79.4499580066213,0.0936982065092859,
41.3253154275176));
#162854=CARTESIAN_POINT('Ctrl Pts',(79.4484330367104,0.227089348265823,
41.328298384151));
#162855=CARTESIAN_POINT('Ctrl Pts',(79.4462937167672,0.312597542125527,
41.3303825413586));
#162856=CARTESIAN_POINT('Ctrl Pts',(79.4239798614364,0.890640058614525,
41.3456815856209));
#162857=CARTESIAN_POINT('Ctrl Pts',(79.3664794302618,1.38079853340422,41.364634055881));
#162858=CARTESIAN_POINT('Ctrl Pts',(79.1930592154606,2.26037060267193,41.4115758706752));
#162859=CARTESIAN_POINT('Ctrl Pts',(79.0896634774893,2.65113601644154,41.4372784661021));
#162860=CARTESIAN_POINT('Ctrl Pts',(78.9153565721231,3.17255386773523,41.478753547543));
#162861=CARTESIAN_POINT('Ctrl Pts',(78.8657654608926,3.31018336640328,41.4904061176143));
#162862=CARTESIAN_POINT('Ctrl Pts',(78.7772447977201,3.53903831672365,41.5109889941186));
#162863=CARTESIAN_POINT('Ctrl Pts',(78.7400269260037,3.63092667698288,41.5195868869408));
#162864=CARTESIAN_POINT('Ctrl Pts',(78.6615879272084,3.8161385768787,41.537600870881));
#162865=CARTESIAN_POINT('Ctrl Pts',(78.6202865170046,3.90941201579866,41.547032380804));
#162866=CARTESIAN_POINT('Ctrl Pts',(78.5087579794538,4.15061849960385,41.5723669270285));
#162867=CARTESIAN_POINT('Ctrl Pts',(78.4361883237057,4.2973810929582,41.5887241858183));
#162868=CARTESIAN_POINT('Ctrl Pts',(78.2627862883836,4.62614525731714,41.6275227786336));
#162869=CARTESIAN_POINT('Ctrl Pts',(78.1596804943812,4.80679676208777,41.650399441286));
#162870=CARTESIAN_POINT('Ctrl Pts',(77.8775850972401,5.26488466117879,41.7124436014301));
#162871=CARTESIAN_POINT('Ctrl Pts',(77.6898535057495,5.53637245625685,41.7532352551908));
#162872=CARTESIAN_POINT('Ctrl Pts',(77.3361300789358,5.99382616202806,41.8289122953539));
#162873=CARTESIAN_POINT('Ctrl Pts',(77.1762363538057,6.18425650362277,41.8627602558458));
#162874=CARTESIAN_POINT('Ctrl Pts',(76.9562526692443,6.42575330159449,41.9087048707286));
#162875=CARTESIAN_POINT('Ctrl Pts',(76.902820575212,6.48293136439645,41.9198191761165));
#162876=CARTESIAN_POINT('Ctrl Pts',(76.8107200257987,6.57900494192104,41.9388929892983));
#162877=CARTESIAN_POINT('Ctrl Pts',(76.7724158704434,6.6182532544279,41.9468014458163));
#162878=CARTESIAN_POINT('Ctrl Pts',(76.6846955543587,6.70654271995284,41.9648570640654));
#162879=CARTESIAN_POINT('Ctrl Pts',(76.6350725544141,6.75536638226418,41.9750328111978));
#162880=CARTESIAN_POINT('Ctrl Pts',(76.4619578983732,6.92186803363263,42.010414973467));
#162881=CARTESIAN_POINT('Ctrl Pts',(76.3357899255324,7.03663091278496,42.0360009439495));
#162882=CARTESIAN_POINT('Ctrl Pts',(75.9720186263783,7.3494768557231,42.1093733591845));
#162883=CARTESIAN_POINT('Ctrl Pts',(75.7276207193639,7.53905058114165,42.1582185491852));
#162884=CARTESIAN_POINT('Ctrl Pts',(75.1709220369443,7.92747425024709,42.2691305383306));
#162885=CARTESIAN_POINT('Ctrl Pts',(74.8552643274913,8.1203812123864,42.3318060257228));
#162886=CARTESIAN_POINT('Ctrl Pts',(74.406064528023,8.3587553228919,42.4211344157782));
#162887=CARTESIAN_POINT('Ctrl Pts',(74.281573591726,8.4212021924072,42.4459026005887));
#162888=CARTESIAN_POINT('Ctrl Pts',(74.0689080409677,8.52183951921638,42.4882484645318));
#162889=CARTESIAN_POINT('Ctrl Pts',(73.9814469472917,8.56154390675176,42.5056733013665));
#162890=CARTESIAN_POINT('Ctrl Pts',(73.799881376015,8.64052158854995,42.5418698858085));
#162891=CARTESIAN_POINT('Ctrl Pts',(73.7057139769804,8.67960992021873,42.5606556280213));
#162892=CARTESIAN_POINT('Ctrl Pts',(73.4550564346684,8.7787385320311,42.6106958356382));
#162893=CARTESIAN_POINT('Ctrl Pts',(73.2975650648375,8.83602556366342,42.6421735631669));
#162894=CARTESIAN_POINT('Ctrl Pts',(72.8373046401687,8.98912228284667,42.7342617389544));
#162895=CARTESIAN_POINT('Ctrl Pts',(72.531108249263,9.07335714483024,42.7956500358838));
#162896=CARTESIAN_POINT('Ctrl Pts',(71.7284958395458,9.24924260375135,42.9565965913385));
#162897=CARTESIAN_POINT('Ctrl Pts',(71.2278526250868,9.31562014137933,43.057049277711));
#162898=CARTESIAN_POINT('Ctrl Pts',(70.6334199380153,9.34406208962301,43.175232095481));
#162899=CARTESIAN_POINT('Ctrl Pts',(70.5425303840906,9.34703103503685,43.1932710781474));
#162900=CARTESIAN_POINT('Ctrl Pts',(70.3981681784863,9.34955725161712,43.2218611099207));
#162901=CARTESIAN_POINT('Ctrl Pts',(70.3447213966133,9.35001641062416,43.2324324736563));
#162902=CARTESIAN_POINT('Ctrl Pts',(70.2371902283325,9.34998249508892,43.2536710627285));
#162903=CARTESIAN_POINT('Ctrl Pts',(70.1831079350329,9.34947813337265,43.2643375789638));
#162904=CARTESIAN_POINT('Ctrl Pts',(70.0349618363308,9.34676155982657,43.2935193913017));
#162905=CARTESIAN_POINT('Ctrl Pts',(69.9409170113203,9.34356234659907,43.3120038491778));
#162906=CARTESIAN_POINT('Ctrl Pts',(69.513865314358,9.32233191380107,43.3958017314541));
#162907=CARTESIAN_POINT('Ctrl Pts',(69.1818631633314,9.28728878461765,43.4605716254989));
#162908=CARTESIAN_POINT('Ctrl Pts',(68.3210744725876,9.14780960690269,43.6285286192555));
#162909=CARTESIAN_POINT('Ctrl Pts',(67.7981528737183,9.01426858421186,43.7306386355001));
#162910=CARTESIAN_POINT('Ctrl Pts',(67.1579455841596,8.78824228614249,43.8570077433325));
#162911=CARTESIAN_POINT('Ctrl Pts',(67.0270426558559,8.73858274292404,43.8829164751728));
#162912=CARTESIAN_POINT('Ctrl Pts',(66.8081873070179,8.64969885775567,43.9263647410801));
#162913=CARTESIAN_POINT('Ctrl Pts',(66.7196268544439,8.61207756716473,43.9439833051687));
#162914=CARTESIAN_POINT('Ctrl Pts',(66.5387764045311,8.5318275673468,43.9800416334691));
#162915=CARTESIAN_POINT('Ctrl Pts',(66.446568414161,8.48904191379462,43.9984695325005));
#162916=CARTESIAN_POINT('Ctrl Pts',(66.2049827429779,8.37196967333293,44.0468664988398));
#162917=CARTESIAN_POINT('Ctrl Pts',(66.0568718116279,8.29508531521283,44.0766569857511));
#162918=CARTESIAN_POINT('Ctrl Pts',(65.8108567620796,8.15865188963051,44.1263330451793));
#162919=CARTESIAN_POINT('Ctrl Pts',(65.7118336099486,8.10126735062367,44.1463826385841));
#162920=CARTESIAN_POINT('Ctrl Pts',(65.271988490689,7.8351731583931,44.2356677593333));
#162921=CARTESIAN_POINT('Ctrl Pts',(64.9437478937064,7.60586242795574,44.302943578339));
#162922=CARTESIAN_POINT('Ctrl Pts',(64.5178369365655,7.26475498713987,44.3906652689716));
#162923=CARTESIAN_POINT('Ctrl Pts',(64.4066026863542,7.17125310750033,44.4136162063759));
#162924=CARTESIAN_POINT('Ctrl Pts',(64.1897106581652,6.97999193005325,44.4584006015486));
#162925=CARTESIAN_POINT('Ctrl Pts',(64.084035169991,6.88231391618696,44.4802373122885));
#162926=CARTESIAN_POINT('Ctrl Pts',(63.9333581290706,6.73636664256785,44.5113576717171));
#162927=CARTESIAN_POINT('Ctrl Pts',(63.8865623425043,6.6900614563923,44.5210204194965));
#162928=CARTESIAN_POINT('Ctrl Pts',(63.8012128372173,6.60378598122045,44.5386345307307));
#162929=CARTESIAN_POINT('Ctrl Pts',(63.7625204231549,6.56396436231669,44.5466154792701));
#162930=CARTESIAN_POINT('Ctrl Pts',(63.66579922435,6.46261405457758,44.5665584431515));
#162931=CARTESIAN_POINT('Ctrl Pts',(63.6082402284705,6.40062458248858,44.5784201737169));
#162932=CARTESIAN_POINT('Ctrl Pts',(63.4813400024463,6.26015084017721,44.6045728241438));
#162933=CARTESIAN_POINT('Ctrl Pts',(63.4124540040022,6.18125385581165,44.6187702209928));
#162934=CARTESIAN_POINT('Ctrl Pts',(63.1905921492661,5.91829912460944,44.6645398524805));
#162935=CARTESIAN_POINT('Ctrl Pts',(63.0432962000735,5.72938605340831,44.6949995989251));
#162936=CARTESIAN_POINT('Ctrl Pts',(62.6198724885067,5.14079846788911,44.783193732117));
#162937=CARTESIAN_POINT('Ctrl Pts',(62.3672559275494,4.72463370734902,44.8367509308623));
#162938=CARTESIAN_POINT('Ctrl Pts',(62.0865672635927,4.16858268396669,44.8985438975456));
#162939=CARTESIAN_POINT('Ctrl Pts',(62.02781886073,4.04559660439793,44.9116349969973));
#162940=CARTESIAN_POINT('Ctrl Pts',(61.9316656869516,3.83246425641149,44.9333575527785));
#162941=CARTESIAN_POINT('Ctrl Pts',(61.8929534106559,3.74295411952806,44.9421958463912));
#162942=CARTESIAN_POINT('Ctrl Pts',(61.8154785592952,3.55585869649356,44.9600865498486));
#162943=CARTESIAN_POINT('Ctrl Pts',(61.7769423149437,3.458191129328,44.9691027208434));
#162944=CARTESIAN_POINT('Ctrl Pts',(61.676997221994,3.19188556461019,44.992819886734));
#162945=CARTESIAN_POINT('Ctrl Pts',(61.6187555577885,3.02206269472006,45.0070167169159));
#162946=CARTESIAN_POINT('Ctrl Pts',(61.3369077133837,2.11657346626009,45.0778441435093));
#162947=CARTESIAN_POINT('Ctrl Pts',(61.1989673516544,1.35632821540749,45.1208272762866));
#162948=CARTESIAN_POINT('Ctrl Pts',(61.1471447103106,0.464914684249992,
45.1499345847225));
#162949=CARTESIAN_POINT('Ctrl Pts',(61.1423965910819,0.342526707933256,
45.1534657989348));
#162950=CARTESIAN_POINT('Ctrl Pts',(61.1388333915165,0.159909273635988,
45.1580172834175));
#162951=CARTESIAN_POINT('Ctrl Pts',(61.1382289181497,0.099736719295513,
45.1594009230751));
#162952=CARTESIAN_POINT('Ctrl Pts',(61.13818578755,0.0263733213606727,45.1609438644884));
#162953=CARTESIAN_POINT('Ctrl Pts',(61.1382053624156,0.0131866373259202,
45.1612155277709));
#162954=CARTESIAN_POINT('Ctrl Pts',(61.1382522597423,8.24276059806775E-10,
45.1614814957336));
#162955=CARTESIAN_POINT('',(61.1677177485993,-7.6877934180699E-10,45.3285885869945));
#162956=CARTESIAN_POINT('',(60.4236626579685,-1.14504475720278E-15,41.1088424787055));
#162957=CARTESIAN_POINT('Ctrl Pts',(61.1677177485993,-1.53755753856922E-9,
45.3285885869945));
#162958=CARTESIAN_POINT('Ctrl Pts',(61.1676477590131,0.0196797378694619,
45.3281916563455));
#162959=CARTESIAN_POINT('Ctrl Pts',(61.167639291223,0.0393596012676555,
45.3277858276557));
#162960=CARTESIAN_POINT('Ctrl Pts',(61.167863801354,0.122656517391383,45.3260301005657));
#162961=CARTESIAN_POINT('Ctrl Pts',(61.1686780323739,0.186268278702916,
45.3245954280457));
#162962=CARTESIAN_POINT('Ctrl Pts',(61.173410355421,0.392916285528057,45.3196204158403));
#162963=CARTESIAN_POINT('Ctrl Pts',(61.1799347051901,0.535862702174635,
45.3156892391233));
#162964=CARTESIAN_POINT('Ctrl Pts',(61.2050985037226,0.903766273149247,
45.3042277371107));
#162965=CARTESIAN_POINT('Ctrl Pts',(61.2285507049289,1.1282763895979,45.2959329068203));
#162966=CARTESIAN_POINT('Ctrl Pts',(61.3439704193222,1.94846801799224,45.2604403057768));
#162967=CARTESIAN_POINT('Ctrl Pts',(61.4846525612222,2.53542694868968,45.2248135093029));
#162968=CARTESIAN_POINT('Ctrl Pts',(61.7237161276422,3.23224163497682,45.1681809287438));
#162969=CARTESIAN_POINT('Ctrl Pts',(61.7703237391244,3.35914822458267,45.1572613655166));
#162970=CARTESIAN_POINT('Ctrl Pts',(61.8551699609553,3.5756874316554,45.1375692710115));
#162971=CARTESIAN_POINT('Ctrl Pts',(61.8921103361962,3.66582759362413,45.1290489906753));
#162972=CARTESIAN_POINT('Ctrl Pts',(61.9718726162913,3.85217572208756,45.1107562198392));
#162973=CARTESIAN_POINT('Ctrl Pts',(62.0149227113742,3.94826665633113,45.1009395701924));
#162974=CARTESIAN_POINT('Ctrl Pts',(62.1370907716631,4.20913513340219,45.0732303231735));
#162975=CARTESIAN_POINT('Ctrl Pts',(62.2193883904309,4.37230519893804,45.0547214072867));
#162976=CARTESIAN_POINT('Ctrl Pts',(62.423551872379,4.74930801230215,45.0091735457337));
#162977=CARTESIAN_POINT('Ctrl Pts',(62.5491450406586,4.96087934971187,44.9814230874892));
#162978=CARTESIAN_POINT('Ctrl Pts',(62.9454545680935,5.57216908699487,44.8947670463164));
#162979=CARTESIAN_POINT('Ctrl Pts',(63.2387310475505,5.95567651204903,44.8317248904969));
#162980=CARTESIAN_POINT('Ctrl Pts',(63.6201647204983,6.38107464424242,44.7518600097091));
#162981=CARTESIAN_POINT('Ctrl Pts',(63.6811440950029,6.44711479845384,44.7391504286313));
#162982=CARTESIAN_POINT('Ctrl Pts',(63.7814914863825,6.55264943184969,44.7183399509459));
#162983=CARTESIAN_POINT('Ctrl Pts',(63.8202775642236,6.59270555139911,44.7103208491484));
#162984=CARTESIAN_POINT('Ctrl Pts',(63.903858481368,6.67746803081045,44.6930952566027));
#162985=CARTESIAN_POINT('Ctrl Pts',(63.9487536242128,6.72206776685744,44.6838748675467));
#162986=CARTESIAN_POINT('Ctrl Pts',(64.0860348613951,6.85566003434745,44.6557682788216));
#162987=CARTESIAN_POINT('Ctrl Pts',(64.1798054109601,6.94316600886333,44.6366877387674));
#162988=CARTESIAN_POINT('Ctrl Pts',(64.5625954944672,7.28568678347697,44.5591649764643));
#162989=CARTESIAN_POINT('Ctrl Pts',(64.8654605867275,7.52414985056887,44.498629694355));
#162990=CARTESIAN_POINT('Ctrl Pts',(65.5000399179384,7.9620734768268,44.3722405517229));
#162991=CARTESIAN_POINT('Ctrl Pts',(65.8312377835154,8.16092743258981,44.3064878143495));
#162992=CARTESIAN_POINT('Ctrl Pts',(66.2842077868128,8.39521545841935,44.216388367868));
#162993=CARTESIAN_POINT('Ctrl Pts',(66.3958786653038,8.45010302211099,44.1941648789301));
#162994=CARTESIAN_POINT('Ctrl Pts',(66.5950010223712,8.54295361129934,44.154507758706));
#162995=CARTESIAN_POINT('Ctrl Pts',(66.6820057377898,8.58186984597548,44.1371701030178));
#162996=CARTESIAN_POINT('Ctrl Pts',(66.868043911442,8.66159405905865,44.1000737286449));
#162997=CARTESIAN_POINT('Ctrl Pts',(66.967214734366,8.70203041623254,44.0802846228976));
#162998=CARTESIAN_POINT('Ctrl Pts',(67.2507284419084,8.81181845287383,44.0236682754481));
#162999=CARTESIAN_POINT('Ctrl Pts',(67.4365878878049,8.87690857348241,43.9865017852307));
#163000=CARTESIAN_POINT('Ctrl Pts',(67.8827983819796,9.01701280948911,43.8971723781408));
#163001=CARTESIAN_POINT('Ctrl Pts',(68.1446288415709,9.08646694553515,43.8446736501665));
#163002=CARTESIAN_POINT('Ctrl Pts',(68.8518744734904,9.2403893370759,43.7028506978136));
#163003=CARTESIAN_POINT('Ctrl Pts',(69.3010521594204,9.30318695348168,43.6127418206919));
#163004=CARTESIAN_POINT('Ctrl Pts',(69.8717811750552,9.33944131655441,43.4990804655496));
#163005=CARTESIAN_POINT('Ctrl Pts',(69.990654553494,9.34462815263743,43.4754539369393));
#163006=CARTESIAN_POINT('Ctrl Pts',(70.1684171434169,9.34885502096827,43.4402183116053));
#163007=CARTESIAN_POINT('Ctrl Pts',(70.2272440715516,9.34967684163236,43.4285734044959));
#163008=CARTESIAN_POINT('Ctrl Pts',(70.336861325391,9.35013343574715,43.4069074827117));
#163009=CARTESIAN_POINT('Ctrl Pts',(70.3876473481467,9.34991524572804,43.3968832234318));
#163010=CARTESIAN_POINT('Ctrl Pts',(70.5145787140558,9.34829589901693,43.3718603939617));
#163011=CARTESIAN_POINT('Ctrl Pts',(70.5907165381837,9.34635840181797,43.35687855519));
#163012=CARTESIAN_POINT('Ctrl Pts',(70.9430782427855,9.33291794706796,43.2876471116057));
#163013=CARTESIAN_POINT('Ctrl Pts',(71.2187761500021,9.30966600004778,43.2337705059214));
#163014=CARTESIAN_POINT('Ctrl Pts',(71.9615613503377,9.21244669351037,43.0887819980959));
#163015=CARTESIAN_POINT('Ctrl Pts',(72.424764235412,9.11436946647626,42.9985165699943));
#163016=CARTESIAN_POINT('Ctrl Pts',(73.0986166813944,8.91537266134385,42.8662229351626));
#163017=CARTESIAN_POINT('Ctrl Pts',(73.3163506661664,8.84194863882161,42.8233251904865));
#163018=CARTESIAN_POINT('Ctrl Pts',(73.6361121080951,8.72037471691119,42.7600266783593));
#163019=CARTESIAN_POINT('Ctrl Pts',(73.7403678569712,8.678499951483,42.7393404353094));
#163020=CARTESIAN_POINT('Ctrl Pts',(73.9301569633891,8.59813876533699,42.7015883988948));
#163021=CARTESIAN_POINT('Ctrl Pts',(74.0159186706203,8.56024553943473,42.6844929800991));
#163022=CARTESIAN_POINT('Ctrl Pts',(74.2082435135765,8.47167774716821,42.6460721122907));
#163023=CARTESIAN_POINT('Ctrl Pts',(74.3144449665,8.42023672012054,42.6247971368161));
#163024=CARTESIAN_POINT('Ctrl Pts',(74.6696079742394,8.23957366494244,42.5534494681739));
#163025=CARTESIAN_POINT('Ctrl Pts',(74.9136886731471,8.1008393207779,42.5040759136865));
#163026=CARTESIAN_POINT('Ctrl Pts',(75.4306035435402,7.77454279510815,42.3988783192705));
#163027=CARTESIAN_POINT('Ctrl Pts',(75.7005052347357,7.58291884366461,42.3435334817253));
#163028=CARTESIAN_POINT('Ctrl Pts',(76.1678518133562,7.21148272380045,42.247304416424));
#163029=CARTESIAN_POINT('Ctrl Pts',(76.3688854772619,7.03694469905623,42.2057656134607));
#163030=CARTESIAN_POINT('Ctrl Pts',(76.620200299385,6.79891853415568,42.1538510448426));
#163031=CARTESIAN_POINT('Ctrl Pts',(76.6774411557679,6.74328016953733,42.1420279427955));
#163032=CARTESIAN_POINT('Ctrl Pts',(76.7728855253443,6.64807517892203,42.1223243994538));
#163033=CARTESIAN_POINT('Ctrl Pts',(76.8114611868241,6.60890495863334,42.1143641248462));
#163034=CARTESIAN_POINT('Ctrl Pts',(76.8973358540869,6.52014047484161,42.0966523094367));
#163035=CARTESIAN_POINT('Ctrl Pts',(76.9444416088117,6.47035690471482,42.0869419779306));
#163036=CARTESIAN_POINT('Ctrl Pts',(77.1012616674015,6.3008977464525,42.0546207467143));
#163037=CARTESIAN_POINT('Ctrl Pts',(77.2084355543498,6.17881227363132,42.0325407442862));
#163038=CARTESIAN_POINT('Ctrl Pts',(77.493070476014,5.83687859668239,41.9737965593625));
#163039=CARTESIAN_POINT('Ctrl Pts',(77.663907612997,5.61153016549304,41.9384175556734));
#163040=CARTESIAN_POINT('Ctrl Pts',(78.058568218926,5.0384787869797,41.855853885111));
#163041=CARTESIAN_POINT('Ctrl Pts',(78.2701808333373,4.68281150404958,41.8108013660867));
#163042=CARTESIAN_POINT('Ctrl Pts',(78.521208736461,4.18901532643776,41.7556213406319));
#163043=CARTESIAN_POINT('Ctrl Pts',(78.5819209265913,4.06263931737579,41.7421104479428));
#163044=CARTESIAN_POINT('Ctrl Pts',(78.6798621217743,3.84646127984038,41.7200068665661));
#163045=CARTESIAN_POINT('Ctrl Pts',(78.7185648551685,3.75737750943101,41.7111809634627));
#163046=CARTESIAN_POINT('Ctrl Pts',(78.795621425458,3.57219111347478,41.693409710767));
#163047=CARTESIAN_POINT('Ctrl Pts',(78.8337847054525,3.47602074711184,41.6844949207615));
#163048=CARTESIAN_POINT('Ctrl Pts',(78.9307475605304,3.21937993075291,41.6615294758774));
#163049=CARTESIAN_POINT('Ctrl Pts',(78.9867831822521,3.0578687030203,41.6479187067432));
#163050=CARTESIAN_POINT('Ctrl Pts',(79.1313180781754,2.60146159058633,41.6117989491338));
#163051=CARTESIAN_POINT('Ctrl Pts',(79.2098338054738,2.30350981565174,41.590899710545));
#163052=CARTESIAN_POINT('Ctrl Pts',(79.3839277782985,1.48163138476183,41.5406959315158));
#163053=CARTESIAN_POINT('Ctrl Pts',(79.4501062043757,0.952357541808737,
41.5163796898752));
#163054=CARTESIAN_POINT('Ctrl Pts',(79.4752948968429,0.330771953954673,
41.4982523339804));
#163055=CARTESIAN_POINT('Ctrl Pts',(79.4776569956186,0.241428764387,41.4958981718124));
#163056=CARTESIAN_POINT('Ctrl Pts',(79.4794293668053,0.0982487996310115,
41.4925384714185));
#163057=CARTESIAN_POINT('Ctrl Pts',(79.479640148999,0.0444310586602378,
41.4913691028231));
#163058=CARTESIAN_POINT('Ctrl Pts',(79.479142108966,-0.0652733811300169,
41.4891788900632));
#163059=CARTESIAN_POINT('Ctrl Pts',(79.4783976381843,-0.121157702673901,
41.4881653415837));
#163060=CARTESIAN_POINT('Ctrl Pts',(79.4749573213269,-0.276748057348876,
41.4856225142354));
#163061=CARTESIAN_POINT('Ctrl Pts',(79.4711889742514,-0.376426368375324,
41.4843126162585));
#163062=CARTESIAN_POINT('Ctrl Pts',(79.4587711965098,-0.608378627047333,
41.4819828885302));
#163063=CARTESIAN_POINT('Ctrl Pts',(79.4489258043924,-0.740569328250936,
41.4812001631271));
#163064=CARTESIAN_POINT('Ctrl Pts',(79.4003239678058,-1.24939102268216,
41.4801997821917));
#163065=CARTESIAN_POINT('Ctrl Pts',(79.3418693483576,-1.62377876705432,
41.4837172802535));
#163066=CARTESIAN_POINT('Ctrl Pts',(79.1773345948621,-2.3780955630158,41.4986104255801));
#163067=CARTESIAN_POINT('Ctrl Pts',(79.0696242685249,-2.75689576457783,
41.5102727087625));
#163068=CARTESIAN_POINT('Ctrl Pts',(78.8946837323403,-3.25228121011682,
41.5307953126299));
#163069=CARTESIAN_POINT('Ctrl Pts',(78.8481057896132,-3.37585821025091,
41.5363712130807));
#163070=CARTESIAN_POINT('Ctrl Pts',(78.7627668173874,-3.58863083514753,
41.5467610696678));
#163071=CARTESIAN_POINT('Ctrl Pts',(78.7251882646852,-3.67828718114622,
41.551387691164));
#163072=CARTESIAN_POINT('Ctrl Pts',(78.6433493984693,-3.86537301179641,
41.5615656104316));
#163073=CARTESIAN_POINT('Ctrl Pts',(78.5988035946059,-3.96265986515513,
41.5671623259228));
#163074=CARTESIAN_POINT('Ctrl Pts',(78.469881010801,-4.23200731986905,41.5835124971289));
#163075=CARTESIAN_POINT('Ctrl Pts',(78.3819100340444,-4.40225328813357,
41.5948372670927));
#163076=CARTESIAN_POINT('Ctrl Pts',(78.1600381891994,-4.80127674475564,
41.6238024343062));
#163077=CARTESIAN_POINT('Ctrl Pts',(78.0215655062823,-5.02726844703198,
41.6421838866607));
#163078=CARTESIAN_POINT('Ctrl Pts',(77.6147944477545,-5.63219087061544,
41.6971594665461));
#163079=CARTESIAN_POINT('Ctrl Pts',(77.3278003134506,-5.99733621274991,
41.7369505904207));
#163080=CARTESIAN_POINT('Ctrl Pts',(76.9582283939438,-6.40192347428828,
41.7901257607769));
#163081=CARTESIAN_POINT('Ctrl Pts',(76.9002864452452,-6.46365309845526,
41.7985138341587));
#163082=CARTESIAN_POINT('Ctrl Pts',(76.8028168428692,-6.56471313104887,
41.8127174052415));
#163083=CARTESIAN_POINT('Ctrl Pts',(76.7637533245473,-6.60449805577137,
41.8184341197212));
#163084=CARTESIAN_POINT('Ctrl Pts',(76.6774347767246,-6.69085357916132,
41.8311212132567));
#163085=CARTESIAN_POINT('Ctrl Pts',(76.6300379103083,-6.73727242026035,
41.8381220211692));
#163086=CARTESIAN_POINT('Ctrl Pts',(76.4769084909859,-6.88408025898879,
41.8608384702931));
#163087=CARTESIAN_POINT('Ctrl Pts',(76.3693486060981,-6.98247071309434,
41.8769416089686));
#163088=CARTESIAN_POINT('Ctrl Pts',(76.0837139780331,-7.23170111570235,
41.9199911856907));
#163089=CARTESIAN_POINT('Ctrl Pts',(75.9022560713896,-7.37838660281563,
41.9476150334515));
#163090=CARTESIAN_POINT('Ctrl Pts',(75.3175820061411,-7.81562462278688,
42.0370753513736));
#163091=CARTESIAN_POINT('Ctrl Pts',(74.8967233754039,-8.0804368107359,42.1020700007053));
#163092=CARTESIAN_POINT('Ctrl Pts',(74.3372618439705,-8.37230850723725,
42.1881986386075));
#163093=CARTESIAN_POINT('Ctrl Pts',(74.2162826783661,-8.43207525160566,
42.2068116474129));
#163094=CARTESIAN_POINT('Ctrl Pts',(74.0062698268108,-8.53013655614144,
42.2390897516805));
#163095=CARTESIAN_POINT('Ctrl Pts',(73.9178544217449,-8.56972960844439,
42.252669100105));
#163096=CARTESIAN_POINT('Ctrl Pts',(73.7327177194676,-8.64914359718673,
42.2810798338431));
#163097=CARTESIAN_POINT('Ctrl Pts',(73.6359103363512,-8.68872455613769,
42.2959225395044));
#163098=CARTESIAN_POINT('Ctrl Pts',(73.3710246724264,-8.7917789126022,42.3364974534785));
#163099=CARTESIAN_POINT('Ctrl Pts',(73.2017458500141,-8.85197578528895,
42.3623858883258));
#163100=CARTESIAN_POINT('Ctrl Pts',(72.8076965428904,-8.97919331143696,
42.4225656644022));
#163101=CARTESIAN_POINT('Ctrl Pts',(72.5819205404346,-9.04263070916509,
42.4569841644419));
#163102=CARTESIAN_POINT('Ctrl Pts',(72.0374785972847,-9.17329194636696,
42.5399299344996));
#163103=CARTESIAN_POINT('Ctrl Pts',(71.7172007969965,-9.23230866803508,
42.5886787531538));
#163104=CARTESIAN_POINT('Ctrl Pts',(71.1208442236375,-9.30961048539096,
42.6797470511734));
#163105=CARTESIAN_POINT('Ctrl Pts',(70.8457261892187,-9.3326789495219,42.7218775705995));
#163106=CARTESIAN_POINT('Ctrl Pts',(70.4926140787116,-9.34624172756384,
42.7763350439376));
#163107=CARTESIAN_POINT('Ctrl Pts',(70.4151482704105,-9.34823077140995,
42.788305763241));
#163108=CARTESIAN_POINT('Ctrl Pts',(70.2864046800583,-9.34989801630088,
42.8082476338993));
#163109=CARTESIAN_POINT('Ctrl Pts',(70.2351352869908,-9.35013031059697,
42.8162016342404));
#163110=CARTESIAN_POINT('Ctrl Pts',(70.1249660759063,-9.34970187027052,
42.8333225496654));
#163111=CARTESIAN_POINT('Ctrl Pts',(70.0660702936538,-9.34890300397762,
42.8424926294406));
#163112=CARTESIAN_POINT('Ctrl Pts',(69.8893674544513,-9.34479595160383,
42.8700500438711));
#163113=CARTESIAN_POINT('Ctrl Pts',(69.7716182945313,-9.33977680912916,
42.8884730979242));
#163114=CARTESIAN_POINT('Ctrl Pts',(69.4853176391083,-9.32201404737564,
42.9333674531374));
#163115=CARTESIAN_POINT('Ctrl Pts',(69.3169613975907,-9.30686609004303,
42.9598511964446));
#163116=CARTESIAN_POINT('Ctrl Pts',(68.8455710259004,-9.25122078965999,
43.0340980317313));
#163117=CARTESIAN_POINT('Ctrl Pts',(68.5439876103763,-9.20016495741468,
43.0817036702807));
#163118=CARTESIAN_POINT('Ctrl Pts',(67.8669248606584,-9.05028083140165,
43.188258658349));
#163119=CARTESIAN_POINT('Ctrl Pts',(67.4939618036342,-8.94247031749705,
43.2467161332711));
#163120=CARTESIAN_POINT('Ctrl Pts',(67.0056423632166,-8.76708270676925,
43.3225232156578));
#163121=CARTESIAN_POINT('Ctrl Pts',(66.8835136394159,-8.72025049758954,
43.3414211840847));
#163122=CARTESIAN_POINT('Ctrl Pts',(66.6732015555481,-8.63441124246578,
43.3738476573233));
#163123=CARTESIAN_POINT('Ctrl Pts',(66.5845683953219,-8.59660041560209,
43.3874766276869));
#163124=CARTESIAN_POINT('Ctrl Pts',(66.3995919563377,-8.51423282012452,
43.4158403043125));
#163125=CARTESIAN_POINT('Ctrl Pts',(66.3033884763813,-8.46938661504602,
43.4305454313516));
#163126=CARTESIAN_POINT('Ctrl Pts',(66.0369807405777,-8.33954956662249,
43.4711363882876));
#163127=CARTESIAN_POINT('Ctrl Pts',(65.8685543850078,-8.25091694285604,
43.4966462363669));
#163128=CARTESIAN_POINT('Ctrl Pts',(65.4736948571926,-8.02727794998775,
43.5561092902592));
#163129=CARTESIAN_POINT('Ctrl Pts',(65.2499980976918,-7.88763394094255,
43.5895148293524));
#163130=CARTESIAN_POINT('Ctrl Pts',(64.6514617240409,-7.47747101488621,
43.6783044346424));
#163131=CARTESIAN_POINT('Ctrl Pts',(64.2901615842566,-7.18801661849064,
43.7312019642404));
#163132=CARTESIAN_POINT('Ctrl Pts',(63.889825154664,-6.81495433001514,43.7898063872883));
#163133=CARTESIAN_POINT('Ctrl Pts',(63.828743787318,-6.75645643225552,43.7987487232169));
#163134=CARTESIAN_POINT('Ctrl Pts',(63.7287348522407,-6.65802457002916,
43.8134008274902));
#163135=CARTESIAN_POINT('Ctrl Pts',(63.6893573028171,-6.61856428309217,
43.8191730154925));
#163136=CARTESIAN_POINT('Ctrl Pts',(63.6038732356581,-6.53134496740896,
43.8317127601257));
#163137=CARTESIAN_POINT('Ctrl Pts',(63.5579173868938,-6.48344068798444,
43.838459179878));
#163138=CARTESIAN_POINT('Ctrl Pts',(63.412529346836,-6.32860560631025,43.8598083270838));
#163139=CARTESIAN_POINT('Ctrl Pts',(63.3150797588329,-6.2198049361081,43.8741268562085));
#163140=CARTESIAN_POINT('Ctrl Pts',(63.0681569641835,-5.93074023115142,
43.9103436083298));
#163141=CARTESIAN_POINT('Ctrl Pts',(62.9228009974106,-5.74701702744547,
43.9315969026629));
#163142=CARTESIAN_POINT('Ctrl Pts',(62.4900873407863,-5.15581693893105,
43.9942670015785));
#163143=CARTESIAN_POINT('Ctrl Pts',(62.2280082134259,-4.73047887605852,
44.031273141868));
#163144=CARTESIAN_POINT('Ctrl Pts',(61.9386266594116,-4.16498198074783,
44.0697887759788));
#163145=CARTESIAN_POINT('Ctrl Pts',(61.879285033914,-4.04257807511931,44.0775327604615));
#163146=CARTESIAN_POINT('Ctrl Pts',(61.7818807877135,-3.83011562015318,
44.0899541654868));
#163147=CARTESIAN_POINT('Ctrl Pts',(61.7425421561281,-3.74068146336149,
44.0948798755865));
#163148=CARTESIAN_POINT('Ctrl Pts',(61.6636111777775,-3.55343223335918,
44.1045638825173));
#163149=CARTESIAN_POINT('Ctrl Pts',(61.6242539690045,-3.45553064094592,
44.1092768688037));
#163150=CARTESIAN_POINT('Ctrl Pts',(61.5217424197407,-3.18770458761023,
44.1212227418835));
#163151=CARTESIAN_POINT('Ctrl Pts',(61.461801847782,-3.01657194478436,44.1278335525662));
#163152=CARTESIAN_POINT('Ctrl Pts',(61.3349750565256,-2.61826730025979,
44.1408997639938));
#163153=CARTESIAN_POINT('Ctrl Pts',(61.2716028887318,-2.39008461889601,
44.1466854827862));
#163154=CARTESIAN_POINT('Ctrl Pts',(61.0970033232018,-1.6560314643066,44.1600679346971));
#163155=CARTESIAN_POINT('Ctrl Pts',(61.0185350430739,-1.14326162752896,
44.1616014611584));
#163156=CARTESIAN_POINT('Ctrl Pts',(60.9738796242,-0.505365600360473,44.1551322452979));
#163157=CARTESIAN_POINT('Ctrl Pts',(60.9677242252422,-0.383865383910097,
44.1535310365709));
#163158=CARTESIAN_POINT('Ctrl Pts',(60.9623991499425,-0.213903533781448,
44.1507983168674));
#163159=CARTESIAN_POINT('Ctrl Pts',(60.9612549119819,-0.165511012761847,
44.1499644609149));
#163160=CARTESIAN_POINT('Ctrl Pts',(60.9598598539427,-0.0780863857449693,
44.1483592250798));
#163161=CARTESIAN_POINT('Ctrl Pts',(60.9594790287912,-0.0390670884311103,
44.1476072249968));
#163162=CARTESIAN_POINT('Ctrl Pts',(60.9593400679932,-3.72638318321969E-5,
44.1468200349313));
#163163=CARTESIAN_POINT('Origin',(69.6316151486327,0.,39.48523201752));
#163164=CARTESIAN_POINT('',(61.3760955617941,-2.33157398522526E-12,46.5103578905782));
#163165=CARTESIAN_POINT('',(61.3466300729431,3.3917537450853E-10,46.3432507993513));
#163166=CARTESIAN_POINT('',(60.4236626579685,-1.14504475720278E-15,41.1088424787055));
#163167=CARTESIAN_POINT('Ctrl Pts',(61.3760955617941,-4.66200292569332E-12,
46.5103578905782));
#163168=CARTESIAN_POINT('Ctrl Pts',(61.3759092912817,0.0523757248735538,
46.5093014980081));
#163169=CARTESIAN_POINT('Ctrl Pts',(61.3761587903896,0.104750688469651,
46.5081821108365));
#163170=CARTESIAN_POINT('Ctrl Pts',(61.3780382048011,0.24844019208441,46.5049337758213));
#163171=CARTESIAN_POINT('Ctrl Pts',(61.3805567471265,0.339734329378578,
46.5026733604136));
#163172=CARTESIAN_POINT('Ctrl Pts',(61.3969927484521,0.730209909702223,
46.4921281641318));
#163173=CARTESIAN_POINT('Ctrl Pts',(61.4237970986573,1.02861563446639,46.4818594483999));
#163174=CARTESIAN_POINT('Ctrl Pts',(61.5488534409189,1.93587297908879,46.443054388668));
#163175=CARTESIAN_POINT('Ctrl Pts',(61.6923914844532,2.53644451156582,46.4066949979011));
#163176=CARTESIAN_POINT('Ctrl Pts',(61.9363505483461,3.24398340818751,46.3489509174635));
#163177=CARTESIAN_POINT('Ctrl Pts',(61.9824078420049,3.36892239095129,46.3381664069915));
#163178=CARTESIAN_POINT('Ctrl Pts',(62.0666007587671,3.58323118613733,46.3186331981672));
#163179=CARTESIAN_POINT('Ctrl Pts',(62.1035111036226,3.67308080805578,46.3101226004056));
#163180=CARTESIAN_POINT('Ctrl Pts',(62.1836256095551,3.85983654692565,46.291754289559));
#163181=CARTESIAN_POINT('Ctrl Pts',(62.2270901101491,3.9566108614179,46.2818461710201));
#163182=CARTESIAN_POINT('Ctrl Pts',(62.3518621916264,4.22230729476755,46.2535555269216));
#163183=CARTESIAN_POINT('Ctrl Pts',(62.4365708269919,4.38950541783899,46.2345138246346));
#163184=CARTESIAN_POINT('Ctrl Pts',(62.6487579129455,4.7789416004206,46.1872078590987));
#163185=CARTESIAN_POINT('Ctrl Pts',(62.7804148627706,4.99863117742488,46.1581465729979));
#163186=CARTESIAN_POINT('Ctrl Pts',(63.1836407772189,5.6127460169362,46.0701076307508));
#163187=CARTESIAN_POINT('Ctrl Pts',(63.4765194455713,5.99162641785026,46.0072419071673));
#163188=CARTESIAN_POINT('Ctrl Pts',(63.8525971093574,6.4071830179322,45.9286142466717));
#163189=CARTESIAN_POINT('Ctrl Pts',(63.9090279660292,6.46787318500417,45.9168663315544));
#163190=CARTESIAN_POINT('Ctrl Pts',(64.0044648730185,6.56777602463498,45.8970898214856));
#163191=CARTESIAN_POINT('Ctrl Pts',(64.0430255111711,6.607419692317,45.8891236809642));
#163192=CARTESIAN_POINT('Ctrl Pts',(64.1288960647629,6.69412421921133,45.8714393256397));
#163193=CARTESIAN_POINT('Ctrl Pts',(64.1763625683649,6.7410199309346,45.8616994205242));
#163194=CARTESIAN_POINT('Ctrl Pts',(64.3320298421017,6.89150426937819,45.8298597528093));
#163195=CARTESIAN_POINT('Ctrl Pts',(64.4422222633373,6.99293746963674,45.8074787856536));
#163196=CARTESIAN_POINT('Ctrl Pts',(64.7390847999251,7.25309741080842,45.7474910223817));
#163197=CARTESIAN_POINT('Ctrl Pts',(64.9296440427546,7.4070626669649,45.7092883500508));
#163198=CARTESIAN_POINT('Ctrl Pts',(65.5046650375672,7.83480318997433,45.5944528961943));
#163199=CARTESIAN_POINT('Ctrl Pts',(65.9040388206625,8.0864675925758,45.515208836139));
#163200=CARTESIAN_POINT('Ctrl Pts',(66.4402571341688,8.36901326543865,45.4085693128488));
#163201=CARTESIAN_POINT('Ctrl Pts',(66.5613657258613,8.42941865289867,45.3844723012947));
#163202=CARTESIAN_POINT('Ctrl Pts',(66.7709729147365,8.52819061414457,45.3427330328278));
#163203=CARTESIAN_POINT('Ctrl Pts',(66.8588398441722,8.56789991570893,45.3252262025234));
#163204=CARTESIAN_POINT('Ctrl Pts',(67.0422541938191,8.64729907022667,45.2886584668199));
#163205=CARTESIAN_POINT('Ctrl Pts',(67.1378787457414,8.6867678189917,45.2695804336307));
#163206=CARTESIAN_POINT('Ctrl Pts',(67.3979329828805,8.78893599513318,45.2176594235434));
#163207=CARTESIAN_POINT('Ctrl Pts',(67.5635026141149,8.84848016295777,45.1845620049626));
#163208=CARTESIAN_POINT('Ctrl Pts',(68.4850063000921,9.14986299707237,45.0001556968078));
#163209=CARTESIAN_POINT('Ctrl Pts',(69.2673285342023,9.29586948249292,44.8425568081824));
#163210=CARTESIAN_POINT('Ctrl Pts',(70.1575257205164,9.34275452113109,44.6654754883752));
#163211=CARTESIAN_POINT('Ctrl Pts',(70.2565311917286,9.34633087032884,44.6458167574969));
#163212=CARTESIAN_POINT('Ctrl Pts',(70.4106457366081,9.34935112906579,44.6152862706049));
#163213=CARTESIAN_POINT('Ctrl Pts',(70.4657200737278,9.34992484502258,44.60438997345));
#163214=CARTESIAN_POINT('Ctrl Pts',(70.5734268766219,9.35005829707073,44.5831114312398));
#163215=CARTESIAN_POINT('Ctrl Pts',(70.6260567078356,9.34966202131723,44.572728536323));
#163216=CARTESIAN_POINT('Ctrl Pts',(70.7654478362208,9.34739016876703,44.545263405391));
#163217=CARTESIAN_POINT('Ctrl Pts',(70.8521956968284,9.34472181099317,44.5282059248447));
#163218=CARTESIAN_POINT('Ctrl Pts',(71.2873535446512,9.32503833715148,44.4427760506991));
#163219=CARTESIAN_POINT('Ctrl Pts',(71.6347226429596,9.28904679440901,44.3750115881413));
#163220=CARTESIAN_POINT('Ctrl Pts',(72.5082696565916,9.14693220932724,44.2045650957269));
#163221=CARTESIAN_POINT('Ctrl Pts',(73.0288767306544,9.01384622354657,44.1029029096697));
#163222=CARTESIAN_POINT('Ctrl Pts',(73.6670893501812,8.78862670332058,43.9769296012621));
#163223=CARTESIAN_POINT('Ctrl Pts',(73.7981798643658,8.73891257747038,43.9509841054947));
#163224=CARTESIAN_POINT('Ctrl Pts',(74.0172507323125,8.64996113655744,43.9074935005626));
#163225=CARTESIAN_POINT('Ctrl Pts',(74.1058418891245,8.61233445828667,43.8898690034339));
#163226=CARTESIAN_POINT('Ctrl Pts',(74.2866766983746,8.53210614902453,43.853814134279));
#163227=CARTESIAN_POINT('Ctrl Pts',(74.3788394554398,8.4893501038429,43.8353954761207));
#163228=CARTESIAN_POINT('Ctrl Pts',(74.6201102220708,8.37245601451012,43.7870621878547));
#163229=CARTESIAN_POINT('Ctrl Pts',(74.767958316516,8.29573370763082,43.7573251629681));
#163230=CARTESIAN_POINT('Ctrl Pts',(75.013452780197,8.15964903507803,43.7077555450065));
#163231=CARTESIAN_POINT('Ctrl Pts',(75.1122156426323,8.10244687622636,43.687759333083));
#163232=CARTESIAN_POINT('Ctrl Pts',(75.5499763567009,7.83778768918829,43.5989008626704));
#163233=CARTESIAN_POINT('Ctrl Pts',(75.8765450893125,7.60996207728207,43.5319740024443));
#163234=CARTESIAN_POINT('Ctrl Pts',(76.3886521989549,7.20067086027229,43.4265069844938));
#163235=CARTESIAN_POINT('Ctrl Pts',(76.5829946908649,7.03149106693584,43.386350993485));
#163236=CARTESIAN_POINT('Ctrl Pts',(76.8281777448555,6.79930552812252,43.3357030462511));
#163237=CARTESIAN_POINT('Ctrl Pts',(76.8854936490011,6.7436003221825,43.3238644243163));
#163238=CARTESIAN_POINT('Ctrl Pts',(76.9810194883662,6.64832139344032,43.3041440306437));
#163239=CARTESIAN_POINT('Ctrl Pts',(77.0196032349987,6.60914585381322,43.2961820691352));
#163240=CARTESIAN_POINT('Ctrl Pts',(77.1054422415198,6.52042450556793,43.278477578197));
#163241=CARTESIAN_POINT('Ctrl Pts',(77.1525053984017,6.47069052590961,43.2687760115412));
#163242=CARTESIAN_POINT('Ctrl Pts',(77.308967672514,6.30163712528161,43.2365284926531));
#163243=CARTESIAN_POINT('Ctrl Pts',(77.4158435767006,6.17992379094053,43.2145098879679));
#163244=CARTESIAN_POINT('Ctrl Pts',(77.6992878807435,5.83956577684957,43.1560122689862));
#163245=CARTESIAN_POINT('Ctrl Pts',(77.8693191906816,5.61549014546257,43.1208019706101));
#163246=CARTESIAN_POINT('Ctrl Pts',(78.2645139546696,5.04251194527642,43.0381398347686));
#163247=CARTESIAN_POINT('Ctrl Pts',(78.4771699789188,4.6854246407792,42.9928731076335));
#163248=CARTESIAN_POINT('Ctrl Pts',(78.72913729618,4.1899388385151,42.9374903421954));
#163249=CARTESIAN_POINT('Ctrl Pts',(78.7899403351605,4.06340615894743,42.923960032166));
#163250=CARTESIAN_POINT('Ctrl Pts',(78.8879825521177,3.84704605053116,42.9018346729445));
#163251=CARTESIAN_POINT('Ctrl Pts',(78.9267019681156,3.75794014902173,42.8930053765545));
#163252=CARTESIAN_POINT('Ctrl Pts',(79.0037602197051,3.57278227447287,42.8752345638923));
#163253=CARTESIAN_POINT('Ctrl Pts',(79.0419108728264,3.47666356446806,42.8663232308247));
#163254=CARTESIAN_POINT('Ctrl Pts',(79.1387714573907,3.22035477802494,42.8433835799918));
#163255=CARTESIAN_POINT('Ctrl Pts',(79.1947308873815,3.05912875198699,42.8297930039927));
#163256=CARTESIAN_POINT('Ctrl Pts',(79.4942260903285,2.1139608666272,42.754962549496));
#163257=CARTESIAN_POINT('Ctrl Pts',(79.6390112382053,1.30132120338144,42.7093879101799));
#163258=CARTESIAN_POINT('Ctrl Pts',(79.6821495521564,0.379258996189193,
42.6813477226864));
#163259=CARTESIAN_POINT('Ctrl Pts',(79.6852556293486,0.278907727998995,
42.6786115198587));
#163260=CARTESIAN_POINT('Ctrl Pts',(79.6876255680066,0.122509079759497,
42.6748527185915));
#163261=CARTESIAN_POINT('Ctrl Pts',(79.6879809167348,0.0664910649123827,
42.6736074044482));
#163262=CARTESIAN_POINT('Ctrl Pts',(79.6877110157052,-0.0432453595123394,
42.6713690019725));
#163263=CARTESIAN_POINT('Ctrl Pts',(79.6871255268144,-0.0969613195950516,
42.6703678807929));
#163264=CARTESIAN_POINT('Ctrl Pts',(79.6843675992852,-0.239514859363793,
42.6679575682373));
#163265=CARTESIAN_POINT('Ctrl Pts',(79.6814077112249,-0.328334563163165,
42.6667098978525));
#163266=CARTESIAN_POINT('Ctrl Pts',(79.6592055443577,-0.797422543436576,
42.6614231723899));
#163267=CARTESIAN_POINT('Ctrl Pts',(79.6184334884666,-1.1763568640383,42.6616689264385));
#163268=CARTESIAN_POINT('Ctrl Pts',(79.4690907847104,-2.06056441786296,
42.6716831507418));
#163269=CARTESIAN_POINT('Ctrl Pts',(79.3418353239273,-2.56138014471964,
42.6847536373139));
#163270=CARTESIAN_POINT('Ctrl Pts',(79.1276289779917,-3.18542652518842,
42.7096457391364));
#163271=CARTESIAN_POINT('Ctrl Pts',(79.0777278396359,-3.32064257997726,
42.7155828657619));
#163272=CARTESIAN_POINT('Ctrl Pts',(78.9887271607178,-3.5457915028773,42.7263769393121));
#163273=CARTESIAN_POINT('Ctrl Pts',(78.9512821880452,-3.63636332207318,
42.7309715622235));
#163274=CARTESIAN_POINT('Ctrl Pts',(78.871731083482,-3.82059426311495,42.7408352184964));
#163275=CARTESIAN_POINT('Ctrl Pts',(78.8294930825966,-3.91418092044108,
42.7461253227874));
#163276=CARTESIAN_POINT('Ctrl Pts',(78.7148205908441,-4.15757261687448,
42.7606206130241));
#163277=CARTESIAN_POINT('Ctrl Pts',(78.6399408073153,-4.30616148146556,
42.7702142684695));
#163278=CARTESIAN_POINT('Ctrl Pts',(78.4603921507384,-4.64012511377814,
42.7935081386222));
#163279=CARTESIAN_POINT('Ctrl Pts',(78.3533019401944,-4.82406594952968,
42.8075989390933));
#163280=CARTESIAN_POINT('Ctrl Pts',(78.0634210453297,-5.28524572843818,
42.8462958433948));
#163281=CARTESIAN_POINT('Ctrl Pts',(77.8720634162778,-5.55662635508195,
42.8723346140961));
#163282=CARTESIAN_POINT('Ctrl Pts',(77.5163563503823,-6.00826518082021,
42.9219010890529));
#163283=CARTESIAN_POINT('Ctrl Pts',(77.3585241201728,-6.19337025792796,
42.944234256554));
#163284=CARTESIAN_POINT('Ctrl Pts',(77.1410090962564,-6.42924515223729,
42.9755993320967));
#163285=CARTESIAN_POINT('Ctrl Pts',(77.0875455247921,-6.48579069705593,
42.9833525042654));
#163286=CARTESIAN_POINT('Ctrl Pts',(76.9950658439429,-6.58119141694582,
42.9968452903587));
#163287=CARTESIAN_POINT('Ctrl Pts',(76.9563953201769,-6.62038545717565,
43.0025113066169));
#163288=CARTESIAN_POINT('Ctrl Pts',(76.8673651571803,-6.70904220996541,
43.0156110693333));
#163289=CARTESIAN_POINT('Ctrl Pts',(76.8167910862964,-6.75827653459227,
43.0230909207361));
#163290=CARTESIAN_POINT('Ctrl Pts',(76.6379509055128,-6.92847471202823,
43.0496602949232));
#163291=CARTESIAN_POINT('Ctrl Pts',(76.5068683924809,-7.04633011891058,
43.0693444007298));
#163292=CARTESIAN_POINT('Ctrl Pts',(76.1223514603993,-7.37278962727507,
43.1275032680691));
#163293=CARTESIAN_POINT('Ctrl Pts',(75.8612509584303,-7.57167544923386,
43.167483332251));
#163294=CARTESIAN_POINT('Ctrl Pts',(75.2761365725286,-7.97010843562931,
43.2574095030625));
#163295=CARTESIAN_POINT('Ctrl Pts',(74.9492903242468,-8.16431366405078,
43.3078355788));
#163296=CARTESIAN_POINT('Ctrl Pts',(74.5000885771895,-8.39491934386381,
43.3769763652317));
#163297=CARTESIAN_POINT('Ctrl Pts',(74.3874663439199,-8.44985778293434,
43.3942999390171));
#163298=CARTESIAN_POINT('Ctrl Pts',(74.186694130876,-8.54276477195986,43.4251529447234));
#163299=CARTESIAN_POINT('Ctrl Pts',(74.0989983955568,-8.5816898511644,43.438619538588));
#163300=CARTESIAN_POINT('Ctrl Pts',(73.911534104962,-8.66140671936107,43.4673827619334));
#163301=CARTESIAN_POINT('Ctrl Pts',(73.8116268976164,-8.7018289332096,43.4826977093368));
#163302=CARTESIAN_POINT('Ctrl Pts',(73.5261941193496,-8.8115049904056,43.5264101725597));
#163303=CARTESIAN_POINT('Ctrl Pts',(73.3391333662533,-8.87651460606896,
43.5550068319848));
#163304=CARTESIAN_POINT('Ctrl Pts',(72.8902457720778,-9.01640029302703,
43.62353071672));
#163305=CARTESIAN_POINT('Ctrl Pts',(72.626923534052,-9.08575538223764,43.6636471481403));
#163306=CARTESIAN_POINT('Ctrl Pts',(71.9172353002217,-9.23922979413597,
43.7717497780101));
#163307=CARTESIAN_POINT('Ctrl Pts',(71.4671177111447,-9.30202562047584,
43.8402774469245));
#163308=CARTESIAN_POINT('Ctrl Pts',(70.8921769577753,-9.33900976848062,
43.9286193641354));
#163309=CARTESIAN_POINT('Ctrl Pts',(70.7698449820668,-9.34441377493864,
43.947464509943));
#163310=CARTESIAN_POINT('Ctrl Pts',(70.5877488657143,-9.34879410333581,
43.9756142279267));
#163311=CARTESIAN_POINT('Ctrl Pts',(70.528034374026,-9.34964483694112,43.9848610024013));
#163312=CARTESIAN_POINT('Ctrl Pts',(70.4172972151225,-9.35013650285605,
44.0020416961283));
#163313=CARTESIAN_POINT('Ctrl Pts',(70.366277578649,-9.34993553400781,44.0099707579248));
#163314=CARTESIAN_POINT('Ctrl Pts',(70.2395058105395,-9.34837380559993,
44.0297033407116));
#163315=CARTESIAN_POINT('Ctrl Pts',(70.1637658835072,-9.34649781050369,
44.041519525266));
#163316=CARTESIAN_POINT('Ctrl Pts',(69.8253223539133,-9.3338984027968,44.0944177141589));
#163317=CARTESIAN_POINT('Ctrl Pts',(69.5631570128807,-9.31277313229554,
44.1356544586938));
#163318=CARTESIAN_POINT('Ctrl Pts',(68.8376199124167,-9.22263993462805,
44.2499606108062));
#163319=CARTESIAN_POINT('Ctrl Pts',(68.3780312779604,-9.12925636895317,
44.3225503403547));
#163320=CARTESIAN_POINT('Ctrl Pts',(67.6887129841414,-8.93312670244812,
44.4305006617752));
#163321=CARTESIAN_POINT('Ctrl Pts',(67.4528842588676,-8.85555083519632,
44.4672672559396));
#163322=CARTESIAN_POINT('Ctrl Pts',(67.1122192914184,-8.72796457053197,
44.5200427427298));
#163323=CARTESIAN_POINT('Ctrl Pts',(67.0048034773589,-8.68540886517917,
44.5366338064274));
#163324=CARTESIAN_POINT('Ctrl Pts',(66.8103642404619,-8.60410466439594,
44.5665691728336));
#163325=CARTESIAN_POINT('Ctrl Pts',(66.7230932753129,-8.56601080044907,
44.5799688416452));
#163326=CARTESIAN_POINT('Ctrl Pts',(66.5304168652247,-8.47832431403028,
44.6094695718655));
#163327=CARTESIAN_POINT('Ctrl Pts',(66.425321097703,-8.42806878166995,44.6255045429834));
#163328=CARTESIAN_POINT('Ctrl Pts',(66.0870544992686,-8.25836387378462,
44.6769327109813));
#163329=CARTESIAN_POINT('Ctrl Pts',(65.85791147279,-8.13092142876955,44.7114798652892));
#163330=CARTESIAN_POINT('Ctrl Pts',(65.2106574721794,-7.73399611934188,
44.8083280265073));
#163331=CARTESIAN_POINT('Ctrl Pts',(64.8081238675418,-7.44015758791296,
44.8675887806537));
#163332=CARTESIAN_POINT('Ctrl Pts',(64.3140836543493,-7.01464388161671,
44.9399782808404));
#163333=CARTESIAN_POINT('Ctrl Pts',(64.1998672259736,-6.91121300416874,
44.9566912980124));
#163334=CARTESIAN_POINT('Ctrl Pts',(64.0373931684379,-6.75655247588688,
44.9804794082859));
#163335=CARTESIAN_POINT('Ctrl Pts',(63.987082226343,-6.70756232085959,44.9878475705288));
#163336=CARTESIAN_POINT('Ctrl Pts',(63.9022223678176,-6.62303508899495,
45.0002847078665));
#163337=CARTESIAN_POINT('Ctrl Pts',(63.8673969778365,-6.58778690016492,
45.0053918269112));
#163338=CARTESIAN_POINT('Ctrl Pts',(63.7812085642904,-6.4991456541875,45.018038219508));
#163339=CARTESIAN_POINT('Ctrl Pts',(63.7301957853784,-6.44541112584493,
45.0255289107896));
#163340=CARTESIAN_POINT('Ctrl Pts',(63.5386475524898,-6.23875699660736,
45.0536598384338));
#163341=CARTESIAN_POINT('Ctrl Pts',(63.4025573844755,-6.08171362542834,
45.0736538291482));
#163342=CARTESIAN_POINT('Ctrl Pts',(62.9739281766282,-5.55240163661811,
45.1363444327762));
#163343=CARTESIAN_POINT('Ctrl Pts',(62.7041930776312,-5.16220129278606,
45.1752995661453));
#163344=CARTESIAN_POINT('Ctrl Pts',(62.3451261146196,-4.54851625783205,
45.2250930539875));
#163345=CARTESIAN_POINT('Ctrl Pts',(62.2331903127512,-4.33952581898627,
45.2402355760548));
#163346=CARTESIAN_POINT('Ctrl Pts',(62.0792078773349,-4.02408501036952,
45.2603784013492));
#163347=CARTESIAN_POINT('Ctrl Pts',(62.0310743071458,-3.92078947451051,
45.2665599073768));
#163348=CARTESIAN_POINT('Ctrl Pts',(61.9457935966874,-3.72879914958888,
45.2772850380384));
#163349=CARTESIAN_POINT('Ctrl Pts',(61.9081119811342,-3.64036456271324,
45.2819329122069));
#163350=CARTESIAN_POINT('Ctrl Pts',(61.8262837521819,-3.43992300574851,
45.2918109057193));
#163351=CARTESIAN_POINT('Ctrl Pts',(61.782909377705,-3.32761196173122,45.29689148475));
#163352=CARTESIAN_POINT('Ctrl Pts',(61.6458653499301,-2.95162044430915,
45.3124005711507));
#163353=CARTESIAN_POINT('Ctrl Pts',(61.5616940643353,-2.68456528383426,
45.3209931751147));
#163354=CARTESIAN_POINT('Ctrl Pts',(61.3542858775893,-1.90844276427591,
45.3392348352261));
#163355=CARTESIAN_POINT('Ctrl Pts',(61.2611201549604,-1.39230848186249,
45.343229002781));
#163356=CARTESIAN_POINT('Ctrl Pts',(61.1930492975319,-0.683822521086543,
45.3389844111742));
#163357=CARTESIAN_POINT('Ctrl Pts',(61.1806351028151,-0.495995502835025,
45.3369498217409));
#163358=CARTESIAN_POINT('Ctrl Pts',(61.1712554465341,-0.236655462932668,
45.3329687035681));
#163359=CARTESIAN_POINT('Ctrl Pts',(61.1694840595521,-0.165349282080866,
45.3317522351483));
#163360=CARTESIAN_POINT('Ctrl Pts',(61.1680967670258,-0.0626889790138221,
45.3298304263121));
#163361=CARTESIAN_POINT('Ctrl Pts',(61.1678292235918,-0.0313446475437261,
45.3292207930631));
#163362=CARTESIAN_POINT('Ctrl Pts',(61.1677177485993,-1.53755753856922E-9,
45.3285885869945));
#163363=CARTESIAN_POINT('Ctrl Pts',(61.1382522597423,8.24276059806775E-10,
45.1614814957336));
#163364=CARTESIAN_POINT('Ctrl Pts',(61.1383891918146,-0.0385026941639486,
45.1622580761255));
#163365=CARTESIAN_POINT('Ctrl Pts',(61.1387590575512,-0.0770049839012811,
45.1629861025056));
#163366=CARTESIAN_POINT('Ctrl Pts',(61.140569995889,-0.192648155176659,
45.1650288677117));
#163367=CARTESIAN_POINT('Ctrl Pts',(61.1427135671748,-0.269777112292349,
45.1661989697657));
#163368=CARTESIAN_POINT('Ctrl Pts',(61.1567253435757,-0.620565322579443,
45.1706684012576));
#163369=CARTESIAN_POINT('Ctrl Pts',(61.1794464992234,-0.893682308946226,
45.1717893024998));
#163370=CARTESIAN_POINT('Ctrl Pts',(61.2740426684191,-1.63919965951693,
45.1689294731104));
#163371=CARTESIAN_POINT('Ctrl Pts',(61.3697656685128,-2.10770871118466,
45.1605693737304));
#163372=CARTESIAN_POINT('Ctrl Pts',(61.5666335727138,-2.79967176878799,
45.1393888259066));
#163373=CARTESIAN_POINT('Ctrl Pts',(61.6417695656924,-3.02981523768952,
45.1307994313242));
#163374=CARTESIAN_POINT('Ctrl Pts',(61.7656403153891,-3.36499433576385,
45.1160601589259));
#163375=CARTESIAN_POINT('Ctrl Pts',(61.8076135640718,-3.47246663252628,
45.1109854684186));
#163376=CARTESIAN_POINT('Ctrl Pts',(61.8881269110202,-3.66796089670592,
45.1011163549103));
#163377=CARTESIAN_POINT('Ctrl Pts',(61.9260631385096,-3.75621926596353,
45.0964174526486));
#163378=CARTESIAN_POINT('Ctrl Pts',(62.0138970825754,-3.95225062666079,
45.0854344918741));
#163379=CARTESIAN_POINT('Ctrl Pts',(62.0644941531437,-4.05968573230524,
45.0790393923797));
#163380=CARTESIAN_POINT('Ctrl Pts',(62.239146779262,-4.41304384895806,45.0567450957195));
#163381=CARTESIAN_POINT('Ctrl Pts',(62.3719233204807,-4.65440542066785,
45.0394581002291));
#163382=CARTESIAN_POINT('Ctrl Pts',(62.8100961257201,-5.37421576032888,
44.9813042080612));
#163383=CARTESIAN_POINT('Ctrl Pts',(63.1481812897066,-5.83078601011641,
44.9350672797241));
#163384=CARTESIAN_POINT('Ctrl Pts',(63.5948561883113,-6.33206780464021,
44.8711589950957));
#163385=CARTESIAN_POINT('Ctrl Pts',(63.6661304719093,-6.4093938041916,44.8608852320421));
#163386=CARTESIAN_POINT('Ctrl Pts',(63.7795725608885,-6.52838446585308,
44.8443995067381));
#163387=CARTESIAN_POINT('Ctrl Pts',(63.8208729940886,-6.57088939356122,
44.8383708882797));
#163388=CARTESIAN_POINT('Ctrl Pts',(63.9046311568014,-6.65546853676753,
44.8260874874132));
#163389=CARTESIAN_POINT('Ctrl Pts',(63.9470939155611,-6.69753363585606,
44.8198315201332));
#163390=CARTESIAN_POINT('Ctrl Pts',(64.0672577477718,-6.81431041144412,
44.8020552325157));
#163391=CARTESIAN_POINT('Ctrl Pts',(64.1458378504009,-6.88807497182399,
44.7903469753841));
#163392=CARTESIAN_POINT('Ctrl Pts',(64.3344021540265,-7.05903407154023,
44.7620897971016));
#163393=CARTESIAN_POINT('Ctrl Pts',(64.4454210403231,-7.15500852082844,
44.7453283414892));
#163394=CARTESIAN_POINT('Ctrl Pts',(64.9459658873624,-7.56743555634622,
44.6693607796848));
#163395=CARTESIAN_POINT('Ctrl Pts',(65.3580806882549,-7.85431584746642,
44.6058294181406));
#163396=CARTESIAN_POINT('Ctrl Pts',(65.9739878810786,-8.212460373497,44.5109478837378));
#163397=CARTESIAN_POINT('Ctrl Pts',(66.1604226371677,-8.31244403231903,
44.4822282192156));
#163398=CARTESIAN_POINT('Ctrl Pts',(66.4483600754999,-8.45430807339837,
44.4379345689287));
#163399=CARTESIAN_POINT('Ctrl Pts',(66.5474816423781,-8.50096155074436,
44.4226970802018));
#163400=CARTESIAN_POINT('Ctrl Pts',(66.7346528701072,-8.58500281343704,
44.3939497327629));
#163401=CARTESIAN_POINT('Ctrl Pts',(66.8225020233732,-8.62281039569729,
44.3804674276224));
#163402=CARTESIAN_POINT('Ctrl Pts',(67.0257915614878,-8.70656071478264,
44.34929467749));
#163403=CARTESIAN_POINT('Ctrl Pts',(67.14159978068,-8.75154299209778,44.3315557445542));
#163404=CARTESIAN_POINT('Ctrl Pts',(67.5623515620808,-8.90521351337595,
44.2671771107874));
#163405=CARTESIAN_POINT('Ctrl Pts',(67.8720017372156,-9.00006157120899,
44.2199374741881));
#163406=CARTESIAN_POINT('Ctrl Pts',(68.4640910832926,-9.14764165091881,
44.1297196239163));
#163407=CARTESIAN_POINT('Ctrl Pts',(68.7452919938032,-9.20386192961857,
44.0869155835871));
#163408=CARTESIAN_POINT('Ctrl Pts',(69.33776452813,-9.29363307788184,43.9965469013414));
#163409=CARTESIAN_POINT('Ctrl Pts',(69.6490632617353,-9.32459034501279,
43.9489615363812));
#163410=CARTESIAN_POINT('Ctrl Pts',(70.0534515474975,-9.34395539089209,
43.8866856019446));
#163411=CARTESIAN_POINT('Ctrl Pts',(70.1457040579469,-9.34697331193446,
43.8724472339339));
#163412=CARTESIAN_POINT('Ctrl Pts',(70.2919491944493,-9.34954033073362,
43.8498135742253));
#163413=CARTESIAN_POINT('Ctrl Pts',(70.3459239123,-9.35000930398093,43.8414467772714));
#163414=CARTESIAN_POINT('Ctrl Pts',(70.4542257209256,-9.34999035428335,
43.8246284789358));
#163415=CARTESIAN_POINT('Ctrl Pts',(70.5085506593413,-9.34949611816943,
43.816177147714));
#163416=CARTESIAN_POINT('Ctrl Pts',(70.6568847672363,-9.34682270338928,
43.7930646466113));
#163417=CARTESIAN_POINT('Ctrl Pts',(70.7508662883036,-9.34367611460512,
43.7783813699122));
#163418=CARTESIAN_POINT('Ctrl Pts',(71.1734548354196,-9.32298770490505,
43.7122227918697));
#163419=CARTESIAN_POINT('Ctrl Pts',(71.5009892693062,-9.28913858177973,
43.6605838916785));
#163420=CARTESIAN_POINT('Ctrl Pts',(72.3710422288497,-9.15138767381555,
43.5234167040289));
#163421=CARTESIAN_POINT('Ctrl Pts',(72.9073221554565,-9.01586112991982,
43.4389312046817));
#163422=CARTESIAN_POINT('Ctrl Pts',(73.5606217753429,-8.78635140384396,
43.3374077803584));
#163423=CARTESIAN_POINT('Ctrl Pts',(73.69156891526,-8.73695869179434,43.3171272612441));
#163424=CARTESIAN_POINT('Ctrl Pts',(73.911026502517,-8.64840418432932,43.2832679673657));
#163425=CARTESIAN_POINT('Ctrl Pts',(74.0001220585936,-8.61080851366969,
43.2695584759816));
#163426=CARTESIAN_POINT('Ctrl Pts',(74.1824827596076,-8.53044875072412,
43.2415764764608));
#163427=CARTESIAN_POINT('Ctrl Pts',(74.2756613476616,-8.48751518209136,
43.2273220468438));
#163428=CARTESIAN_POINT('Ctrl Pts',(74.5208211787036,-8.36955117402205,
43.1899334610542));
#163429=CARTESIAN_POINT('Ctrl Pts',(74.6715169352929,-8.29185492156071,
43.1670719101866));
#163430=CARTESIAN_POINT('Ctrl Pts',(74.9223226682064,-8.15366977599374,
43.1292185900963));
#163431=CARTESIAN_POINT('Ctrl Pts',(75.0235527925827,-8.09536678830495,
43.1139957886111));
#163432=CARTESIAN_POINT('Ctrl Pts',(75.4782124326391,-7.82190345719705,
43.0458590388681));
#163433=CARTESIAN_POINT('Ctrl Pts',(75.8183541324543,-7.58492369752779,
42.9955600813075));
#163434=CARTESIAN_POINT('Ctrl Pts',(76.3300352707207,-7.17493371267975,
42.9203866492962));
#163435=CARTESIAN_POINT('Ctrl Pts',(76.512452173251,-7.01671503482492,42.8936921021068));
#163436=CARTESIAN_POINT('Ctrl Pts',(76.7467121625727,-6.79695481574242,
42.8593982243701));
#163437=CARTESIAN_POINT('Ctrl Pts',(76.8041618989408,-6.74165395449314,
42.8509867349533));
#163438=CARTESIAN_POINT('Ctrl Pts',(76.9001747992212,-6.64682104063442,
42.8369186825579));
#163439=CARTESIAN_POINT('Ctrl Pts',(76.9391064783845,-6.60767643675937,
42.8312110348119));
#163440=CARTESIAN_POINT('Ctrl Pts',(77.0260472535047,-6.51868824573315,
42.8184562151595));
#163441=CARTESIAN_POINT('Ctrl Pts',(77.0738546905375,-6.46864952745328,
42.8114372410274));
#163442=CARTESIAN_POINT('Ctrl Pts',(77.2341482275809,-6.29708373989492,
42.7878979549438));
#163443=CARTESIAN_POINT('Ctrl Pts',(77.3439742623138,-6.17306294577502,
42.7717610240008));
#163444=CARTESIAN_POINT('Ctrl Pts',(77.6378611362748,-5.82283557549946,
42.7286889049466));
#163445=CARTESIAN_POINT('Ctrl Pts',(77.8147870107264,-5.59075525269269,
42.702888435309));
#163446=CARTESIAN_POINT('Ctrl Pts',(78.2099289152862,-5.01898559763149,
42.6461294373541));
#163447=CARTESIAN_POINT('Ctrl Pts',(78.4177245339355,-4.67263188716936,
42.6170308931888));
#163448=CARTESIAN_POINT('Ctrl Pts',(78.6672884620141,-4.18888980141818,
42.5837208272088));
#163449=CARTESIAN_POINT('Ctrl Pts',(78.7289477644033,-4.06253506423639,
42.5756538627039));
#163450=CARTESIAN_POINT('Ctrl Pts',(78.8285283536836,-3.84638174135585,
42.562928486005));
#163451=CARTESIAN_POINT('Ctrl Pts',(78.8679133782832,-3.75730097016881,
42.5579853493193));
#163452=CARTESIAN_POINT('Ctrl Pts',(78.9464008117894,-3.57211066688893,
42.5483300982718));
#163453=CARTESIAN_POINT('Ctrl Pts',(78.9853133825372,-3.47593325736649,
42.5436545039925));
#163454=CARTESIAN_POINT('Ctrl Pts',(79.0842976154617,-3.21924716498243,
42.5320702487633));
#163455=CARTESIAN_POINT('Ctrl Pts',(79.14161973557,-3.05769704539769,42.525693911188));
#163456=CARTESIAN_POINT('Ctrl Pts',(79.2903895957021,-2.59941208261279,
42.5101399593312));
#163457=CARTESIAN_POINT('Ctrl Pts',(79.3717270832539,-2.29956636865247,
42.5028984416816));
#163458=CARTESIAN_POINT('Ctrl Pts',(79.5517513113485,-1.47858201540354,
42.4906407088634));
#163459=CARTESIAN_POINT('Ctrl Pts',(79.6217739367768,-0.952251686110478,
42.4908670523403));
#163460=CARTESIAN_POINT('Ctrl Pts',(79.6517132336951,-0.333126884221562,
42.4992240432676));
#163461=CARTESIAN_POINT('Ctrl Pts',(79.6547752741753,-0.243274911438908,
42.5006333537901));
#163462=CARTESIAN_POINT('Ctrl Pts',(79.6576221625992,-0.0994862722151973,
42.5031920897253));
#163463=CARTESIAN_POINT('Ctrl Pts',(79.6582280669377,-0.0455690728587685,
42.5042197554209));
#163464=CARTESIAN_POINT('Ctrl Pts',(79.6585211511328,0.0641079833002689,
42.5064459190048));
#163465=CARTESIAN_POINT('Ctrl Pts',(79.6581762866144,0.119865495212415,
42.5076491650542));
#163466=CARTESIAN_POINT('Ctrl Pts',(79.6558480115764,0.274691649171249,
42.5111943210018));
#163467=CARTESIAN_POINT('Ctrl Pts',(79.652799617398,0.373733196296196,42.513694212661));
#163468=CARTESIAN_POINT('Ctrl Pts',(79.6420936919487,0.603874671675038,
42.5200676571738));
#163469=CARTESIAN_POINT('Ctrl Pts',(79.6332603593372,0.734893795255606,
42.524122862127));
#163470=CARTESIAN_POINT('Ctrl Pts',(79.5890380035763,1.23540673627678,42.5413386752479));
#163471=CARTESIAN_POINT('Ctrl Pts',(79.5346595055153,1.60276752291058,42.5575934474194));
#163472=CARTESIAN_POINT('Ctrl Pts',(79.3767974089433,2.35957425469762,42.5995738122192));
#163473=CARTESIAN_POINT('Ctrl Pts',(79.2697139851994,2.74745774704834,42.6259463748392));
#163474=CARTESIAN_POINT('Ctrl Pts',(79.0952985403823,3.25166237822745,42.6672074948404));
#163475=CARTESIAN_POINT('Ctrl Pts',(79.0495943071676,3.37534013457415,42.6779053789683));
#163476=CARTESIAN_POINT('Ctrl Pts',(78.9658154574366,3.58822616531385,42.6973377712738));
#163477=CARTESIAN_POINT('Ctrl Pts',(78.9289197674915,3.67789657022253,42.7058431698303));
#163478=CARTESIAN_POINT('Ctrl Pts',(78.8485560881626,3.86495653900656,42.7242651208208));
#163479=CARTESIAN_POINT('Ctrl Pts',(78.804806064531,3.96220429095443,42.7342362936111));
#163480=CARTESIAN_POINT('Ctrl Pts',(78.6782169860375,4.23127219419301,42.7629326486843));
#163481=CARTESIAN_POINT('Ctrl Pts',(78.5918183775931,4.40128473000045,42.78234768701));
#163482=CARTESIAN_POINT('Ctrl Pts',(78.3739004873866,4.79956818087367,42.8309088357964));
#163483=CARTESIAN_POINT('Ctrl Pts',(78.2378610238797,5.0250721335885,42.8609166741631));
#163484=CARTESIAN_POINT('Ctrl Pts',(77.8369047997137,5.63031275557458,42.9483691811843));
#163485=CARTESIAN_POINT('Ctrl Pts',(77.5531802429082,5.99616976321783,43.0092316426236));
#163486=CARTESIAN_POINT('Ctrl Pts',(77.1871134972828,6.40148009376108,43.0857908745933));
#163487=CARTESIAN_POINT('Ctrl Pts',(77.1297216062,6.46329823634021,43.0977419106633));
#163488=CARTESIAN_POINT('Ctrl Pts',(77.0331855893049,6.56445721735398,43.1177497176243));
#163489=CARTESIAN_POINT('Ctrl Pts',(76.994513494296,6.60425458471733,43.1257402737068));
#163490=CARTESIAN_POINT('Ctrl Pts',(76.9090947140926,6.69058249577736,43.1433343257902));
#163491=CARTESIAN_POINT('Ctrl Pts',(76.8622054028657,6.73696238602991,43.1529575926938));
#163492=CARTESIAN_POINT('Ctrl Pts',(76.7108635985738,6.88347422985578,43.1839190271693));
#163493=CARTESIAN_POINT('Ctrl Pts',(76.6045726332316,6.98161999258863,43.205516447744));
#163494=CARTESIAN_POINT('Ctrl Pts',(76.3225230296137,7.22998628208738,43.2625390633344));
#163495=CARTESIAN_POINT('Ctrl Pts',(76.1433896813764,7.37609803303641,43.2984791375007));
#163496=CARTESIAN_POINT('Ctrl Pts',(75.5629044394448,7.81415511477105,43.4144850285718));
#163497=CARTESIAN_POINT('Ctrl Pts',(75.1436636470306,8.08005791266137,43.4976551122374));
#163498=CARTESIAN_POINT('Ctrl Pts',(74.5869236781629,8.37267567785277,43.6083783553441));
#163499=CARTESIAN_POINT('Ctrl Pts',(74.4669916321185,8.43237178069141,43.6322419022846));
#163500=CARTESIAN_POINT('Ctrl Pts',(74.2587390179006,8.53035451895324,43.6737123006198));
#163501=CARTESIAN_POINT('Ctrl Pts',(74.171026420403,8.56993477055856,43.6911887631566));
#163502=CARTESIAN_POINT('Ctrl Pts',(73.9873057579724,8.6493509348009,43.727818352145));
#163503=CARTESIAN_POINT('Ctrl Pts',(73.8912120669089,8.68894473996208,43.7469904731175));
#163504=CARTESIAN_POINT('Ctrl Pts',(73.6281111760892,8.79210036928979,43.7995212755182));
#163505=CARTESIAN_POINT('Ctrl Pts',(73.4599176114563,8.85237169062116,43.8331448394899));
#163506=CARTESIAN_POINT('Ctrl Pts',(73.0682476616612,8.97977994567656,43.9115281011586));
#163507=CARTESIAN_POINT('Ctrl Pts',(72.8437765954576,9.04330881375593,43.9565136487428));
#163508=CARTESIAN_POINT('Ctrl Pts',(72.3032305367332,9.17391128055197,44.0648946893024));
#163509=CARTESIAN_POINT('Ctrl Pts',(71.9855779059975,9.23281836282717,44.1286303673378));
#163510=CARTESIAN_POINT('Ctrl Pts',(71.396139126813,9.30964010279295,44.2465977655833));
#163511=CARTESIAN_POINT('Ctrl Pts',(71.1253402381074,9.33253167020398,44.300676527649));
#163512=CARTESIAN_POINT('Ctrl Pts',(70.776513484022,9.3461613443158,44.3699569756783));
#163513=CARTESIAN_POINT('Ctrl Pts',(70.6990959858151,9.34818593421559,44.3853085828565));
#163514=CARTESIAN_POINT('Ctrl Pts',(70.5711860171721,9.3498794031418,44.4106247550794));
#163515=CARTESIAN_POINT('Ctrl Pts',(70.5207077770349,9.3501230910819,44.4206030718155));
#163516=CARTESIAN_POINT('Ctrl Pts',(70.4122130108698,9.34973430845383,44.4420209537332));
#163517=CARTESIAN_POINT('Ctrl Pts',(70.3541990466229,9.34896567230278,44.453456220126));
#163518=CARTESIAN_POINT('Ctrl Pts',(70.1817544940958,9.34501381780451,44.4874030365932));
#163519=CARTESIAN_POINT('Ctrl Pts',(70.0673629963074,9.3402093525268,44.5098640163913));
#163520=CARTESIAN_POINT('Ctrl Pts',(69.790844329686,9.32331070217026,44.5640620303458));
#163521=CARTESIAN_POINT('Ctrl Pts',(69.6288787146776,9.30900652781442,44.5957269268059));
#163522=CARTESIAN_POINT('Ctrl Pts',(69.1579534102891,9.25454516109661,44.6876956112489));
#163523=CARTESIAN_POINT('Ctrl Pts',(68.8505087791426,9.20274418269688,44.7476180663682));
#163524=CARTESIAN_POINT('Ctrl Pts',(68.1686521773753,9.05119811535233,44.8808490024888));
#163525=CARTESIAN_POINT('Ctrl Pts',(67.7966616690478,8.94305585212277,44.9537745060253));
#163526=CARTESIAN_POINT('Ctrl Pts',(67.3103740039708,8.76714068293004,45.0498483601642));
#163527=CARTESIAN_POINT('Ctrl Pts',(67.189122272089,8.72030120849037,45.0738654206605));
#163528=CARTESIAN_POINT('Ctrl Pts',(66.9803751612613,8.63445348628344,45.1153309446797));
#163529=CARTESIAN_POINT('Ctrl Pts',(66.892422396613,8.59664239913894,45.1328388876741));
#163530=CARTESIAN_POINT('Ctrl Pts',(66.7089068362032,8.51428014031234,45.1694500875882));
#163531=CARTESIAN_POINT('Ctrl Pts',(66.6134853209868,8.46943998561442,45.1885333538665));
#163532=CARTESIAN_POINT('Ctrl Pts',(66.3493299383934,8.33964170265897,45.2414932109064));
#163533=CARTESIAN_POINT('Ctrl Pts',(66.1823935944975,8.251045200325,45.275115282189));
#163534=CARTESIAN_POINT('Ctrl Pts',(65.7911919742105,8.0275298152719,45.3542508626446));
#163535=CARTESIAN_POINT('Ctrl Pts',(65.5696807032507,7.88798083492555,45.3993438335201));
#163536=CARTESIAN_POINT('Ctrl Pts',(64.976803850965,7.47784657526231,45.5206332480599));
#163537=CARTESIAN_POINT('Ctrl Pts',(64.6190340744635,7.18828988392634,45.5945320135782));
#163538=CARTESIAN_POINT('Ctrl Pts',(64.2226218741965,6.81508024424111,45.6764211767408));
#163539=CARTESIAN_POINT('Ctrl Pts',(64.1621396049242,6.75655917078396,45.6889145848829));
#163540=CARTESIAN_POINT('Ctrl Pts',(64.0631214673264,6.65810068743555,45.7093572118277));
#163541=CARTESIAN_POINT('Ctrl Pts',(64.0241408132752,6.61863759275749,45.7174018046744));
#163542=CARTESIAN_POINT('Ctrl Pts',(63.939531422534,6.53142857852746,45.7348538897822));
#163543=CARTESIAN_POINT('Ctrl Pts',(63.8940511714908,6.48353773236676,45.7442297823508));
#163544=CARTESIAN_POINT('Ctrl Pts',(63.7502170122502,6.32880210927485,45.7738757079306));
#163545=CARTESIAN_POINT('Ctrl Pts',(63.6538196743931,6.22009088945213,45.7937354689004));
#163546=CARTESIAN_POINT('Ctrl Pts',(63.4096578329589,5.93136086736737,45.8441023521848));
#163547=CARTESIAN_POINT('Ctrl Pts',(63.2659691884263,5.7478940184156,45.8738099494438));
#163548=CARTESIAN_POINT('Ctrl Pts',(62.837675918919,5.15655031671898,45.9629637280234));
#163549=CARTESIAN_POINT('Ctrl Pts',(62.5784233733331,4.73074206580403,46.0178922203095));
#163550=CARTESIAN_POINT('Ctrl Pts',(62.2931000338066,4.16476561179506,46.0807232472096));
#163551=CARTESIAN_POINT('Ctrl Pts',(62.2347087060269,4.04239654377244,46.0937380033867));
#163552=CARTESIAN_POINT('Ctrl Pts',(62.1389527001908,3.82997412969038,46.1153750919193));
#163553=CARTESIAN_POINT('Ctrl Pts',(62.1003054492743,3.74054447543286,46.1242003069603));
#163554=CARTESIAN_POINT('Ctrl Pts',(62.0228219007994,3.55328578285513,46.1420966381629));
#163555=CARTESIAN_POINT('Ctrl Pts',(61.9842226698562,3.45536996933814,46.1511298133378));
#163556=CARTESIAN_POINT('Ctrl Pts',(61.8837789958078,3.18745141400362,46.17497258347));
#163557=CARTESIAN_POINT('Ctrl Pts',(61.8251712753624,3.01623906647071,46.1892669265274));
#163558=CARTESIAN_POINT('Ctrl Pts',(61.7014705938649,2.61769704019826,46.2203811378928));
#163559=CARTESIAN_POINT('Ctrl Pts',(61.6399158951708,2.38935480918901,46.2366272675377));
#163560=CARTESIAN_POINT('Ctrl Pts',(61.5134742138492,1.83876015535367,46.271976884671));
#163561=CARTESIAN_POINT('Ctrl Pts',(61.4566789542818,1.514882355785,46.2897162252043));
#163562=CARTESIAN_POINT('Ctrl Pts',(61.3829730502265,0.911817358754139,
46.3167968886324));
#163563=CARTESIAN_POINT('Ctrl Pts',(61.3613509727544,0.633609519968516,
46.3269885572506));
#163564=CARTESIAN_POINT('Ctrl Pts',(61.3493294788365,0.27644775799563,46.3369130930585));
#163565=CARTESIAN_POINT('Ctrl Pts',(61.3476591515173,0.198075737816354,
46.3388963092262));
#163566=CARTESIAN_POINT('Ctrl Pts',(61.3465964072363,0.0797938840208599,
46.3415892699295));
#163567=CARTESIAN_POINT('Ctrl Pts',(61.3464881809499,0.0398973309146011,
46.3424460898535));
#163568=CARTESIAN_POINT('Ctrl Pts',(61.3466300729431,6.78351894061817E-10,
46.3432507993512));
#163569=CARTESIAN_POINT('Origin',(69.6316151486327,0.,39.48523201752));
#163570=CARTESIAN_POINT('',(61.5844733749945,-1.05941772399783E-11,47.6921271941932));
#163571=CARTESIAN_POINT('',(61.5550078861458,-4.86126027327237E-15,47.5250201029796));
#163572=CARTESIAN_POINT('',(60.4236626579685,-1.14504475720278E-15,41.1088424787055));
#163573=CARTESIAN_POINT('Ctrl Pts',(61.5844733749945,-2.11872094351994E-11,
47.6921271941932));
#163574=CARTESIAN_POINT('Ctrl Pts',(61.5842929354516,0.0507361671291354,
47.6911038706948));
#163575=CARTESIAN_POINT('Ctrl Pts',(61.5845214100859,0.101471586690972,
47.6900214356351));
#163576=CARTESIAN_POINT('Ctrl Pts',(61.5862815682886,0.241622984157713,
47.6868639103638));
#163577=CARTESIAN_POINT('Ctrl Pts',(61.5886742245124,0.331019890792252,
47.6846615324012));
#163578=CARTESIAN_POINT('Ctrl Pts',(61.6102159788509,0.85684770224775,47.6705525309141));
#163579=CARTESIAN_POINT('Ctrl Pts',(61.6583199084181,1.29142584940214,47.6541862392567));
#163580=CARTESIAN_POINT('Ctrl Pts',(61.7935917959083,2.03778638130491,47.6165165916725));
#163581=CARTESIAN_POINT('Ctrl Pts',(61.8671215260744,2.35138758969453,47.5976618126942));
#163582=CARTESIAN_POINT('Ctrl Pts',(62.0174597539692,2.87172645419634,47.5608806841529));
#163583=CARTESIAN_POINT('Ctrl Pts',(62.0858229563173,3.08071752135588,47.5445616599601));
#163584=CARTESIAN_POINT('Ctrl Pts',(62.1998241824614,3.39204170854816,47.5178368445746));
#163585=CARTESIAN_POINT('Ctrl Pts',(62.2401288325453,3.49633215786767,47.5084646823107));
#163586=CARTESIAN_POINT('Ctrl Pts',(62.3184627761913,3.68878201727469,47.4903798030388));
#163587=CARTESIAN_POINT('Ctrl Pts',(62.356007213887,3.77713137804031,47.4817614760077));
#163588=CARTESIAN_POINT('Ctrl Pts',(62.444551137137,3.97695331086373,47.4615434050977));
#163589=CARTESIAN_POINT('Ctrl Pts',(62.4963847322258,4.08802022114772,47.449781842913));
#163590=CARTESIAN_POINT('Ctrl Pts',(62.6781413189272,4.45841396233786,47.4087812380242));
#163591=CARTESIAN_POINT('Ctrl Pts',(62.8178094412927,4.7125578435906,47.3776562799437));
#163592=CARTESIAN_POINT('Ctrl Pts',(63.1814521335152,5.30709796324024,47.2976155258387));
#163593=CARTESIAN_POINT('Ctrl Pts',(63.4162224372565,5.63991142013717,47.2466884074534));
#163594=CARTESIAN_POINT('Ctrl Pts',(63.7568268631208,6.06105615200825,47.1742663267379));
#163595=CARTESIAN_POINT('Ctrl Pts',(63.8441382676801,6.16430264500433,47.1558152865586));
#163596=CARTESIAN_POINT('Ctrl Pts',(64.0009468622567,6.34168388079855,47.1229094958199));
#163597=CARTESIAN_POINT('Ctrl Pts',(64.0694756202341,6.41667133055997,47.1086019253659));
#163598=CARTESIAN_POINT('Ctrl Pts',(64.1793136706874,6.5329421853728,47.085798292829));
#163599=CARTESIAN_POINT('Ctrl Pts',(64.2198116851775,6.57500349641795,47.077416987984));
#163600=CARTESIAN_POINT('Ctrl Pts',(64.3028181220067,6.65958816724649,47.0602956712981));
#163601=CARTESIAN_POINT('Ctrl Pts',(64.3453482814871,6.70208543016566,47.0515527011133));
#163602=CARTESIAN_POINT('Ctrl Pts',(64.4673556420151,6.8216316254395,47.0265472894332));
#163603=CARTESIAN_POINT('Ctrl Pts',(64.5477973183034,6.89765283215523,47.010150283614));
#163604=CARTESIAN_POINT('Ctrl Pts',(65.038805601335,7.34518011827836,46.9105005960701));
#163605=CARTESIAN_POINT('Ctrl Pts',(65.480353797727,7.67993856850869,46.8226152984355));
#163606=CARTESIAN_POINT('Ctrl Pts',(66.1782498101072,8.11583051850937,46.6838542653863));
#163607=CARTESIAN_POINT('Ctrl Pts',(66.4139413240052,8.24885968766421,46.637026598617));
#163608=CARTESIAN_POINT('Ctrl Pts',(66.7593094615069,8.42401882617389,46.5683158940448));
#163609=CARTESIAN_POINT('Ctrl Pts',(66.864576240933,8.47488116457744,46.5473621037125));
#163610=CARTESIAN_POINT('Ctrl Pts',(67.0567483309537,8.5632067491331,46.5090814865076));
#163611=CARTESIAN_POINT('Ctrl Pts',(67.1433258714238,8.60137306869108,46.4918252635365));
#163612=CARTESIAN_POINT('Ctrl Pts',(67.335217076235,8.68240881958609,46.453553522453));
#163613=CARTESIAN_POINT('Ctrl Pts',(67.4407632375819,8.72466204937684,46.4324865824092));
#163614=CARTESIAN_POINT('Ctrl Pts',(67.7705233291266,8.84953419786848,46.3666146255636));
#163615=CARTESIAN_POINT('Ctrl Pts',(67.9971346922067,8.92524244646938,46.3212712850732));
#163616=CARTESIAN_POINT('Ctrl Pts',(68.676376836835,9.12264318304177,46.1852021866924));
#163617=CARTESIAN_POINT('Ctrl Pts',(69.1354991681207,9.21811255635417,46.0929954260109));
#163618=CARTESIAN_POINT('Ctrl Pts',(69.8655301277863,9.31138704599842,45.9469092282523));
#163619=CARTESIAN_POINT('Ctrl Pts',(70.132612834611,9.33345516464316,45.8935821136841));
#163620=CARTESIAN_POINT('Ctrl Pts',(70.4758986537097,9.34643310642858,45.82541276935));
#163621=CARTESIAN_POINT('Ctrl Pts',(70.5515222348317,9.34833764530241,45.8104188944733));
#163622=CARTESIAN_POINT('Ctrl Pts',(70.6778712594269,9.34992615942374,45.7854141189114));
#163623=CARTESIAN_POINT('Ctrl Pts',(70.7285837967516,9.35013517765976,45.7753906226654));
#163624=CARTESIAN_POINT('Ctrl Pts',(70.8383720794793,9.34965998121752,45.7537198955298));
#163625=CARTESIAN_POINT('Ctrl Pts',(70.8974450038083,9.34882288301324,45.7420774678941));
#163626=CARTESIAN_POINT('Ctrl Pts',(71.0768185555494,9.34451524391306,45.7067718257637));
#163627=CARTESIAN_POINT('Ctrl Pts',(71.1970727952368,9.33921447984585,45.6831656991541));
#163628=CARTESIAN_POINT('Ctrl Pts',(71.767970359901,9.30257568808484,45.5713006567979));
#163629=CARTESIAN_POINT('Ctrl Pts',(72.2161360986599,9.23978067162353,45.4840601309465));
#163630=CARTESIAN_POINT('Ctrl Pts',(72.9222270747495,9.08609362766255,45.3461211097089));
#163631=CARTESIAN_POINT('Ctrl Pts',(73.1839193302501,9.01669093156669,45.2948927267057));
#163632=CARTESIAN_POINT('Ctrl Pts',(73.6298976479552,8.87670134239577,45.2071950939817));
#163633=CARTESIAN_POINT('Ctrl Pts',(73.8156851763723,8.81165312246985,45.1705406976543));
#163634=CARTESIAN_POINT('Ctrl Pts',(74.099093148297,8.70192459788366,45.1143957831611));
#163635=CARTESIAN_POINT('Ctrl Pts',(74.1982541374931,8.66149560352107,45.0947069027952));
#163636=CARTESIAN_POINT('Ctrl Pts',(74.384281915816,8.58177533992011,45.057681322667));
#163637=CARTESIAN_POINT('Ctrl Pts',(74.4712880488393,8.54285445653339,45.0403267762469));
#163638=CARTESIAN_POINT('Ctrl Pts',(74.670434769791,8.44997414328666,45.0005158898019));
#163639=CARTESIAN_POINT('Ctrl Pts',(74.7821214252236,8.39505992903263,44.9781230320513));
#163640=CARTESIAN_POINT('Ctrl Pts',(75.2318753210742,8.16232396663947,44.8876825574029));
#163641=CARTESIAN_POINT('Ctrl Pts',(75.5599254332986,7.96544299901811,44.8210757649213));
#163642=CARTESIAN_POINT('Ctrl Pts',(76.1928779475659,7.52926816358422,44.6916148293074));
#163643=CARTESIAN_POINT('Ctrl Pts',(76.4969206679319,7.29002776986537,44.6289298468552));
#163644=CARTESIAN_POINT('Ctrl Pts',(76.8817031613893,6.94587147966392,44.5494635255703));
#163645=CARTESIAN_POINT('Ctrl Pts',(76.9762657471438,6.85764477573636,44.5299239699813));
#163646=CARTESIAN_POINT('Ctrl Pts',(77.1144611468848,6.72317323209954,44.5013830758345));
#163647=CARTESIAN_POINT('Ctrl Pts',(77.1594890109749,6.67844761848896,44.4920860919943));
#163648=CARTESIAN_POINT('Ctrl Pts',(77.2431542199366,6.59361772457472,44.4748209491069));
#163649=CARTESIAN_POINT('Ctrl Pts',(77.2818941931828,6.55362401444824,44.466830915629));
#163650=CARTESIAN_POINT('Ctrl Pts',(77.3818783572235,6.44852548867097,44.4462163758196));
#163651=CARTESIAN_POINT('Ctrl Pts',(77.4425576895692,6.38286767609957,44.4337122999456));
#163652=CARTESIAN_POINT('Ctrl Pts',(77.8257500122904,5.95601876208129,44.3547395037467));
#163653=CARTESIAN_POINT('Ctrl Pts',(78.1210224477279,5.57038294798842,44.2938098916412));
#163654=CARTESIAN_POINT('Ctrl Pts',(78.5184935178876,4.95741988162425,44.2100538041697));
#163655=CARTESIAN_POINT('Ctrl Pts',(78.6437057411616,4.74658094648005,44.1833469048989));
#163656=CARTESIAN_POINT('Ctrl Pts',(78.8473550659568,4.37070517350294,44.1391564574824));
#163657=CARTESIAN_POINT('Ctrl Pts',(78.9294991055963,4.20790417673299,44.1210767392552));
#163658=CARTESIAN_POINT('Ctrl Pts',(79.0514882243411,3.94747999309863,44.0937652729814));
#163659=CARTESIAN_POINT('Ctrl Pts',(79.0945127446425,3.85145197166169,44.0840294915981));
#163660=CARTESIAN_POINT('Ctrl Pts',(79.1742485775417,3.66513946355785,44.065775094472));
#163661=CARTESIAN_POINT('Ctrl Pts',(79.2111864757117,3.57497047303852,44.057220953098));
#163662=CARTESIAN_POINT('Ctrl Pts',(79.296062755395,3.35821358200969,44.0373202781904));
#163663=CARTESIAN_POINT('Ctrl Pts',(79.3426874747542,3.23111618883632,44.0261826816205));
#163664=CARTESIAN_POINT('Ctrl Pts',(79.6095671584164,2.45193874627957,43.961108463404));
#163665=CARTESIAN_POINT('Ctrl Pts',(79.7606548515972,1.77750193020893,43.9181130146766));
#163666=CARTESIAN_POINT('Ctrl Pts',(79.8565048939638,0.920491744571245,
43.8812914383959));
#163667=CARTESIAN_POINT('Ctrl Pts',(79.8710149393486,0.74838401433794,43.874785802587));
#163668=CARTESIAN_POINT('Ctrl Pts',(79.887660711033,0.456103357784508,43.8653100264595));
#163669=CARTESIAN_POINT('Ctrl Pts',(79.8922193259913,0.336127208478359,
43.8618677605506));
#163670=CARTESIAN_POINT('Ctrl Pts',(79.8956518364819,0.15635675704603,43.8574025493286));
#163671=CARTESIAN_POINT('Ctrl Pts',(79.896231078801,0.096615854261143,43.8560331407062));
#163672=CARTESIAN_POINT('Ctrl Pts',(79.8962652386196,-0.0149516582472375,
43.8536932349455));
#163673=CARTESIAN_POINT('Ctrl Pts',(79.8958591318493,-0.0667746651457365,
43.8526943805451));
#163674=CARTESIAN_POINT('Ctrl Pts',(79.893783252201,-0.196651454328757,
43.8504088285477));
#163675=CARTESIAN_POINT('Ctrl Pts',(79.8915777443699,-0.274694678543371,
43.8492322904412));
#163676=CARTESIAN_POINT('Ctrl Pts',(79.8774419494162,-0.623239351866993,
43.8448341465956));
#163677=CARTESIAN_POINT('Ctrl Pts',(79.8549509216157,-0.89320715823354,
43.8437310256787));
#163678=CARTESIAN_POINT('Ctrl Pts',(79.761097665114,-1.63513072707011,43.8465248467742));
#163679=CARTESIAN_POINT('Ctrl Pts',(79.6656921721349,-2.10318679714962,
43.8548386650293));
#163680=CARTESIAN_POINT('Ctrl Pts',(79.4698227408968,-2.79306192592099,
43.8758904798355));
#163681=CARTESIAN_POINT('Ctrl Pts',(79.3954270375592,-3.02157658766399,
43.8843862338626));
#163682=CARTESIAN_POINT('Ctrl Pts',(79.272154048444,-3.35627805357526,43.8990393336369));
#163683=CARTESIAN_POINT('Ctrl Pts',(79.2298742603108,-3.46483316014934,
43.9041472701406));
#163684=CARTESIAN_POINT('Ctrl Pts',(79.1490896085262,-3.66140620489206,
43.9140443140295));
#163685=CARTESIAN_POINT('Ctrl Pts',(79.111227501466,-3.74967598103152,43.9187317340391));
#163686=CARTESIAN_POINT('Ctrl Pts',(79.0240451250798,-3.94464965997893,
43.9296282729007));
#163687=CARTESIAN_POINT('Ctrl Pts',(78.9740660983701,-4.0510352142974,43.9359419926541));
#163688=CARTESIAN_POINT('Ctrl Pts',(78.8050064488066,-4.39406661237065,
43.9575099080971));
#163689=CARTESIAN_POINT('Ctrl Pts',(78.6779615505193,-4.62656135263761,
43.9740314033395));
#163690=CARTESIAN_POINT('Ctrl Pts',(78.280674488259,-5.28586991543662,44.0266620854071));
#163691=CARTESIAN_POINT('Ctrl Pts',(77.9857871601714,-5.69639426449568,
44.0668163399807));
#163692=CARTESIAN_POINT('Ctrl Pts',(77.5627833194022,-6.1951079653315,44.1266840464022));
#163693=CARTESIAN_POINT('Ctrl Pts',(77.4631596187382,-6.30700885685074,
44.140927466147));
#163694=CARTESIAN_POINT('Ctrl Pts',(77.3134842806087,-6.46722609250427,
44.1625752464041));
#163695=CARTESIAN_POINT('Ctrl Pts',(77.2654789458563,-6.51747918687255,
44.1695539992147));
#163696=CARTESIAN_POINT('Ctrl Pts',(77.1783702675988,-6.60665771758114,
44.1822864075788));
#163697=CARTESIAN_POINT('Ctrl Pts',(77.1394712133046,-6.64578300526042,
44.1879966853377));
#163698=CARTESIAN_POINT('Ctrl Pts',(77.0438098225237,-6.74031347790275,
44.2020968268391));
#163699=CARTESIAN_POINT('Ctrl Pts',(76.9866903220004,-6.79533882719089,
44.2105635522342));
#163700=CARTESIAN_POINT('Ctrl Pts',(76.7254401133325,-7.04067165445713,
44.2494749222281));
#163701=CARTESIAN_POINT('Ctrl Pts',(76.5136668174149,-7.22237105706044,
44.2815196386154));
#163702=CARTESIAN_POINT('Ctrl Pts',(75.8289899135573,-7.75825424614105,
44.3859355422191));
#163703=CARTESIAN_POINT('Ctrl Pts',(75.3306830973099,-8.07662238378006,
44.4629789001512));
#163704=CARTESIAN_POINT('Ctrl Pts',(74.6960227910028,-8.40105268266193,
44.5606599973577));
#163705=CARTESIAN_POINT('Ctrl Pts',(74.5851387575322,-8.45495128724056,
44.5777151784796));
#163706=CARTESIAN_POINT('Ctrl Pts',(74.3862930427995,-8.54670845206675,
44.6082706204161));
#163707=CARTESIAN_POINT('Ctrl Pts',(74.2987530858974,-8.58545587667913,
44.6217125886091));
#163708=CARTESIAN_POINT('Ctrl Pts',(74.1103622594536,-8.66534407638271,
44.6506164593381));
#163709=CARTESIAN_POINT('Ctrl Pts',(74.0093553248903,-8.7060717758318,44.6660989899191));
#163710=CARTESIAN_POINT('Ctrl Pts',(73.7163971595207,-8.81817812154903,
44.7109606166623));
#163711=CARTESIAN_POINT('Ctrl Pts',(73.5227793895229,-8.88492893541359,
44.7405556616244));
#163712=CARTESIAN_POINT('Ctrl Pts',(73.0526074671429,-9.02959950313031,
44.81231780172));
#163713=CARTESIAN_POINT('Ctrl Pts',(72.7743366292329,-9.10109686795152,
44.854702161811));
#163714=CARTESIAN_POINT('Ctrl Pts',(72.0100883376822,-9.25958522729923,
44.9711176202923));
#163715=CARTESIAN_POINT('Ctrl Pts',(71.5197864970839,-9.32052525431402,
45.0457882796291));
#163716=CARTESIAN_POINT('Ctrl Pts',(70.9431077636185,-9.34522877390416,
45.134663802177));
#163717=CARTESIAN_POINT('Ctrl Pts',(70.8589985663068,-9.34766867069676,
45.1476535652867));
#163718=CARTESIAN_POINT('Ctrl Pts',(70.7276352543985,-9.34966392969701,
45.1679927970317));
#163719=CARTESIAN_POINT('Ctrl Pts',(70.6803939688228,-9.35001496894424,
45.1753176745899));
#163720=CARTESIAN_POINT('Ctrl Pts',(70.5786665679482,-9.34998168171136,
45.1911155105324));
#163721=CARTESIAN_POINT('Ctrl Pts',(70.5241828871197,-9.34947628301745,
45.1995918244727));
#163722=CARTESIAN_POINT('Ctrl Pts',(70.3749020693892,-9.34675527259986,
45.2228526695562));
#163723=CARTESIAN_POINT('Ctrl Pts',(70.2801333916433,-9.34355063555204,
45.2376597266483));
#163724=CARTESIAN_POINT('Ctrl Pts',(69.8494099039252,-9.32226378291602,
45.3050960059052));
#163725=CARTESIAN_POINT('Ctrl Pts',(69.5145911943086,-9.28709552336704,
45.3578927054202));
#163726=CARTESIAN_POINT('Ctrl Pts',(68.6486251493079,-9.14743292108761,
45.4944157637464));
#163727=CARTESIAN_POINT('Ctrl Pts',(68.1233207982288,-9.01408871639936,
45.5771534099938));
#163728=CARTESIAN_POINT('Ctrl Pts',(67.4793680043824,-8.78841095541494,
45.6772353876486));
#163729=CARTESIAN_POINT('Ctrl Pts',(67.3474153734026,-8.73872747713203,
45.6976735660068));
#163730=CARTESIAN_POINT('Ctrl Pts',(67.1268032895602,-8.64981397540812,
45.7317133640528));
#163731=CARTESIAN_POINT('Ctrl Pts',(67.0375442484723,-8.61219032828018,
45.7454489470292));
#163732=CARTESIAN_POINT('Ctrl Pts',(66.8552747594323,-8.5319498712965,45.773418770139));
#163733=CARTESIAN_POINT('Ctrl Pts',(66.7623449495561,-8.4891772279756,45.7876362163649));
#163734=CARTESIAN_POINT('Ctrl Pts',(66.5189155672574,-8.3721832832526,45.8247640727464));
#163735=CARTESIAN_POINT('Ctrl Pts',(66.3696644570503,-8.29537015094108,
45.8474096647137));
#163736=CARTESIAN_POINT('Ctrl Pts',(66.1217267607052,-8.15909004759748,
45.8848372409637));
#163737=CARTESIAN_POINT('Ctrl Pts',(66.0219336368077,-8.10178570775886,
45.8998476125375));
#163738=CARTESIAN_POINT('Ctrl Pts',(65.5790041948646,-7.83632365892998,
45.9662455043399));
#163739=CARTESIAN_POINT('Ctrl Pts',(65.2482939337322,-7.6076674799902,46.015184367765));
#163740=CARTESIAN_POINT('Ctrl Pts',(64.7316571227747,-7.19842344716327,
46.0911276093541));
#163741=CARTESIAN_POINT('Ctrl Pts',(64.5367085343107,-7.03036358650403,
46.1196564078289));
#163742=CARTESIAN_POINT('Ctrl Pts',(64.2902792969943,-6.79939483554443,
46.155731584172));
#163743=CARTESIAN_POINT('Ctrl Pts',(64.2323534000645,-6.74367418913392,
46.1642126727656));
#163744=CARTESIAN_POINT('Ctrl Pts',(64.1358246750655,-6.6483781690436,46.1783561062047));
#163745=CARTESIAN_POINT('Ctrl Pts',(64.0968427633549,-6.60920138930952,
46.1840710023907));
#163746=CARTESIAN_POINT('Ctrl Pts',(64.0101334607199,-6.52048995157325,
46.1967916718428));
#163747=CARTESIAN_POINT('Ctrl Pts',(63.9626003298457,-6.4707673840282,46.2037702714994));
#163748=CARTESIAN_POINT('Ctrl Pts',(63.8046276084255,-6.30180719229914,
46.2269685667879));
#163749=CARTESIAN_POINT('Ctrl Pts',(63.6967354426032,-6.18017931554389,
46.2428214013686));
#163750=CARTESIAN_POINT('Ctrl Pts',(63.4106532575059,-5.84018228267994,
46.2847550609032));
#163751=CARTESIAN_POINT('Ctrl Pts',(63.2390201432225,-5.61639797040577,
46.3097955129248));
#163752=CARTESIAN_POINT('Ctrl Pts',(62.8392886966675,-5.04347252996542,
46.3673001421793));
#163753=CARTESIAN_POINT('Ctrl Pts',(62.623753983855,-4.68609939844356,46.3975289029817));
#163754=CARTESIAN_POINT('Ctrl Pts',(62.3678260815757,-4.19025164771539,
46.4316938538536));
#163755=CARTESIAN_POINT('Ctrl Pts',(62.3060310686472,-4.06366583368732,
46.4397797356504));
#163756=CARTESIAN_POINT('Ctrl Pts',(62.2062994777375,-3.8472439589025,46.4525258896893));
#163757=CARTESIAN_POINT('Ctrl Pts',(62.1668896177593,-3.75813053523251,
46.457472739046));
#163758=CARTESIAN_POINT('Ctrl Pts',(62.0884000553372,-3.57298223156225,
46.4671294501713));
#163759=CARTESIAN_POINT('Ctrl Pts',(62.0495067118821,-3.47688095411806,
46.471803467681));
#163760=CARTESIAN_POINT('Ctrl Pts',(61.9506771143066,-3.22068420441144,
46.4833718946316));
#163761=CARTESIAN_POINT('Ctrl Pts',(61.8934706957066,-3.05955440991123,
46.4897377913923));
#163762=CARTESIAN_POINT('Ctrl Pts',(61.7456597363704,-2.60461511553207,
46.505201460731));
#163763=CARTESIAN_POINT('Ctrl Pts',(61.6649033228772,-2.30777256955171,
46.5124132896182));
#163764=CARTESIAN_POINT('Ctrl Pts',(61.483313556705,-1.48442652282495,46.5248916239801));
#163765=CARTESIAN_POINT('Ctrl Pts',(61.4123666256894,-0.95244722013598,
46.5246862459331));
#163766=CARTESIAN_POINT('Ctrl Pts',(61.3825629698841,-0.328599288406227,
46.5162097791634));
#163767=CARTESIAN_POINT('Ctrl Pts',(61.3795722237579,-0.239723111787004,
46.5148100865087));
#163768=CARTESIAN_POINT('Ctrl Pts',(61.3768903644626,-0.102378217551117,
46.512360485323));
#163769=CARTESIAN_POINT('Ctrl Pts',(61.3763170637519,-0.0539295302680966,
46.5114413258576));
#163770=CARTESIAN_POINT('Ctrl Pts',(61.3761090838066,-0.00365311208907833,
46.5104314954195));
#163771=CARTESIAN_POINT('Ctrl Pts',(61.3761020578081,-0.00182655558397092,
46.5103947313045));
#163772=CARTESIAN_POINT('Ctrl Pts',(61.3760955617941,-4.66200292569332E-12,
46.5103578905782));
#163773=CARTESIAN_POINT('',(61.5550077244638,4.54923683265615E-5,47.5250191853983));
#163774=CARTESIAN_POINT('Ctrl Pts',(61.3466300729431,6.78351894061817E-10,
46.3432507993512));
#163775=CARTESIAN_POINT('Ctrl Pts',(61.3466726607641,-0.0119748847392668,
46.3434923268914));
#163776=CARTESIAN_POINT('Ctrl Pts',(61.3467377807059,-0.0239498401668987,
46.3437291599298));
#163777=CARTESIAN_POINT('Ctrl Pts',(61.3472616663556,-0.0955194346373169,
46.3451166672421));
#163778=CARTESIAN_POINT('Ctrl Pts',(61.348256014986,-0.155110844989952,
46.3461561349238));
#163779=CARTESIAN_POINT('Ctrl Pts',(61.3529156344919,-0.333901531499684,
46.3489343308675));
#163780=CARTESIAN_POINT('Ctrl Pts',(61.3582576403879,-0.453050007964962,
46.3503314868498));
#163781=CARTESIAN_POINT('Ctrl Pts',(61.3767024539108,-0.742763072692121,
46.3526667192506));
#163782=CARTESIAN_POINT('Ctrl Pts',(61.3921642298094,-0.913137614746343,
46.3531419890592));
#163783=CARTESIAN_POINT('Ctrl Pts',(61.4484768670439,-1.3902732856939,46.352084861717));
#163784=CARTESIAN_POINT('Ctrl Pts',(61.4997137632451,-1.69557791631918,
46.3486227128504));
#163785=CARTESIAN_POINT('Ctrl Pts',(61.6495225018596,-2.38089696814083,
46.335037561194));
#163786=CARTESIAN_POINT('Ctrl Pts',(61.7569452993122,-2.75834853336005,
46.3234020627189));
#163787=CARTESIAN_POINT('Ctrl Pts',(61.9314304590403,-3.25241660548061,
46.302932504685));
#163788=CARTESIAN_POINT('Ctrl Pts',(61.9780020879817,-3.37597157857149,
46.2973572918494));
#163789=CARTESIAN_POINT('Ctrl Pts',(62.0633337041784,-3.58871941622418,
46.2869682484681));
#163790=CARTESIAN_POINT('Ctrl Pts',(62.1009120258662,-3.67837269398528,
46.2823416237566));
#163791=CARTESIAN_POINT('Ctrl Pts',(62.1827555074008,-3.86546421015422,
46.2721630696317));
#163792=CARTESIAN_POINT('Ctrl Pts',(62.2273065483308,-3.96275963774058,
46.2665656605729));
#163793=CARTESIAN_POINT('Ctrl Pts',(62.3562627005691,-4.23216841650119,
46.2502111220432));
#163794=CARTESIAN_POINT('Ctrl Pts',(62.4442649437281,-4.4024655934303,46.2388822110638));
#163795=CARTESIAN_POINT('Ctrl Pts',(62.6662437506602,-4.80165151662173,
46.2099026801945));
#163796=CARTESIAN_POINT('Ctrl Pts',(62.8047986237087,-5.0277503326074,46.1915099439424));
#163797=CARTESIAN_POINT('Ctrl Pts',(63.2115943451449,-5.63261191214171,
46.1365293905606));
#163798=CARTESIAN_POINT('Ctrl Pts',(63.4985000435387,-5.99760905925112,
46.0967496198762));
#163799=CARTESIAN_POINT('Ctrl Pts',(63.8679447031853,-6.4020404625602,46.0435922621873));
#163800=CARTESIAN_POINT('Ctrl Pts',(63.9258665430216,-6.46374675374832,
46.0352070381961));
#163801=CARTESIAN_POINT('Ctrl Pts',(64.0233130511043,-6.56478071413928,
46.0210067611629));
#163802=CARTESIAN_POINT('Ctrl Pts',(64.0623741307016,-6.60456236937709,
46.0152903756185));
#163803=CARTESIAN_POINT('Ctrl Pts',(64.1487016008485,-6.69092522428066,
46.0026019156905));
#163804=CARTESIAN_POINT('Ctrl Pts',(64.1961101059915,-6.73735437443061,
45.9955993525748));
#163805=CARTESIAN_POINT('Ctrl Pts',(64.3493257147542,-6.88424065940277,
45.9728699872818));
#163806=CARTESIAN_POINT('Ctrl Pts',(64.4569630883872,-6.98269597000688,
45.9567550712773));
#163807=CARTESIAN_POINT('Ctrl Pts',(64.7428876245874,-7.23215576862245,
45.9136612401674));
#163808=CARTESIAN_POINT('Ctrl Pts',(64.9245675154636,-7.37899361112587,
45.8860030442394));
#163809=CARTESIAN_POINT('Ctrl Pts',(65.5091169965193,-7.81601653809011,
45.7965602056484));
#163810=CARTESIAN_POINT('Ctrl Pts',(65.9295686122815,-8.0805409665039,45.7316287471787));
#163811=CARTESIAN_POINT('Ctrl Pts',(66.4886148872436,-8.37221490034032,
45.6455639737845));
#163812=CARTESIAN_POINT('Ctrl Pts',(66.6096241865374,-8.43199967080375,
45.6269463126964));
#163813=CARTESIAN_POINT('Ctrl Pts',(66.8196716730826,-8.5300810250407,45.5946628630405));
#163814=CARTESIAN_POINT('Ctrl Pts',(66.9080909718603,-8.56967734571778,
45.5810829068597));
#163815=CARTESIAN_POINT('Ctrl Pts',(67.0932194860375,-8.64909079682306,
45.5526734096657));
#163816=CARTESIAN_POINT('Ctrl Pts',(67.1900145651305,-8.68866849190123,
45.5378325779662));
#163817=CARTESIAN_POINT('Ctrl Pts',(67.4548202028363,-8.79169711251207,
45.4972698836512));
#163818=CARTESIAN_POINT('Ctrl Pts',(67.6240300661649,-8.85187506142831,
45.4713919534327));
#163819=CARTESIAN_POINT('Ctrl Pts',(68.0178739928377,-8.97904413005395,
45.411243430795));
#163820=CARTESIAN_POINT('Ctrl Pts',(68.2435119467076,-9.04245827772779,
45.3768458854809));
#163821=CARTESIAN_POINT('Ctrl Pts',(68.7878083763292,-9.17313444876951,
45.2939221829229));
#163822=CARTESIAN_POINT('Ctrl Pts',(69.1080820201528,-9.23217904713312,
45.2451740618639));
#163823=CARTESIAN_POINT('Ctrl Pts',(69.7047365491124,-9.30957189379992,
45.1540607697768));
#163824=CARTESIAN_POINT('Ctrl Pts',(69.9801592643347,-9.33267595224281,
45.1118838544893));
#163825=CARTESIAN_POINT('Ctrl Pts',(70.3335571167051,-9.34624476590553,
45.0573821941967));
#163826=CARTESIAN_POINT('Ctrl Pts',(70.4110027406322,-9.3482324668144,45.0454145715436));
#163827=CARTESIAN_POINT('Ctrl Pts',(70.5397230860263,-9.34989846758445,
45.0254762742257));
#163828=CARTESIAN_POINT('Ctrl Pts',(70.5909894278427,-9.3501303981416,45.0175227362279));
#163829=CARTESIAN_POINT('Ctrl Pts',(70.7011646808674,-9.34970123745941,
45.0004008606364));
#163830=CARTESIAN_POINT('Ctrl Pts',(70.760069552404,-9.34890178716619,44.9912293524378));
#163831=CARTESIAN_POINT('Ctrl Pts',(70.9368317726177,-9.3447917071955,44.963662634205));
#163832=CARTESIAN_POINT('Ctrl Pts',(71.0546311473423,-9.33976834879518,
44.9452316739513));
#163833=CARTESIAN_POINT('Ctrl Pts',(71.3410872683884,-9.32198850567812,
44.9003128067773));
#163834=CARTESIAN_POINT('Ctrl Pts',(71.509548379318,-9.30682376647028,44.8738124606415));
#163835=CARTESIAN_POINT('Ctrl Pts',(71.9808747458421,-9.2511570394844,44.7995754990106));
#163836=CARTESIAN_POINT('Ctrl Pts',(72.2822915445319,-9.20011911921818,
44.7519962490739));
#163837=CARTESIAN_POINT('Ctrl Pts',(72.9591737565349,-9.05027084314983,
44.6454697094686));
#163838=CARTESIAN_POINT('Ctrl Pts',(73.3321201375491,-8.94246393286336,
44.5870148755854));
#163839=CARTESIAN_POINT('Ctrl Pts',(73.8204232690107,-8.76708205076489,
44.5112103276699));
#163840=CARTESIAN_POINT('Ctrl Pts',(73.9425517105278,-8.72024992377672,
44.4923124034965));
#163841=CARTESIAN_POINT('Ctrl Pts',(74.1528634767407,-8.63441076443044,
44.4598859799939));
#163842=CARTESIAN_POINT('Ctrl Pts',(74.2414965976929,-8.59659994050184,
44.4462570159857));
#163843=CARTESIAN_POINT('Ctrl Pts',(74.4264731097673,-8.5142322846033,44.4178933287952));
#163844=CARTESIAN_POINT('Ctrl Pts',(74.522676699809,-8.4693860110368,44.403188185328));
#163845=CARTESIAN_POINT('Ctrl Pts',(74.7890852228057,-8.33954852375368,
44.3625971097258));
#163846=CARTESIAN_POINT('Ctrl Pts',(74.9575122358945,-8.25091549104413,
44.337087163515));
#163847=CARTESIAN_POINT('Ctrl Pts',(75.3523738504045,-8.02727509853063,
44.2776238000474));
#163848=CARTESIAN_POINT('Ctrl Pts',(75.5760719862675,-7.88763001333651,
44.2442180599122));
#163849=CARTESIAN_POINT('Ctrl Pts',(76.1746076003093,-7.47746674754934,
44.1554285809942));
#163850=CARTESIAN_POINT('Ctrl Pts',(76.535905853825,-7.18801349112879,44.1025313295171));
#163851=CARTESIAN_POINT('Ctrl Pts',(76.936240287193,-6.81495285807577,44.0439271985903));
#163852=CARTESIAN_POINT('Ctrl Pts',(76.9973213463289,-6.75645523117442,
44.0349849077155));
#163853=CARTESIAN_POINT('Ctrl Pts',(77.0973299370408,-6.65802368003523,
44.0203328537811));
#163854=CARTESIAN_POINT('Ctrl Pts',(77.1367074432985,-6.61856342587494,
44.0145606720422));
#163855=CARTESIAN_POINT('Ctrl Pts',(77.2221916074237,-6.53134398961019,
44.0020209130758));
#163856=CARTESIAN_POINT('Ctrl Pts',(77.2681475924562,-6.48343955303723,
43.9952744732626));
#163857=CARTESIAN_POINT('Ctrl Pts',(77.4135366697861,-6.32860330746571,
43.9739251736349));
#163858=CARTESIAN_POINT('Ctrl Pts',(77.5109871153879,-6.21980159041315,
43.959606518489));
#163859=CARTESIAN_POINT('Ctrl Pts',(77.7579129448062,-5.93073296709067,
43.923389322992));
#163860=CARTESIAN_POINT('Ctrl Pts',(77.9032709278136,-5.7470067615247,43.9021357372137));
#163861=CARTESIAN_POINT('Ctrl Pts',(78.3359817498253,-5.15580834521874,
43.8394660783437));
#163862=CARTESIAN_POINT('Ctrl Pts',(78.5980570752674,-4.73047577709636,
43.8024604939837));
#163863=CARTESIAN_POINT('Ctrl Pts',(78.8874360059866,-4.16498448900198,
43.7639451975362));
#163864=CARTESIAN_POINT('Ctrl Pts',(78.9467778682253,-4.04258017942232,
43.7562011800701));
#163865=CARTESIAN_POINT('Ctrl Pts',(79.0441823778068,-3.83011726014096,
43.7437797386978));
#163866=CARTESIAN_POINT('Ctrl Pts',(79.0835210522288,-3.74068305111187,
43.7388540220899));
#163867=CARTESIAN_POINT('Ctrl Pts',(79.1624520231416,-3.55343393065613,
43.7291700137279));
#163868=CARTESIAN_POINT('Ctrl Pts',(79.2018091886896,-3.45553250299467,
43.7244570311495));
#163869=CARTESIAN_POINT('Ctrl Pts',(79.3043203981019,-3.18770752122583,
43.7125111929558));
#163870=CARTESIAN_POINT('Ctrl Pts',(79.3642607195549,-3.01657580170413,
43.7059004045354));
#163871=CARTESIAN_POINT('Ctrl Pts',(79.4910868677747,-2.61827390662252,
43.6928342408215));
#163872=CARTESIAN_POINT('Ctrl Pts',(79.5544587247302,-2.39009307307585,
43.6870485320038));
#163873=CARTESIAN_POINT('Ctrl Pts',(79.6853816149668,-1.83966854410041,
43.677013679843));
#163874=CARTESIAN_POINT('Ctrl Pts',(79.7448506469194,-1.51579562147201,
43.6742524479917));
#163875=CARTESIAN_POINT('Ctrl Pts',(79.8234791940555,-0.912379387627375,
43.6744812281231));
#163876=CARTESIAN_POINT('Ctrl Pts',(79.8473251561585,-0.633812339879392,
43.6766641937312));
#163877=CARTESIAN_POINT('Ctrl Pts',(79.8620238830965,-0.276314779159023,
43.681884424806));
#163878=CARTESIAN_POINT('Ctrl Pts',(79.8642700600739,-0.19796777031579,
43.6831764891021));
#163879=CARTESIAN_POINT('Ctrl Pts',(79.8663742280622,-0.0682497633545942,
43.6855532569837));
#163880=CARTESIAN_POINT('Ctrl Pts',(79.8667884538124,-0.0168900632655849,
43.6865557931488));
#163881=CARTESIAN_POINT('Ctrl Pts',(79.8667780725513,0.0938369406020547,
43.6888477114382));
#163882=CARTESIAN_POINT('Ctrl Pts',(79.866212708815,0.153200899447015,43.6901578905364));
#163883=CARTESIAN_POINT('Ctrl Pts',(79.8628528270007,0.330510398218484,
43.6943213851528));
#163884=CARTESIAN_POINT('Ctrl Pts',(79.8584087802861,0.448406855380347,
43.6974207258766));
#163885=CARTESIAN_POINT('Ctrl Pts',(79.8422744922485,0.734255331836819,
43.7057819316328));
#163886=CARTESIAN_POINT('Ctrl Pts',(79.828303006439,0.902026381114984,43.7114007504348));
#163887=CARTESIAN_POINT('Ctrl Pts',(79.7755870792911,1.38043930972032,43.7295972908011));
#163888=CARTESIAN_POINT('Ctrl Pts',(79.7259058096718,1.68957455777478,43.7439975619436));
#163889=CARTESIAN_POINT('Ctrl Pts',(79.5797051199031,2.37939279627776,43.7826895473336));
#163890=CARTESIAN_POINT('Ctrl Pts',(79.4746312691167,2.75756779437402,43.808535770282));
#163891=CARTESIAN_POINT('Ctrl Pts',(79.3034285819782,3.25234275460055,43.8490349265531));
#163892=CARTESIAN_POINT('Ctrl Pts',(79.2577553666244,3.37590974147408,43.8597252007661));
#163893=CARTESIAN_POINT('Ctrl Pts',(79.1740126928187,3.58867109811851,43.8791487803523));
#163894=CARTESIAN_POINT('Ctrl Pts',(79.1371181047329,3.67832604909296,43.8876537629297));
#163895=CARTESIAN_POINT('Ctrl Pts',(79.0567316031642,3.86541446290809,43.9060806342698));
#163896=CARTESIAN_POINT('Ctrl Pts',(79.0129557062284,3.96270521286113,43.9160575220774));
#163897=CARTESIAN_POINT('Ctrl Pts',(78.8862010040632,4.23208053550023,43.9447908598919));
#163898=CARTESIAN_POINT('Ctrl Pts',(78.7996480317851,4.40234977481434,43.9642399944474));
#163899=CARTESIAN_POINT('Ctrl Pts',(78.581202121744,4.80144705626461,44.0129167707692));
#163900=CARTESIAN_POINT('Ctrl Pts',(78.4447566902517,5.02748742971026,44.0430122573211));
#163901=CARTESIAN_POINT('Ctrl Pts',(78.0437031144844,5.63238183204341,44.1304776619868));
#163902=CARTESIAN_POINT('Ctrl Pts',(77.7604473021958,5.99745950068413,44.1912350519678));
#163903=CARTESIAN_POINT('Ctrl Pts',(77.3950336374395,6.40197581988324,44.2676555646764));
#163904=CARTESIAN_POINT('Ctrl Pts',(77.3377260177182,6.46369500267863,44.2795887881123));
#163905=CARTESIAN_POINT('Ctrl Pts',(77.241286860215,6.56474336759332,44.299576214983));
#163906=CARTESIAN_POINT('Ctrl Pts',(77.2026250052317,6.60452682870524,44.3075645356558));
#163907=CARTESIAN_POINT('Ctrl Pts',(77.1171689031824,6.69088563015779,44.3251660399807));
#163908=CARTESIAN_POINT('Ctrl Pts',(77.0702308398464,6.73730908233219,44.3347991582582));
#163909=CARTESIAN_POINT('Ctrl Pts',(76.9185285751454,6.88415200333873,44.3658337798556));
#163910=CARTESIAN_POINT('Ctrl Pts',(76.8119133828088,6.9825714618315,44.3874963293361));
#163911=CARTESIAN_POINT('Ctrl Pts',(76.5286522353668,7.2319044336687,44.4447614961987));
#163912=CARTESIAN_POINT('Ctrl Pts',(76.3485911559729,7.37865804067762,44.4808853429198));
#163913=CARTESIAN_POINT('Ctrl Pts',(75.7686351820489,7.815799767526,44.5967787128622));
#163914=CARTESIAN_POINT('Ctrl Pts',(75.351108782912,8.08048320056685,44.6796101264728));
#163915=CARTESIAN_POINT('Ctrl Pts',(74.7961135331527,8.37226645687446,44.789986101782));
#163916=CARTESIAN_POINT('Ctrl Pts',(74.6760508461963,8.4320412981402,44.8138755720144));
#163917=CARTESIAN_POINT('Ctrl Pts',(74.4676481176996,8.53011160846007,44.8553757657832));
#163918=CARTESIAN_POINT('Ctrl Pts',(74.379918666909,8.56970612874324,44.8728555433475));
#163919=CARTESIAN_POINT('Ctrl Pts',(74.1962336795464,8.64911987511433,44.9094779314105));
#163920=CARTESIAN_POINT('Ctrl Pts',(74.1001934752728,8.68869936729909,44.928639325752));
#163921=CARTESIAN_POINT('Ctrl Pts',(73.8374406052869,8.79174215847888,44.9811004715326));
#163922=CARTESIAN_POINT('Ctrl Pts',(73.669546913669,8.85193052735368,45.0146639044545));
#163923=CARTESIAN_POINT('Ctrl Pts',(73.2787705307102,8.97912627689817,45.0928678432809));
#163924=CARTESIAN_POINT('Ctrl Pts',(73.0549001899189,9.04255322668433,45.1377326031135));
#163925=CARTESIAN_POINT('Ctrl Pts',(72.5149878427279,9.17322117496631,45.245986137296));
#163926=CARTESIAN_POINT('Ctrl Pts',(72.1973539487951,9.23225042323679,45.3097183456386));
#163927=CARTESIAN_POINT('Ctrl Pts',(71.6056777244385,9.30959372118856,45.4281357791377));
#163928=CARTESIAN_POINT('Ctrl Pts',(71.332601583977,9.33267835252477,45.482670079045));
#163929=CARTESIAN_POINT('Ctrl Pts',(70.9820293622766,9.34624341394468,45.5522939643191));
#163930=CARTESIAN_POINT('Ctrl Pts',(70.9051522017376,9.34823171241028,45.567537818062));
#163931=CARTESIAN_POINT('Ctrl Pts',(70.7773650805505,9.34989826679501,45.5928289416275));
#163932=CARTESIAN_POINT('Ctrl Pts',(70.7264688613684,9.35013035922616,45.602889453219));
#163933=CARTESIAN_POINT('Ctrl Pts',(70.6170846369799,9.34970151916232,45.6244817905244));
#163934=CARTESIAN_POINT('Ctrl Pts',(70.5585993426785,9.34890232881752,45.6360092582636));
#163935=CARTESIAN_POINT('Ctrl Pts',(70.3830950720406,9.34479359661985,45.670556107415));
#163936=CARTESIAN_POINT('Ctrl Pts',(70.2661183186129,9.33977211512419,45.6935220909587));
#163937=CARTESIAN_POINT('Ctrl Pts',(69.9816432283738,9.3219998770592,45.7492725090466));
#163938=CARTESIAN_POINT('Ctrl Pts',(69.8143243141681,9.30684261005231,45.7819784001714));
#163939=CARTESIAN_POINT('Ctrl Pts',(69.3460036069198,9.25118542265482,45.8734271983071));
#163940=CARTESIAN_POINT('Ctrl Pts',(69.0464176982463,9.20013952992897,45.931822272195));
#163941=CARTESIAN_POINT('Ctrl Pts',(68.3738424006576,9.05027529716222,46.0632430078357));
#163942=CARTESIAN_POINT('Ctrl Pts',(68.0033873173336,8.94246677995383,46.1358700431178));
#163943=CARTESIAN_POINT('Ctrl Pts',(67.5185985652017,8.76708234335628,46.2316480011527));
#163944=CARTESIAN_POINT('Ctrl Pts',(67.3973717741238,8.72025017970903,46.2556601728448));
#163945=CARTESIAN_POINT('Ctrl Pts',(67.1886527286124,8.63441097764425,46.2971201899961));
#163946=CARTESIAN_POINT('Ctrl Pts',(67.100703441243,8.59660015240663,46.3146274691476));
#163947=CARTESIAN_POINT('Ctrl Pts',(66.917181457716,8.51423252345746,46.351240008046));
#163948=CARTESIAN_POINT('Ctrl Pts',(66.8217502474301,8.46938628043826,46.3703252489888));
#163949=CARTESIAN_POINT('Ctrl Pts',(66.5575255067944,8.33954898889645,46.4232991256447));
#163950=CARTESIAN_POINT('Ctrl Pts',(66.3905312605465,8.25091613858479,46.4569329894159));
#163951=CARTESIAN_POINT('Ctrl Pts',(65.9991459688741,8.02727637034531,46.5361061429746));
#163952=CARTESIAN_POINT('Ctrl Pts',(65.7775136528271,7.88763176513871,46.5812241582663));
#163953=CARTESIAN_POINT('Ctrl Pts',(65.1847060251401,7.47746865092028,46.7025006395234));
#163954=CARTESIAN_POINT('Ctrl Pts',(64.8271039639216,7.18801488609426,46.7763649342709));
#163955=CARTESIAN_POINT('Ctrl Pts',(64.4308679765701,6.81495351472009,46.8582176872529));
#163956=CARTESIAN_POINT('Ctrl Pts',(64.3704119763466,6.75645576698684,46.8707056632443));
#163957=CARTESIAN_POINT('Ctrl Pts',(64.2714231920131,6.65802407706972,46.891142220252));
#163958=CARTESIAN_POINT('Ctrl Pts',(64.232446218481,6.6185638082873,46.8991860479607));
#163959=CARTESIAN_POINT('Ctrl Pts',(64.1478285729352,6.53134442581497,46.9166398262734));
#163960=CARTESIAN_POINT('Ctrl Pts',(64.1023367147926,6.48344005934743,46.9260181067699));
#163961=CARTESIAN_POINT('Ctrl Pts',(63.9584142392529,6.32860433300367,46.9556822261476));
#163962=CARTESIAN_POINT('Ctrl Pts',(63.8619438848834,6.21980308296312,46.9755570289167));
#163963=CARTESIAN_POINT('Ctrl Pts',(63.6175238345535,5.9307362076723,47.0259773279547));
#163964=CARTESIAN_POINT('Ctrl Pts',(63.4736637457863,5.74701134127474,47.0557206629557));
#163965=CARTESIAN_POINT('Ctrl Pts',(63.0456130382846,5.15581217900249,47.1448265123596));
#163966=CARTESIAN_POINT('Ctrl Pts',(62.7866844550062,4.73047715963278,47.1996880252191));
#163967=CARTESIAN_POINT('Ctrl Pts',(62.5015830507618,4.1649833701103,47.2624691674286));
#163968=CARTESIAN_POINT('Ctrl Pts',(62.4431714350186,4.04257924072671,47.2754882612951));
#163969=CARTESIAN_POINT('Ctrl Pts',(62.3473928689251,3.83011652856883,47.2971302038777));
#163970=CARTESIAN_POINT('Ctrl Pts',(62.3087419315082,3.7406823428418,47.3059561595857));
#163971=CARTESIAN_POINT('Ctrl Pts',(62.231258951763,3.55343317352007,47.3238521521074));
#163972=CARTESIAN_POINT('Ctrl Pts',(62.1926633600608,3.45553167236604,47.3328843455987));
#163973=CARTESIAN_POINT('Ctrl Pts',(62.0922484679552,3.18770621258904,47.356719865362));
#163974=CARTESIAN_POINT('Ctrl Pts',(62.0336618589915,3.01657408119746,47.3710085824877));
#163975=CARTESIAN_POINT('Ctrl Pts',(61.9100150953728,2.6182709596395,47.4021075803621));
#163976=CARTESIAN_POINT('Ctrl Pts',(61.848486068248,2.39008930181531,47.4183452873219));
#163977=CARTESIAN_POINT('Ctrl Pts',(61.6798368110033,1.65602837583178,47.4654870472214));
#163978=CARTESIAN_POINT('Ctrl Pts',(61.6055753582875,1.14324940002398,47.4908841185973));
#163979=CARTESIAN_POINT('Ctrl Pts',(61.5658269000459,0.505351179248187,
47.512236036455));
#163980=CARTESIAN_POINT('Ctrl Pts',(61.5605908046069,0.383857980702777,
47.5158457141457));
#163981=CARTESIAN_POINT('Ctrl Pts',(61.5565217323495,0.213904894315144,
47.5202346860237));
#163982=CARTESIAN_POINT('Ctrl Pts',(61.555731712949,0.165514109940709,47.5214095668697));
#163983=CARTESIAN_POINT('Ctrl Pts',(61.5549698199378,0.0780956836856776,
47.523395001381));
#163984=CARTESIAN_POINT('Ctrl Pts',(61.5548691195383,0.0390708528840299,
47.524232024342));
#163985=CARTESIAN_POINT('Ctrl Pts',(61.5550077244638,4.54923683265615E-5,
47.5250191853983));
#163986=CARTESIAN_POINT('Ctrl Pts',(61.5550077244638,4.54923683265615E-5,
47.5250191853983));
#163987=CARTESIAN_POINT('Ctrl Pts',(61.5550077783217,3.03282455134599E-5,
47.5250194912663));
#163988=CARTESIAN_POINT('Ctrl Pts',(61.5550078322157,1.51641227338287E-5,
47.5250197971267));
#163989=CARTESIAN_POINT('Ctrl Pts',(61.5550078861458,-8.57747578934197E-15,
47.5250201029796));
#163990=CARTESIAN_POINT('Origin',(69.6316151486327,0.,39.48523201752));
#163991=CARTESIAN_POINT('',(61.7928511881971,-3.40955384291398E-10,48.8738964978212));
#163992=CARTESIAN_POINT('',(61.763385699346,8.81065254412669E-12,48.7067894065939));
#163993=CARTESIAN_POINT('',(60.4236626579685,-1.14504475720278E-15,41.1088424787055));
#163994=CARTESIAN_POINT('Ctrl Pts',(61.7928511881971,-6.81909623538039E-10,
48.8738964978212));
#163995=CARTESIAN_POINT('Ctrl Pts',(61.7927093875837,0.0398716337037261,
48.8730923065971));
#163996=CARTESIAN_POINT('Ctrl Pts',(61.7928201229409,0.079742808460378,
48.8722516099169));
#163997=CARTESIAN_POINT('Ctrl Pts',(61.7938970464417,0.197975584846006,
48.869648227374));
#163998=CARTESIAN_POINT('Ctrl Pts',(61.7955859471352,0.276324641715018,
48.8677791949698));
#163999=CARTESIAN_POINT('Ctrl Pts',(61.8077391834102,0.633772298995458,
48.858571281954));
#164000=CARTESIAN_POINT('Ctrl Pts',(61.82959410914,0.912294132295975,48.8494975486385));
#164001=CARTESIAN_POINT('Ctrl Pts',(61.90388876499,1.51567460582303,48.8252206613235));
#164002=CARTESIAN_POINT('Ctrl Pts',(61.9610202792514,1.83954707276695,48.8092283784813));
#164003=CARTESIAN_POINT('Ctrl Pts',(62.087930408233,2.38999814777087,48.7764440961858));
#164004=CARTESIAN_POINT('Ctrl Pts',(62.149629027767,2.61820050379103,48.7611466119104));
#164005=CARTESIAN_POINT('Ctrl Pts',(62.2735006171906,3.01653378061279,48.7312824940788));
#164006=CARTESIAN_POINT('Ctrl Pts',(62.3321599462423,3.18767622698851,48.7173889778356));
#164007=CARTESIAN_POINT('Ctrl Pts',(62.4326425833639,3.45551184770372,48.6939197693051));
#164008=CARTESIAN_POINT('Ctrl Pts',(62.4712527680553,3.55341518306191,48.6849673361731));
#164009=CARTESIAN_POINT('Ctrl Pts',(62.5487437909795,3.7406654284178,48.6671168763836));
#164010=CARTESIAN_POINT('Ctrl Pts',(62.5873896398572,3.83009901599484,48.658264697418));
#164011=CARTESIAN_POINT('Ctrl Pts',(62.6831346662027,4.04255724851014,48.6364477691766));
#164012=CARTESIAN_POINT('Ctrl Pts',(62.7415095785075,4.16495681714975,48.6232355320527));
#164013=CARTESIAN_POINT('Ctrl Pts',(63.0264122525956,4.73051261477613,48.5591593164579));
#164014=CARTESIAN_POINT('Ctrl Pts',(63.2849881828916,5.15589910065763,48.5020793761147));
#164015=CARTESIAN_POINT('Ctrl Pts',(63.7125017277984,5.74710375971109,48.4098170127609));
#164016=CARTESIAN_POINT('Ctrl Pts',(63.8561713553807,5.93080105228094,48.3791027442129));
#164017=CARTESIAN_POINT('Ctrl Pts',(64.1003557608425,6.21983194810889,48.3275080634672));
#164018=CARTESIAN_POINT('Ctrl Pts',(64.1967554870541,6.32862362780603,48.3072792530823));
#164019=CARTESIAN_POINT('Ctrl Pts',(64.3406191147498,6.48344999314284,48.2773295468307));
#164020=CARTESIAN_POINT('Ctrl Pts',(64.3860996658139,6.53135292177966,48.2678945160641));
#164021=CARTESIAN_POINT('Ctrl Pts',(64.4707106363186,6.6185713154146,48.2504073822016));
#164022=CARTESIAN_POINT('Ctrl Pts',(64.5096903100394,6.65803189240602,48.2423766014184));
#164023=CARTESIAN_POINT('Ctrl Pts',(64.6086993023588,6.75646608260662,48.2220383523451));
#164024=CARTESIAN_POINT('Ctrl Pts',(64.669179056021,6.8149663498546,48.209668672977));
#164025=CARTESIAN_POINT('Ctrl Pts',(65.0655988267846,7.18802062998159,48.1288906796568));
#164026=CARTESIAN_POINT('Ctrl Pts',(65.4235963300728,7.47747300199336,48.0572849906119));
#164027=CARTESIAN_POINT('Ctrl Pts',(66.0169565033158,7.88763976461308,47.9391000779253));
#164028=CARTESIAN_POINT('Ctrl Pts',(66.2387704597362,8.02728249550912,47.8950231730325));
#164029=CARTESIAN_POINT('Ctrl Pts',(66.6303863241417,8.25091993500563,47.8171782011556));
#164030=CARTESIAN_POINT('Ctrl Pts',(66.7974532858258,8.3395519942289,47.7839619079423));
#164031=CARTESIAN_POINT('Ctrl Pts',(67.0617408995793,8.46938770035125,47.7313625456761));
#164032=CARTESIAN_POINT('Ctrl Pts',(67.1571859119804,8.5142338026188,47.7123564639545));
#164033=CARTESIAN_POINT('Ctrl Pts',(67.3407148804679,8.59660126797913,47.675785125181));
#164034=CARTESIAN_POINT('Ctrl Pts',(67.4286593240644,8.63441206936909,47.6582499605551));
#164035=CARTESIAN_POINT('Ctrl Pts',(67.6373482034933,8.72025170719849,47.6166119098222));
#164036=CARTESIAN_POINT('Ctrl Pts',(67.7585419008783,8.76708392705567,47.5924093871011));
#164037=CARTESIAN_POINT('Ctrl Pts',(68.2431420010052,8.94246895398043,47.4955487795057));
#164038=CARTESIAN_POINT('Ctrl Pts',(68.6133134664131,9.05027439873143,47.4213533810061));
#164039=CARTESIAN_POINT('Ctrl Pts',(69.2852265247751,9.2001233660496,47.2866167086761));
#164040=CARTESIAN_POINT('Ctrl Pts',(69.5844658875582,9.25116307658516,47.2265956650692));
#164041=CARTESIAN_POINT('Ctrl Pts',(70.0523842120146,9.30682753616114,47.1330050204991));
#164042=CARTESIAN_POINT('Ctrl Pts',(70.2196190134392,9.32199080350287,47.0996088203838));
#164043=CARTESIAN_POINT('Ctrl Pts',(70.5039956188471,9.33976903456648,47.0429806418733));
#164044=CARTESIAN_POINT('Ctrl Pts',(70.6209418047642,9.34479206758022,47.0197391521012));
#164045=CARTESIAN_POINT('Ctrl Pts',(70.7964272605224,9.34890188912022,46.9849565986193));
#164046=CARTESIAN_POINT('Ctrl Pts',(70.8549073060047,9.34970129582141,46.9733808715733));
#164047=CARTESIAN_POINT('Ctrl Pts',(70.9642892004743,9.35013038770566,46.9517622846922));
#164048=CARTESIAN_POINT('Ctrl Pts',(71.015186904825,9.34989843097453,46.9417164022726));
#164049=CARTESIAN_POINT('Ctrl Pts',(71.142982625768,9.34823231706115,46.9165242015347));
#164050=CARTESIAN_POINT('Ctrl Pts',(71.219872796493,9.34624451319848,46.9013951541355));
#164051=CARTESIAN_POINT('Ctrl Pts',(71.5706797080047,9.33267703018759,46.8324735046096));
#164052=CARTESIAN_POINT('Ctrl Pts',(71.8440752444452,9.30957876278128,46.7790464154775));
#164053=CARTESIAN_POINT('Ctrl Pts',(72.4363754978243,9.23219786051485,46.6634312042488));
#164054=CARTESIAN_POINT('Ctrl Pts',(72.754315530605,9.17315748604154,46.6014513431682));
#164055=CARTESIAN_POINT('Ctrl Pts',(73.2946254946761,9.04248259108015,46.4957734989395));
#164056=CARTESIAN_POINT('Ctrl Pts',(73.5186064155076,8.97906475306848,46.4518612476887));
#164057=CARTESIAN_POINT('Ctrl Pts',(73.9095178036318,8.85188882900484,46.374910778791));
#164058=CARTESIAN_POINT('Ctrl Pts',(74.0774536022795,8.79170793759926,46.341748862393));
#164059=CARTESIAN_POINT('Ctrl Pts',(74.3402372603444,8.68867627423887,46.2896615924129));
#164060=CARTESIAN_POINT('Ctrl Pts',(74.4362866013123,8.64909806620124,46.270581084491));
#164061=CARTESIAN_POINT('Ctrl Pts',(74.6199761890769,8.56968460210561,46.2340049515081));
#164062=CARTESIAN_POINT('Ctrl Pts',(74.70770255296,8.53008873092478,46.2164985544831));
#164063=CARTESIAN_POINT('Ctrl Pts',(74.9160889544367,8.43200997118076,46.1748199196186));
#164064=CARTESIAN_POINT('Ctrl Pts',(75.0361295619263,8.37222776282541,46.1507343628081));
#164065=CARTESIAN_POINT('Ctrl Pts',(75.5907296749105,8.08052515010787,46.0391031358023));
#164066=CARTESIAN_POINT('Ctrl Pts',(76.0076924810794,7.81596351365729,45.9540952227733));
#164067=CARTESIAN_POINT('Ctrl Pts',(76.5870296794796,7.37892200492217,45.8350622137528));
#164068=CARTESIAN_POINT('Ctrl Pts',(76.7670142116694,7.23210274587378,45.7979446973591));
#164069=CARTESIAN_POINT('Ctrl Pts',(77.0501917030216,6.98267050576356,45.7394745499622));
#164070=CARTESIAN_POINT('Ctrl Pts',(77.1567774749319,6.88422311446124,45.7174496829604));
#164071=CARTESIAN_POINT('Ctrl Pts',(77.3084673362869,6.73734499443617,45.6861200206139));
#164072=CARTESIAN_POINT('Ctrl Pts',(77.3554003436349,6.69091709909592,45.6764288853439));
#164073=CARTESIAN_POINT('Ctrl Pts',(77.440854482312,6.60455500724864,45.6587930803067));
#164074=CARTESIAN_POINT('Ctrl Pts',(77.4795176196987,6.5647729666128,45.6508181128989));
#164075=CARTESIAN_POINT('Ctrl Pts',(77.5759639912022,6.46373624165309,45.6309317177989));
#164076=CARTESIAN_POINT('Ctrl Pts',(77.6332840098771,6.40202715843781,45.6191191804156));
#164077=CARTESIAN_POINT('Ctrl Pts',(77.9988113722254,5.9976017671801,45.5437883239921));
#164078=CARTESIAN_POINT('Ctrl Pts',(78.2824166163544,5.63260774015445,45.485299976364));
#164079=CARTESIAN_POINT('Ctrl Pts',(78.6840330175363,5.02773899565478,45.4009246579117));
#164080=CARTESIAN_POINT('Ctrl Pts',(78.8207045613723,4.80164182792807,45.3718606754667));
#164081=CARTESIAN_POINT('Ctrl Pts',(79.0394400357541,4.40245908022573,45.3244992077555));
#164082=CARTESIAN_POINT('Ctrl Pts',(79.1260827061336,4.23216267970861,45.3054638953936));
#164083=CARTESIAN_POINT('Ctrl Pts',(79.2529198919031,3.96275686917369,45.2771007622597));
#164084=CARTESIAN_POINT('Ctrl Pts',(79.2967124299097,3.86546157438083,45.2672024067856));
#164085=CARTESIAN_POINT('Ctrl Pts',(79.3771085221401,3.67837032000539,45.2488161775587));
#164086=CARTESIAN_POINT('Ctrl Pts',(79.4139980537783,3.58871697754349,45.2402833708288));
#164087=CARTESIAN_POINT('Ctrl Pts',(79.4977058625176,3.3759679920793,45.2206828505326));
#164088=CARTESIAN_POINT('Ctrl Pts',(79.543342204226,3.25241260877376,45.2098031242783));
#164089=CARTESIAN_POINT('Ctrl Pts',(79.7141143293387,2.75834538967054,45.1682786333352));
#164090=CARTESIAN_POINT('Ctrl Pts',(79.8187578690572,2.38090392850897,45.14090273317));
#164091=CARTESIAN_POINT('Ctrl Pts',(79.9635697487114,1.69569555389937,45.0991056934429));
#164092=CARTESIAN_POINT('Ctrl Pts',(80.0126028905576,1.39048155231731,45.0832004164284));
#164093=CARTESIAN_POINT('Ctrl Pts',(80.0655137982829,0.913382414859032,
45.062786091966));
#164094=CARTESIAN_POINT('Ctrl Pts',(80.0797689913388,0.742950917010975,
45.0563658147369));
#164095=CARTESIAN_POINT('Ctrl Pts',(80.0961587154085,0.453152887005338,
45.0469930909051));
#164096=CARTESIAN_POINT('Ctrl Pts',(80.1006549660521,0.333977130123532,
45.0435802396458));
#164097=CARTESIAN_POINT('Ctrl Pts',(80.1040441138188,0.155152760200764,
45.0391436857227));
#164098=CARTESIAN_POINT('Ctrl Pts',(80.1046148848364,0.0955564107881091,
45.0377790476352));
#164099=CARTESIAN_POINT('Ctrl Pts',(80.1046383312521,-0.0159141927496996,
45.0354433926729));
#164100=CARTESIAN_POINT('Ctrl Pts',(80.1042264911596,-0.0677848918374825,
45.0344447366344));
#164101=CARTESIAN_POINT('Ctrl Pts',(80.1021303232615,-0.198027377199186,
45.0321557167181));
#164102=CARTESIAN_POINT('Ctrl Pts',(80.0999032129076,-0.276388431176385,
45.0309769550136));
#164103=CARTESIAN_POINT('Ctrl Pts',(80.0853380512284,-0.63365742266964,
45.0264838144944));
#164104=CARTESIAN_POINT('Ctrl Pts',(80.0617200238406,-0.911989439126223,
45.0254315872871));
#164105=CARTESIAN_POINT('Ctrl Pts',(79.9836587278326,-1.51518432935195,
45.0280224367092));
#164106=CARTESIAN_POINT('Ctrl Pts',(79.9245200285978,-1.83905941027557,
45.032531759564));
#164107=CARTESIAN_POINT('Ctrl Pts',(79.794059522035,-2.3896018148766,45.04512747728));
#164108=CARTESIAN_POINT('Ctrl Pts',(79.7308352654742,-2.61789081272124,
45.0518557524078));
#164109=CARTESIAN_POINT('Ctrl Pts',(79.6041898877887,-3.01635299916493,
45.0661621440667));
#164110=CARTESIAN_POINT('Ctrl Pts',(79.544304578152,-3.18753873037347,45.0731704224207));
#164111=CARTESIAN_POINT('Ctrl Pts',(79.441838940388,-3.4554245847302,45.0854854650915));
#164112=CARTESIAN_POINT('Ctrl Pts',(79.402493302489,-3.5533356432085,45.0902786024331));
#164113=CARTESIAN_POINT('Ctrl Pts',(79.3235700024699,-3.74059102650108,
45.1000081353203));
#164114=CARTESIAN_POINT('Ctrl Pts',(79.2842291712769,-3.83002216813102,
45.1049071898515));
#164115=CARTESIAN_POINT('Ctrl Pts',(79.1868088006053,-4.04245865076035,
45.117151093802));
#164116=CARTESIAN_POINT('Ctrl Pts',(79.127446579768,-4.16483929652454,45.1246995865182));
#164117=CARTESIAN_POINT('Ctrl Pts',(78.8376881397524,-4.73065622344361,
45.1619455053558));
#164118=CARTESIAN_POINT('Ctrl Pts',(78.5750063112216,-5.15629868667662,
45.1967698974858));
#164119=CARTESIAN_POINT('Ctrl Pts',(78.1415872119472,-5.74758144430734,
45.2563100328585));
#164120=CARTESIAN_POINT('Ctrl Pts',(77.9961710005488,-5.93113909249284,
45.2765733795583));
#164121=CARTESIAN_POINT('Ctrl Pts',(77.749207677565,-6.2199876850907,45.3115866262057));
#164122=CARTESIAN_POINT('Ctrl Pts',(77.651742866081,-6.3287306452149,45.3255428141669));
#164123=CARTESIAN_POINT('Ctrl Pts',(77.506360183959,-6.48350283982889,45.3465966458874));
#164124=CARTESIAN_POINT('Ctrl Pts',(77.4604018247016,-6.53139845271807,
45.3532849810303));
#164125=CARTESIAN_POINT('Ctrl Pts',(77.3749170867828,-6.61861123522454,
45.365790480238));
#164126=CARTESIAN_POINT('Ctrl Pts',(77.3355394776719,-6.65807334050427,
45.3715761607064));
#164127=CARTESIAN_POINT('Ctrl Pts',(77.2355293345143,-6.75652202434567,
45.3863299358669));
#164128=CARTESIAN_POINT('Ctrl Pts',(77.1744519297252,-6.81503491003287,
45.3953936982221));
#164129=CARTESIAN_POINT('Ctrl Pts',(76.7742163553425,-7.18816839315752,
45.4550852244507));
#164130=CARTESIAN_POINT('Ctrl Pts',(76.4132278982452,-7.47767560706471,
45.5102544302851));
#164131=CARTESIAN_POINT('Ctrl Pts',(75.8151932141065,-7.88782668734451,
45.6021440598486));
#164132=CARTESIAN_POINT('Ctrl Pts',(75.5917464975128,-8.02741820785937,
45.6365800868764));
#164133=CARTESIAN_POINT('Ctrl Pts',(75.1972226196877,-8.25098903860689,
45.6973549638813));
#164134=CARTESIAN_POINT('Ctrl Pts',(75.0289016541265,-8.33960163458169,
45.7232772962621));
#164135=CARTESIAN_POINT('Ctrl Pts',(74.7625999361083,-8.46941645347655,
45.7642359791166));
#164136=CARTESIAN_POINT('Ctrl Pts',(74.6664157343671,-8.51425929583976,
45.7790194117436));
#164137=CARTESIAN_POINT('Ctrl Pts',(74.481450253293,-8.59662388566012,45.8074236572265));
#164138=CARTESIAN_POINT('Ctrl Pts',(74.3928102552396,-8.63443482705536,
45.8210250466622));
#164139=CARTESIAN_POINT('Ctrl Pts',(74.182450667112,-8.72027902564148,45.8532761872953));
#164140=CARTESIAN_POINT('Ctrl Pts',(74.0602746430061,-8.76711515896276,
45.8719859917722));
#164141=CARTESIAN_POINT('Ctrl Pts',(73.5709789811025,-8.94277846001009,
45.9468309314503));
#164142=CARTESIAN_POINT('Ctrl Pts',(73.1969443301631,-9.05075890642989,
46.0038392179424));
#164143=CARTESIAN_POINT('Ctrl Pts',(72.5143651718206,-9.20153563227824,
46.1078134436371));
#164144=CARTESIAN_POINT('Ctrl Pts',(72.2082869265093,-9.25299899086914,
46.1544213795432));
#164145=CARTESIAN_POINT('Ctrl Pts',(71.7351189661655,-9.30801541318731,
46.2267447213101));
#164146=CARTESIAN_POINT('Ctrl Pts',(71.5695011866917,-9.32270911040497,
46.2521113910088));
#164147=CARTESIAN_POINT('Ctrl Pts',(71.2872907903927,-9.34000785246016,
46.2954911652769));
#164148=CARTESIAN_POINT('Ctrl Pts',(71.1708687670721,-9.34491212923875,
46.3134318333393));
#164149=CARTESIAN_POINT('Ctrl Pts',(70.9957504101543,-9.34893637020397,
46.340507940003));
#164150=CARTESIAN_POINT('Ctrl Pts',(70.9370961065956,-9.34971918461126,
46.3495920779163));
#164151=CARTESIAN_POINT('Ctrl Pts',(70.827670542458,-9.35012556127216,46.3665717061112));
#164152=CARTESIAN_POINT('Ctrl Pts',(70.776902038224,-9.34989080110659,46.3744628303659));
#164153=CARTESIAN_POINT('Ctrl Pts',(70.6486429722421,-9.34822814954453,
46.394429272106));
#164154=CARTESIAN_POINT('Ctrl Pts',(70.5711658249032,-9.34623704442709,
46.4065183953776));
#164155=CARTESIAN_POINT('Ctrl Pts',(70.2184319281362,-9.33267623374973,
46.4616600380233));
#164156=CARTESIAN_POINT('Ctrl Pts',(69.9437874759586,-9.30963798221351,
46.5048769460366));
#164157=CARTESIAN_POINT('Ctrl Pts',(69.3481894664989,-9.23241160402367,
46.5987296503087));
#164158=CARTESIAN_POINT('Ctrl Pts',(69.0282183267463,-9.1734172006384,46.6492308187572));
#164159=CARTESIAN_POINT('Ctrl Pts',(68.4841093852778,-9.04276693141672,
46.7347615984483));
#164160=CARTESIAN_POINT('Ctrl Pts',(68.2583898464631,-8.97931075027964,
46.7701396476123));
#164161=CARTESIAN_POINT('Ctrl Pts',(67.8643962464191,-8.85205490638486,
46.8315827518995));
#164162=CARTESIAN_POINT('Ctrl Pts',(67.6951325365816,-8.79184280688282,
46.8578760183822));
#164163=CARTESIAN_POINT('Ctrl Pts',(67.4302498777407,-8.68876870089034,
46.8988278856758));
#164164=CARTESIAN_POINT('Ctrl Pts',(67.3334468299633,-8.64918510982089,
46.9137520736513));
#164165=CARTESIAN_POINT('Ctrl Pts',(67.1483118208652,-8.56977075447606,
46.942209475053));
#164166=CARTESIAN_POINT('Ctrl Pts',(67.0598948902342,-8.53018026866594,
46.9557620994396));
#164167=CARTESIAN_POINT('Ctrl Pts',(66.8498779073544,-8.43213454901513,
46.9878607591748));
#164168=CARTESIAN_POINT('Ctrl Pts',(66.7288885856046,-8.37238204604089,
47.0062766004639));
#164169=CARTESIAN_POINT('Ctrl Pts',(66.1688744394223,-8.08035568204751,
47.0911658075432));
#164170=CARTESIAN_POINT('Ctrl Pts',(65.7473152088772,-7.81532259479731,
47.153992251449));
#164171=CARTESIAN_POINT('Ctrl Pts',(65.1619997861138,-7.37792841477651,
47.2403105904215));
#164172=CARTESIAN_POINT('Ctrl Pts',(64.9805383962621,-7.23135848563247,
47.2669362214911));
#164173=CARTESIAN_POINT('Ctrl Pts',(64.6949155489118,-6.98230167254136,
47.308774952385));
#164174=CARTESIAN_POINT('Ctrl Pts',(64.5873517124558,-6.88396045552704,
47.3245142562146));
#164175=CARTESIAN_POINT('Ctrl Pts',(64.434235683113,-6.73721076280984,47.3469343340552));
#164176=CARTESIAN_POINT('Ctrl Pts',(64.3868375929826,-6.690799748617,47.3538768930162));
#164177=CARTESIAN_POINT('Ctrl Pts',(64.3005197920082,-6.60444965553853,
47.3665295639714));
#164178=CARTESIAN_POINT('Ctrl Pts',(64.2614567372036,-6.56466225397752,
47.3722597109192));
#164179=CARTESIAN_POINT('Ctrl Pts',(64.1639874271476,-6.46358280133991,
47.3865647777498));
#164180=CARTESIAN_POINT('Ctrl Pts',(64.1060511807115,-6.40183548166547,
47.3950740674123));
#164181=CARTESIAN_POINT('Ctrl Pts',(63.7365884459327,-5.99714766694451,
47.4493354637004));
#164182=CARTESIAN_POINT('Ctrl Pts',(63.449932645172,-5.6319028390746,47.4913947660234));
#164183=CARTESIAN_POINT('Ctrl Pts',(63.0437185164782,-5.02692974599468,
47.5494603011872));
#164184=CARTESIAN_POINT('Ctrl Pts',(62.905486568237,-4.80101243802735,47.5688731951127));
#164185=CARTESIAN_POINT('Ctrl Pts',(62.6839232214926,-4.40210250558855,
47.599154274381));
#164186=CARTESIAN_POINT('Ctrl Pts',(62.5960477146251,-4.23189210386382,
47.6108930877713));
#164187=CARTESIAN_POINT('Ctrl Pts',(62.467215297971,-3.96258927756738,47.6276136610573));
#164188=CARTESIAN_POINT('Ctrl Pts',(62.4226871186887,-3.86530838290369,
47.6332889398925));
#164189=CARTESIAN_POINT('Ctrl Pts',(62.340858775073,-3.67822667365684,47.6435074473755));
#164190=CARTESIAN_POINT('Ctrl Pts',(62.303275164339,-3.58856817504586,47.648106136056));
#164191=CARTESIAN_POINT('Ctrl Pts',(62.2178993929925,-3.3757775421119,47.6583186342856));
#164192=CARTESIAN_POINT('Ctrl Pts',(62.1712835390476,-3.25218515070423,
47.6637045858437));
#164193=CARTESIAN_POINT('Ctrl Pts',(61.995821435896,-2.75584633495742,47.6831779392435));
#164194=CARTESIAN_POINT('Ctrl Pts',(61.8876270265883,-2.37607830650069,
47.6932745526513));
#164195=CARTESIAN_POINT('Ctrl Pts',(61.7226473671648,-1.62151959949796,
47.7044558437569));
#164196=CARTESIAN_POINT('Ctrl Pts',(61.6640252952989,-1.24789122720521,
47.7058983580691));
#164197=CARTESIAN_POINT('Ctrl Pts',(61.6151903277049,-0.739965160821248,
47.7028607836474));
#164198=CARTESIAN_POINT('Ctrl Pts',(61.6052813083504,-0.607899836463236,
47.7016209296473));
#164199=CARTESIAN_POINT('Ctrl Pts',(61.5927768348471,-0.376140884189838,
47.6986919183964));
#164200=CARTESIAN_POINT('Ctrl Pts',(61.5889797094579,-0.276530595462918,
47.6971898566419));
#164201=CARTESIAN_POINT('Ctrl Pts',(61.5855140036737,-0.12102090730317,
47.6944797824192));
#164202=CARTESIAN_POINT('Ctrl Pts',(61.5847645279554,-0.065150117516361,
47.6934326383007));
#164203=CARTESIAN_POINT('Ctrl Pts',(61.5844968904708,-0.0061849436233789,
47.6922517218026));
#164204=CARTESIAN_POINT('Ctrl Pts',(61.5844843731439,-0.00309247043366816,
47.6921895677981));
#164205=CARTESIAN_POINT('Ctrl Pts',(61.5844733749945,-2.11872094351994E-11,
47.6921271941932));
#164206=CARTESIAN_POINT('Ctrl Pts',(61.5550078861458,-8.57747578934197E-15,
47.5250201029796));
#164207=CARTESIAN_POINT('Ctrl Pts',(61.5551466499392,-0.0390177391739191,
47.5258070715583));
#164208=CARTESIAN_POINT('Ctrl Pts',(61.5555246228054,-0.078035244936701,
47.5265441818857));
#164209=CARTESIAN_POINT('Ctrl Pts',(61.5569077936725,-0.165457667185358,
47.5280855343779));
#164210=CARTESIAN_POINT('Ctrl Pts',(61.5580420633262,-0.21385988472972,
47.5288631953164));
#164211=CARTESIAN_POINT('Ctrl Pts',(61.5633215687984,-0.383870843256392,
47.5313330557453));
#164212=CARTESIAN_POINT('Ctrl Pts',(61.5694253014728,-0.505412079323531,
47.5326283672832));
#164213=CARTESIAN_POINT('Ctrl Pts',(61.6137244421188,-1.14327639601798,
47.5370539152006));
#164214=CARTESIAN_POINT('Ctrl Pts',(61.6916432728872,-1.6559795486642,47.532472516678));
#164215=CARTESIAN_POINT('Ctrl Pts',(61.86562232674,-2.38999811288596,47.5156723695157));
#164216=CARTESIAN_POINT('Ctrl Pts',(61.928832113267,-2.61820047653147,47.5089451318185));
#164217=CARTESIAN_POINT('Ctrl Pts',(62.0554474642774,-3.01653376469872,
47.4946416439468));
#164218=CARTESIAN_POINT('Ctrl Pts',(62.115321066375,-3.18767621488445,47.4876346063985));
#164219=CARTESIAN_POINT('Ctrl Pts',(62.2177708024606,-3.45551184002182,
47.4753213623619));
#164220=CARTESIAN_POINT('Ctrl Pts',(62.2571144207432,-3.55341517606029,
47.4705284367934));
#164221=CARTESIAN_POINT('Ctrl Pts',(62.3360373800074,-3.74066542186744,
47.4607988913694));
#164222=CARTESIAN_POINT('Ctrl Pts',(62.3753802223634,-3.83009900922906,
47.4558995598736));
#164223=CARTESIAN_POINT('Ctrl Pts',(62.4728129449329,-4.04255723982814,
47.4436540388593));
#164224=CARTESIAN_POINT('Ctrl Pts',(62.5321862695213,-4.16495680680075,
47.4361040848444));
#164225=CARTESIAN_POINT('Ctrl Pts',(62.8218225772558,-4.73051262752732,
47.398873577017));
#164226=CARTESIAN_POINT('Ctrl Pts',(63.0843269759402,-5.15589913604641,
47.3640729969055));
#164227=CARTESIAN_POINT('Ctrl Pts',(63.5176138977982,-5.74710380199329,
47.304553013241));
#164228=CARTESIAN_POINT('Ctrl Pts',(63.6631240768806,-5.9308010822008,47.2842770792455));
#164229=CARTESIAN_POINT('Ctrl Pts',(63.910228768393,-6.21983196189127,47.2492442363948));
#164230=CARTESIAN_POINT('Ctrl Pts',(64.0077335368504,-6.32862363727644,
47.2352824525607));
#164231=CARTESIAN_POINT('Ctrl Pts',(64.1531645247452,-6.48344999781946,
47.2142217125675));
#164232=CARTESIAN_POINT('Ctrl Pts',(64.1991292329824,-6.53135292580872,
47.207532476842));
#164233=CARTESIAN_POINT('Ctrl Pts',(64.2846184892329,-6.61857131894665,
47.1950263512879));
#164234=CARTESIAN_POINT('Ctrl Pts',(64.3239940899608,-6.65803189607302,
47.1892409831086));
#164235=CARTESIAN_POINT('Ctrl Pts',(64.4239882017162,-6.75646608755569,
47.1744896157259));
#164236=CARTESIAN_POINT('Ctrl Pts',(64.485051260719,-6.81496635591992,47.1654280179423));
#164237=CARTESIAN_POINT('Ctrl Pts',(64.8851917031561,-7.18802064291156,
47.1057509541167));
#164238=CARTESIAN_POINT('Ctrl Pts',(65.246089911098,-7.47747301965684,47.0505959331056));
#164239=CARTESIAN_POINT('Ctrl Pts',(65.8440877113012,-7.88763978087938,
46.9587122914352));
#164240=CARTESIAN_POINT('Ctrl Pts',(66.0675998329727,-8.02728250731837,
46.9242661934201));
#164241=CARTESIAN_POINT('Ctrl Pts',(66.4622229107417,-8.25091994101796,
46.8634760263164));
#164242=CARTESIAN_POINT('Ctrl Pts',(66.6305751404579,-8.33955199854741,
46.8375488661788));
#164243=CARTESIAN_POINT('Ctrl Pts',(66.8969142990296,-8.46938770285203,
46.7965844117256));
#164244=CARTESIAN_POINT('Ctrl Pts',(66.9931037352125,-8.51423380483586,
46.7818001697188));
#164245=CARTESIAN_POINT('Ctrl Pts',(67.1780726868272,-8.59660126994594,
46.7533953828372));
#164246=CARTESIAN_POINT('Ctrl Pts',(67.2667108111955,-8.63441207134806,
46.7397942764122));
#164247=CARTESIAN_POINT('Ctrl Pts',(67.4770552646312,-8.72025170957431,
46.7075454447762));
#164248=CARTESIAN_POINT('Ctrl Pts',(67.5992178392097,-8.76708392977196,
46.6888376908535));
#164249=CARTESIAN_POINT('Ctrl Pts',(68.0877213237592,-8.94246898040873,
46.6141138830279));
#164250=CARTESIAN_POINT('Ctrl Pts',(68.4609451081589,-9.05027444007471,
46.5572286433543));
#164251=CARTESIAN_POINT('Ctrl Pts',(69.1384202529569,-9.20012355536855,
46.454031785933));
#164252=CARTESIAN_POINT('Ctrl Pts',(69.4401423684263,-9.25116333983993,
46.4080871231519));
#164253=CARTESIAN_POINT('Ctrl Pts',(69.9118519146182,-9.30682771093848,
46.335996027152));
#164254=CARTESIAN_POINT('Ctrl Pts',(70.0804229631028,-9.32199090897221,
46.3101805850801));
#164255=CARTESIAN_POINT('Ctrl Pts',(70.3670168959907,-9.33976906949828,
46.2661312373467));
#164256=CARTESIAN_POINT('Ctrl Pts',(70.4848592141131,-9.34479208510376,
46.2479731742685));
#164257=CARTESIAN_POINT('Ctrl Pts',(70.6616576905881,-9.34890189414368,
46.2206385601175));
#164258=CARTESIAN_POINT('Ctrl Pts',(70.7205700520679,-9.34970129843407,
46.2115148376248));
#164259=CARTESIAN_POINT('Ctrl Pts',(70.8307493783468,-9.35013038734498,
46.1944188567541));
#164260=CARTESIAN_POINT('Ctrl Pts',(70.8820134822541,-9.34989842911278,
46.1864508561971));
#164261=CARTESIAN_POINT('Ctrl Pts',(71.0107185141546,-9.34823231006586,
46.1664150555058));
#164262=CARTESIAN_POINT('Ctrl Pts',(71.0881461623868,-9.34624450066235,
46.1543337094176));
#164263=CARTESIAN_POINT('Ctrl Pts',(71.4413678007677,-9.33267705949493,
46.0991160975365));
#164264=CARTESIAN_POINT('Ctrl Pts',(71.7165470145877,-9.30957899594627,
46.0558146266122));
#164265=CARTESIAN_POINT('Ctrl Pts',(72.3126682665991,-9.23219861293737,
45.9618790324743));
#164266=CARTESIAN_POINT('Ctrl Pts',(72.6326325541485,-9.17315840028106,
45.9113791504871));
#164267=CARTESIAN_POINT('Ctrl Pts',(73.1765026348197,-9.0424835919843,45.8258868138484));
#164268=CARTESIAN_POINT('Ctrl Pts',(73.4019955279895,-8.97906561901957,
45.7905447187263));
#164269=CARTESIAN_POINT('Ctrl Pts',(73.795651876037,-8.85188941371181,45.7291547498995));
#164270=CARTESIAN_POINT('Ctrl Pts',(73.9648023501125,-8.79170841246524,
45.7028792692916));
#164271=CARTESIAN_POINT('Ctrl Pts',(74.2295535742093,-8.68867659973452,
45.6619479156828));
#164272=CARTESIAN_POINT('Ctrl Pts',(74.3263364205575,-8.64909837275343,
45.6470269075817));
#164273=CARTESIAN_POINT('Ctrl Pts',(74.5114579923559,-8.56968490555063,
45.618571683026));
#164274=CARTESIAN_POINT('Ctrl Pts',(74.5998813268982,-8.5300890533527,45.6050181348481));
#164275=CARTESIAN_POINT('Ctrl Pts',(74.809955222012,-8.43201041005115,45.5729109238203));
#164276=CARTESIAN_POINT('Ctrl Pts',(74.9309940655172,-8.37222830638353,
45.5544876642797));
#164277=CARTESIAN_POINT('Ctrl Pts',(75.4903302536429,-8.08052453772989,
45.4697019241712));
#164278=CARTESIAN_POINT('Ctrl Pts',(75.9112239243894,-7.81596122060783,
45.4069732045745));
#164279=CARTESIAN_POINT('Ctrl Pts',(76.4963352276659,-7.37891845664684,
45.3206825547105));
#164280=CARTESIAN_POINT('Ctrl Pts',(76.678159003098,-7.23210008835748,45.2940034671813));
#164281=CARTESIAN_POINT('Ctrl Pts',(76.9642550736277,-6.98266918936499,
45.2520952760861));
#164282=CARTESIAN_POINT('Ctrl Pts',(77.0719454317692,-6.88422217714014,
45.2363374664093));
#164283=CARTESIAN_POINT('Ctrl Pts',(77.225202146662,-6.73734451562587,45.2138968045589));
#164284=CARTESIAN_POINT('Ctrl Pts',(77.2726192427457,-6.69091668052719,
45.2069514689035));
#164285=CARTESIAN_POINT('Ctrl Pts',(77.3589516146158,-6.60455463154549,
45.1942966756078));
#164286=CARTESIAN_POINT('Ctrl Pts',(77.3980106932074,-6.56477257182652,
45.188567119731));
#164287=CARTESIAN_POINT('Ctrl Pts',(77.4954423192641,-6.46373569462105,
45.1742675968315));
#164288=CARTESIAN_POINT('Ctrl Pts',(77.5533457608891,-6.40202647514572,
45.1657631327824));
#164289=CARTESIAN_POINT('Ctrl Pts',(77.9225945180331,-5.99760019624139,
45.1115331558459));
#164290=CARTESIAN_POINT('Ctrl Pts',(78.2091009640789,-5.63260532935765,
45.06949544635));
#164291=CARTESIAN_POINT('Ctrl Pts',(78.6153548458468,-5.0277362445293,45.0114214416589));
#164292=CARTESIAN_POINT('Ctrl Pts',(78.7537240859896,-4.8016396884229,44.9919882995805));
#164293=CARTESIAN_POINT('Ctrl Pts',(78.9754661633144,-4.40245786836224,
44.9616816701779));
#164294=CARTESIAN_POINT('Ctrl Pts',(79.063393923333,-4.23216176019283,44.9499354992954));
#164295=CARTESIAN_POINT('Ctrl Pts',(79.1922824622699,-3.96275629974334,
44.9332072798286));
#164296=CARTESIAN_POINT('Ctrl Pts',(79.2368193941881,-3.86546105389666,
44.9275307655133));
#164297=CARTESIAN_POINT('Ctrl Pts',(79.3186554432657,-3.67836983199058,
44.9173110904372));
#164298=CARTESIAN_POINT('Ctrl Pts',(79.3562386570575,-3.58871647202851,
44.912712343258));
#164299=CARTESIAN_POINT('Ctrl Pts',(79.4416020820573,-3.37596734514096,
44.9025010467075));
#164300=CARTESIAN_POINT('Ctrl Pts',(79.4882073372486,-3.25241183615882,
44.8971160936505));
#164301=CARTESIAN_POINT('Ctrl Pts',(79.6628853659389,-2.75833735794606,
44.8777285700723));
#164302=CARTESIAN_POINT('Ctrl Pts',(79.7705828292355,-2.38088847080519,
44.867663202802));
#164303=CARTESIAN_POINT('Ctrl Pts',(79.9209728102791,-1.6955995292544,44.8574101028781));
#164304=CARTESIAN_POINT('Ctrl Pts',(79.9724968997835,-1.390311142986,44.8555861998798));
#164305=CARTESIAN_POINT('Ctrl Pts',(80.0291897862859,-0.913183433070077,
44.8566749372101));
#164306=CARTESIAN_POINT('Ctrl Pts',(80.0447736721481,-0.742798737011347,
44.8578326514166));
#164307=CARTESIAN_POINT('Ctrl Pts',(80.0633729428985,-0.45307008460399,
44.8610342535038));
#164308=CARTESIAN_POINT('Ctrl Pts',(80.068763381637,-0.333916737630476,
44.8627032990736));
#164309=CARTESIAN_POINT('Ctrl Pts',(80.0734641142772,-0.155118865850148,
44.8657128003228));
#164310=CARTESIAN_POINT('Ctrl Pts',(80.0744669279504,-0.0955265730669187,
44.8667998810079));
#164311=CARTESIAN_POINT('Ctrl Pts',(80.0752874772849,0.0159413341490429,
44.8689866509228));
#164312=CARTESIAN_POINT('Ctrl Pts',(80.0752418806346,0.0678133948819915,
44.870065988658));
#164313=CARTESIAN_POINT('Ctrl Pts',(80.0740545116948,0.198066253930946,
44.872934184593));
#164314=CARTESIAN_POINT('Ctrl Pts',(80.0723643185048,0.276436314977128,
44.8748038435572));
#164315=CARTESIAN_POINT('Ctrl Pts',(80.0602153783642,0.633609941853107,
44.8840054660573));
#164316=CARTESIAN_POINT('Ctrl Pts',(80.0383926790477,0.911838032421433,
44.893068252948));
#164317=CARTESIAN_POINT('Ctrl Pts',(79.9641819924431,1.51493124829092,44.9173252648197));
#164318=CARTESIAN_POINT('Ctrl Pts',(79.9070763060138,1.83880768724944,44.9333129482378));
#164319=CARTESIAN_POINT('Ctrl Pts',(79.7801803750855,2.38939724846813,44.9660968304035));
#164320=CARTESIAN_POINT('Ctrl Pts',(79.7184606004295,2.61773097458111,44.9814003407129));
#164321=CARTESIAN_POINT('Ctrl Pts',(79.5945447213174,3.01625970548475,45.0112758931591));
#164322=CARTESIAN_POINT('Ctrl Pts',(79.5358680677186,3.18746777811519,45.025173712915));
#164323=CARTESIAN_POINT('Ctrl Pts',(79.4353618405169,3.45537956016921,45.0486486052679));
#164324=CARTESIAN_POINT('Ctrl Pts',(79.3967486683343,3.55329460465372,45.0576017840323));
#164325=CARTESIAN_POINT('Ctrl Pts',(79.3192571654795,3.74055264121777,45.0754524385989));
#164326=CARTESIAN_POINT('Ctrl Pts',(79.2806143248932,3.82998252195275,45.0843039694124));
#164327=CARTESIAN_POINT('Ctrl Pts',(79.1848877315677,4.04240778784193,45.1061167971568));
#164328=CARTESIAN_POINT('Ctrl Pts',(79.1265293936778,4.16477867426913,45.1193253589925));
#164329=CARTESIAN_POINT('Ctrl Pts',(78.8414452200882,4.73072936788794,45.1834428390304));
#164330=CARTESIAN_POINT('Ctrl Pts',(78.5826047965841,5.15650301509456,45.2405807210477));
#164331=CARTESIAN_POINT('Ctrl Pts',(78.1548929060647,5.74782591547893,45.3328828326126));
#164332=CARTESIAN_POINT('Ctrl Pts',(78.0113632840991,5.93131211553293,45.3635663948128));
#164333=CARTESIAN_POINT('Ctrl Pts',(77.7673898535157,6.22006742031824,45.4151158154594));
#164334=CARTESIAN_POINT('Ctrl Pts',(77.671049793879,6.32878544188141,45.4353319131716));
#164335=CARTESIAN_POINT('Ctrl Pts',(77.5272583743304,6.48352990604932,45.46526645379));
#164336=CARTESIAN_POINT('Ctrl Pts',(77.4817873108411,6.53142177293023,45.4746994806034));
#164337=CARTESIAN_POINT('Ctrl Pts',(77.3971830833238,6.61863168363854,45.4921851679235));
#164338=CARTESIAN_POINT('Ctrl Pts',(77.3582003927593,6.65809457282074,45.5002165439707));
#164339=CARTESIAN_POINT('Ctrl Pts',(77.2591673676685,6.75655068466948,45.5205596644514));
#164340=CARTESIAN_POINT('Ctrl Pts',(77.1986661035534,6.81507003666324,45.5329336887519));
#164341=CARTESIAN_POINT('Ctrl Pts',(76.8021021880893,7.18824546712365,45.613740635306));
#164342=CARTESIAN_POINT('Ctrl Pts',(76.4439674282961,7.47778191758882,45.6853731746204));
#164343=CARTESIAN_POINT('Ctrl Pts',(75.8505507713923,7.88792505719625,45.8035688445681));
#164344=CARTESIAN_POINT('Ctrl Pts',(75.6288358823475,8.0274896321279,45.847626050178));
#164345=CARTESIAN_POINT('Ctrl Pts',(75.2373702839884,8.25102541207991,45.9254411657672));
#164346=CARTESIAN_POINT('Ctrl Pts',(75.0703506874581,8.33962776470298,45.9586480616816));
#164347=CARTESIAN_POINT('Ctrl Pts',(74.8061197910239,8.46943159045896,46.0112361559338));
#164348=CARTESIAN_POINT('Ctrl Pts',(74.7106827095551,8.51427271694368,46.0302406658211));
#164349=CARTESIAN_POINT('Ctrl Pts',(74.5271590011423,8.59663579344307,46.0668109694259));
#164350=CARTESIAN_POINT('Ctrl Pts',(74.4392117213579,8.63444680875874,46.0843467064769));
#164351=CARTESIAN_POINT('Ctrl Pts',(74.2304999226481,8.72029340928881,46.1259893476084));
#164352=CARTESIAN_POINT('Ctrl Pts',(74.1092858588738,8.76713160347592,46.1501959514979));
#164353=CARTESIAN_POINT('Ctrl Pts',(73.623472004764,8.94294650236137,46.2472992278547));
#164354=CARTESIAN_POINT('Ctrl Pts',(73.2520583667685,9.05102226038947,46.321744446618));
#164355=CARTESIAN_POINT('Ctrl Pts',(72.5725213296973,9.20225946910197,46.4580100925124));
#164356=CARTESIAN_POINT('Ctrl Pts',(72.266807608604,9.25392665468341,46.5193298191909));
#164357=CARTESIAN_POINT('Ctrl Pts',(71.7967307155527,9.30861069770923,46.6133379064377));
#164358=CARTESIAN_POINT('Ctrl Pts',(71.6338984807729,9.32307020107794,46.645849649464));
#164359=CARTESIAN_POINT('Ctrl Pts',(71.3560634116172,9.34012859970737,46.7011688961548));
#164360=CARTESIAN_POINT('Ctrl Pts',(71.2412404937854,9.34497303030257,46.7239862122937));
#164361=CARTESIAN_POINT('Ctrl Pts',(71.0682681832646,9.34895390789572,46.7582687371924));
#164362=CARTESIAN_POINT('Ctrl Pts',(71.0101747427237,9.34972824786854,46.7697673586588));
#164363=CARTESIAN_POINT('Ctrl Pts',(70.901627033317,9.3501241138955,46.7912201515143));
#164364=CARTESIAN_POINT('Ctrl Pts',(70.8511767883932,9.34988403705377,46.8011773995548));
#164365=CARTESIAN_POINT('Ctrl Pts',(70.7234825994232,9.34820305143747,46.8263491217628));
#164366=CARTESIAN_POINT('Ctrl Pts',(70.6462466740132,9.34619205452021,46.8415458203407));
#164367=CARTESIAN_POINT('Ctrl Pts',(70.2968982520604,9.33259629184533,46.910178973912));
#164368=CARTESIAN_POINT('Ctrl Pts',(70.0253013412726,9.30966583385118,46.9632555188312));
#164369=CARTESIAN_POINT('Ctrl Pts',(69.4347663982018,9.23273047198067,47.0785272525984));
#164370=CARTESIAN_POINT('Ctrl Pts',(69.1168088671572,9.17380466130383,47.140510010473));
#164371=CARTESIAN_POINT('Ctrl Pts',(68.575903963802,9.04319115422186,47.2463019625653));
#164372=CARTESIAN_POINT('Ctrl Pts',(68.3513592349754,8.97967774756271,47.2903236630419));
#164373=CARTESIAN_POINT('Ctrl Pts',(67.9596093454733,8.85230258111096,47.367437824625));
#164374=CARTESIAN_POINT('Ctrl Pts',(67.7913921456816,8.79204390546941,47.400654814471));
#164375=CARTESIAN_POINT('Ctrl Pts',(67.5282819835793,8.68890644369087,47.4528063144562));
#164376=CARTESIAN_POINT('Ctrl Pts',(67.4321824434198,8.64931481581403,47.4718966298189));
#164377=CARTESIAN_POINT('Ctrl Pts',(67.2484593626417,8.56989909888166,47.5084791513825));
#164378=CARTESIAN_POINT('Ctrl Pts',(67.1607487912074,8.53031662042858,47.5259822513675));
#164379=CARTESIAN_POINT('Ctrl Pts',(66.9525031809757,8.43232004852205,47.5676323568917));
#164380=CARTESIAN_POINT('Ctrl Pts',(66.8325850799753,8.37261173540689,47.591693032778));
#164381=CARTESIAN_POINT('Ctrl Pts',(66.2763344791619,8.08011881748052,47.7036547071207));
#164382=CARTESIAN_POINT('Ctrl Pts',(65.8577528356841,7.81440369621049,47.7889962894379));
#164383=CARTESIAN_POINT('Ctrl Pts',(65.2779173637126,7.37649729721469,47.9081376415754));
#164384=CARTESIAN_POINT('Ctrl Pts',(65.0988108022077,7.23028613382362,47.9450747958339));
#164385=CARTESIAN_POINT('Ctrl Pts',(64.8167799410034,6.98176966596709,48.0033085362981));
#164386=CARTESIAN_POINT('Ctrl Pts',(64.7105009217701,6.88358146425984,48.0252699974668));
#164387=CARTESIAN_POINT('Ctrl Pts',(64.5591522066784,6.73701687399964,48.0565291608474));
#164388=CARTESIAN_POINT('Ctrl Pts',(64.5122653144452,6.69063021813372,48.0662107561013));
#164389=CARTESIAN_POINT('Ctrl Pts',(64.4268464822436,6.60429739213573,48.0838392412265));
#164390=CARTESIAN_POINT('Ctrl Pts',(64.3881736469449,6.56450220826576,48.0918161896623));
#164391=CARTESIAN_POINT('Ctrl Pts',(64.2916356048183,6.46336087245438,48.1117214535804));
#164392=CARTESIAN_POINT('Ctrl Pts',(64.2342358054794,6.40155819219595,48.1235504136862));
#164393=CARTESIAN_POINT('Ctrl Pts',(63.8681269878283,5.99642266751781,48.1990011178357));
#164394=CARTESIAN_POINT('Ctrl Pts',(63.5841079256245,5.63073787295009,48.2575756279011));
#164395=CARTESIAN_POINT('Ctrl Pts',(63.1825862566011,5.02556877408242,48.3419386339542));
#164396=CARTESIAN_POINT('Ctrl Pts',(63.0462802689799,4.79995372401824,48.3709275079765));
#164397=CARTESIAN_POINT('Ctrl Pts',(62.8280200629741,4.40150236508274,48.4181891275067));
#164398=CARTESIAN_POINT('Ctrl Pts',(62.7415162948175,4.23143661175899,48.4371949525007));
#164399=CARTESIAN_POINT('Ctrl Pts',(62.614828075304,3.96230700734142,48.4655257645866));
#164400=CARTESIAN_POINT('Ctrl Pts',(62.5710588156807,3.86505034155375,48.4754191868442));
#164401=CARTESIAN_POINT('Ctrl Pts',(62.4906832805168,3.67798465926539,48.4938012777463));
#164402=CARTESIAN_POINT('Ctrl Pts',(62.4537927894449,3.58831745171678,48.5023346002953));
#164403=CARTESIAN_POINT('Ctrl Pts',(62.3700525881338,3.3754565605272,48.5219434618219));
#164404=CARTESIAN_POINT('Ctrl Pts',(62.3243884767053,3.25180174801528,48.5328304309446));
#164405=CARTESIAN_POINT('Ctrl Pts',(62.1511607465684,2.75050009199837,48.5749553460674));
#164406=CARTESIAN_POINT('Ctrl Pts',(62.0449873355903,2.36562747392848,48.6027816976324));
#164407=CARTESIAN_POINT('Ctrl Pts',(61.8871778716001,1.60968238304879,48.6485502601413));
#164408=CARTESIAN_POINT('Ctrl Pts',(61.832583123548,1.24001638979765,48.6669726065383));
#164409=CARTESIAN_POINT('Ctrl Pts',(61.788351794091,0.736774046757258,48.6863097536381));
#164410=CARTESIAN_POINT('Ctrl Pts',(61.7795485402972,0.605367799175815,
48.6908333914838));
#164411=CARTESIAN_POINT('Ctrl Pts',(61.7688926641797,0.374627363626792,
48.6978226176743));
#164412=CARTESIAN_POINT('Ctrl Pts',(61.7658631597748,0.275375134965116,
48.7005202239672));
#164413=CARTESIAN_POINT('Ctrl Pts',(61.7635527613475,0.120295156280997,
48.7042392363218));
#164414=CARTESIAN_POINT('Ctrl Pts',(61.7632111060365,0.0644956546494876,
48.7054771489709));
#164415=CARTESIAN_POINT('Ctrl Pts',(61.7633664053386,0.00579618557849801,
48.7066722253423));
#164416=CARTESIAN_POINT('Ctrl Pts',(61.763375392491,0.00289809158621373,
48.7067309535146));
#164417=CARTESIAN_POINT('Ctrl Pts',(61.763385699346,1.76224501330106E-11,
48.7067894065939));
#164418=CARTESIAN_POINT('Origin',(69.6316151486327,0.,39.48523201752));
#164419=CARTESIAN_POINT('',(61.9938354925483,-1.14504475720278E-15,50.0137351291169));
#164420=CARTESIAN_POINT('',(61.9717635125435,4.06541970932136E-10,49.8885587101925));
#164421=CARTESIAN_POINT('',(60.4236626579685,-1.14504475720278E-15,41.1088424787055));
#164422=CARTESIAN_POINT('',(62.2702697977904,2.27382383755812,49.9649923028056));
#164423=CARTESIAN_POINT('Origin',(71.2017879831895,0.,48.390124667801));
#164424=CARTESIAN_POINT('Ctrl Pts',(62.2702697981662,2.2738238374481,49.9649923025089));
#164425=CARTESIAN_POINT('Ctrl Pts',(62.338464173385,2.5537129532415,49.9476325953518));
#164426=CARTESIAN_POINT('Ctrl Pts',(62.4193581571629,2.83019087195468,49.9279210944292));
#164427=CARTESIAN_POINT('Ctrl Pts',(62.5465841826798,3.20128874871533,49.8977784992525));
#164428=CARTESIAN_POINT('Ctrl Pts',(62.5821211470682,3.29959436495245,49.8894317833168));
#164429=CARTESIAN_POINT('Ctrl Pts',(62.6511157296328,3.48097710305096,49.8733500262581));
#164430=CARTESIAN_POINT('Ctrl Pts',(62.6841409394582,3.56421300851538,49.8656989389923));
#164431=CARTESIAN_POINT('Ctrl Pts',(62.755504163825,3.73686226755046,49.8492574290012));
#164432=CARTESIAN_POINT('Ctrl Pts',(62.7940500879524,3.82617414250865,49.8404267614445));
#164433=CARTESIAN_POINT('Ctrl Pts',(62.8891808036111,4.03753497415995,49.8187464730798));
#164434=CARTESIAN_POINT('Ctrl Pts',(62.947003098936,4.15897804528599,49.8056567782711));
#164435=CARTESIAN_POINT('Ctrl Pts',(63.2321092720499,4.72609987004622,49.7415198841712));
#164436=CARTESIAN_POINT('Ctrl Pts',(63.4918566382141,5.15381181483561,49.6841744167643));
#164437=CARTESIAN_POINT('Ctrl Pts',(63.9208794975226,5.74710370347294,49.5915863256821));
#164438=CARTESIAN_POINT('Ctrl Pts',(64.0645491360096,5.93080101248646,49.5608720547424));
#164439=CARTESIAN_POINT('Ctrl Pts',(64.3087335579026,6.21983192977895,49.5092773704718));
#164440=CARTESIAN_POINT('Ctrl Pts',(64.4051332887595,6.32862361521098,49.489048559097));
#164441=CARTESIAN_POINT('Ctrl Pts',(64.5489969220775,6.48344998692467,49.4590988516647));
#164442=CARTESIAN_POINT('Ctrl Pts',(64.5944774738798,6.53135291642221,49.4496638207421));
#164443=CARTESIAN_POINT('Ctrl Pts',(64.6790884449091,6.6185713107172,49.4321766867671));
#164444=CARTESIAN_POINT('Ctrl Pts',(64.7180681183952,6.65803188752871,49.4241459060302));
#164445=CARTESIAN_POINT('Ctrl Pts',(64.8170771088458,6.75646607602476,49.4038076573357));
#164446=CARTESIAN_POINT('Ctrl Pts',(64.8775568608351,6.81496634178852,49.3914379783055));
#164447=CARTESIAN_POINT('Ctrl Pts',(65.2739766207081,7.18802061279423,49.3106599871719));
#164448=CARTESIAN_POINT('Ctrl Pts',(65.6319741136846,7.47747297851757,49.2390543001437));
#164449=CARTESIAN_POINT('Ctrl Pts',(66.2253342827472,7.88763974299578,49.1208693882525));
#164450=CARTESIAN_POINT('Ctrl Pts',(66.4471482466748,8.02728247981476,49.0767924818669));
#164451=CARTESIAN_POINT('Ctrl Pts',(66.8387641224665,8.25091992701465,48.9989475077277));
#164452=CARTESIAN_POINT('Ctrl Pts',(67.0058310877387,8.33955198848845,48.9657312138024));
#164453=CARTESIAN_POINT('Ctrl Pts',(67.2701187057887,8.46938769702591,48.9131318506826));
#164454=CARTESIAN_POINT('Ctrl Pts',(67.3655637187904,8.51423379967032,48.894125768842));
#164455=CARTESIAN_POINT('Ctrl Pts',(67.5490926876763,8.59660126536313,48.8575544299901));
#164456=CARTESIAN_POINT('Ctrl Pts',(67.637037131058,8.63441206673688,48.8400192654076));
#164457=CARTESIAN_POINT('Ctrl Pts',(67.8457260087512,8.72025170403908,48.7983812150223));
#164458=CARTESIAN_POINT('Ctrl Pts',(67.9669197045937,8.76708392344383,48.7741786926102));
#164459=CARTESIAN_POINT('Ctrl Pts',(68.4515197156878,8.94246891885684,48.6773181028156));
#164460=CARTESIAN_POINT('Ctrl Pts',(68.8216910900359,9.05027434378702,48.6031227226294));
#164461=CARTESIAN_POINT('Ctrl Pts',(69.4936031650876,9.2001231144595,48.4683862474918));
#164462=CARTESIAN_POINT('Ctrl Pts',(69.7928416204905,9.25116272674127,48.4083653859328));
#164463=CARTESIAN_POINT('Ctrl Pts',(70.260759596456,9.30682730389654,48.3147748092573));
#164464=CARTESIAN_POINT('Ctrl Pts',(70.427994969166,9.32199066334297,48.2813784943645));
#164465=CARTESIAN_POINT('Ctrl Pts',(70.7123724214733,9.33976898814513,48.2247501463861));
#164466=CARTESIAN_POINT('Ctrl Pts',(70.8293188809134,9.34479204429296,48.2015086019685));
#164467=CARTESIAN_POINT('Ctrl Pts',(71.004804660127,9.34890188244447,48.1667259841301));
#164468=CARTESIAN_POINT('Ctrl Pts',(71.063284755114,9.3497012923494,48.155150247211));
#164469=CARTESIAN_POINT('Ctrl Pts',(71.1726666825065,9.35013038818495,48.1335316537052));
#164470=CARTESIAN_POINT('Ctrl Pts',(71.2235643702529,9.34989843344863,48.1234857745022));
#164471=CARTESIAN_POINT('Ctrl Pts',(71.3513599646629,9.34823232635723,48.0982935985594));
#164472=CARTESIAN_POINT('Ctrl Pts',(71.4282500255082,9.34624452985781,48.0831645726596));
#164473=CARTESIAN_POINT('Ctrl Pts',(71.7790590888718,9.33267699070815,48.0142424997428));
#164474=CARTESIAN_POINT('Ctrl Pts',(72.0524568776137,9.30957845060198,47.9608149724904));
#164475=CARTESIAN_POINT('Ctrl Pts',(72.6447593322961,9.23219685377472,47.8451993336549));
#164476=CARTESIAN_POINT('Ctrl Pts',(72.9626993329413,9.17315626279074,47.783219477862));
#164477=CARTESIAN_POINT('Ctrl Pts',(73.5030081749324,9.04248125187234,47.6775418488351));
#164478=CARTESIAN_POINT('Ctrl Pts',(73.7269880315798,8.97906359442736,47.6336298041711));
#164479=CARTESIAN_POINT('Ctrl Pts',(74.1178978365918,8.85188804666713,47.5566796443309));
#164480=CARTESIAN_POINT('Ctrl Pts',(74.2858331036707,8.79170730222868,47.5235178319677));
#164481=CARTESIAN_POINT('Ctrl Pts',(74.5486161449311,8.68867583872546,47.4714306833254));
#164482=CARTESIAN_POINT('Ctrl Pts',(74.6446653910438,8.64909765603412,47.4523501939351));
#164483=CARTESIAN_POINT('Ctrl Pts',(74.8283549156776,8.56968419609555,47.4157740729919));
#164484=CARTESIAN_POINT('Ctrl Pts',(74.9160813095565,8.53008829951544,47.3982676697056));
#164485=CARTESIAN_POINT('Ctrl Pts',(75.1244679779698,8.43200938396914,47.3565889807507));
#164486=CARTESIAN_POINT('Ctrl Pts',(75.244508817673,8.37222703554004,47.3325033767778));
#164487=CARTESIAN_POINT('Ctrl Pts',(75.7991057103828,8.08052596965006,47.2208727946198));
#164488=CARTESIAN_POINT('Ctrl Pts',(76.2160653638557,7.81596658217665,47.1358655314547));
#164489=CARTESIAN_POINT('Ctrl Pts',(76.7954016041098,7.3789267530892,47.016832730998));
#164490=CARTESIAN_POINT('Ctrl Pts',(76.9753878582457,7.23210630205661,46.9797148608713));
#164491=CARTESIAN_POINT('Ctrl Pts',(77.2585675970679,6.98267226730892,46.9212442501048));
#164492=CARTESIAN_POINT('Ctrl Pts',(77.365153969425,6.88422436874041,46.8992192589907));
#164493=CARTESIAN_POINT('Ctrl Pts',(77.5168444983906,6.73734563515452,46.8678894586805));
#164494=CARTESIAN_POINT('Ctrl Pts',(77.56377759588,6.69091765920212,46.8581983047626));
#164495=CARTESIAN_POINT('Ctrl Pts',(77.6492318037112,6.60455550999448,46.8405624853882));
#164496=CARTESIAN_POINT('Ctrl Pts',(77.6878949222799,6.56477349489488,46.8325875218241));
#164497=CARTESIAN_POINT('Ctrl Pts',(77.7843411152716,6.46373697365865,46.8127011634677));
#164498=CARTESIAN_POINT('Ctrl Pts',(77.8416609785207,6.4020280727773,46.8008886580784));
#164499=CARTESIAN_POINT('Ctrl Pts',(78.2071873852409,5.99760386885256,46.7255579986303));
#164500=CARTESIAN_POINT('Ctrl Pts',(78.4907919707448,5.63261096514926,46.6670697883629));
#164501=CARTESIAN_POINT('Ctrl Pts',(78.8924085685413,5.02774267575176,46.5826944414633));
#164502=CARTESIAN_POINT('Ctrl Pts',(79.029080732912,4.80164468987789,46.5536303315256));
#164503=CARTESIAN_POINT('Ctrl Pts',(79.2478170137369,4.40246070129444,46.506268694393));
#164504=CARTESIAN_POINT('Ctrl Pts',(79.3344599196518,4.23216390971288,46.4872333320305));
#164505=CARTESIAN_POINT('Ctrl Pts',(79.4612973579826,3.96275763087981,46.4588701440984));
#164506=CARTESIAN_POINT('Ctrl Pts',(79.5050899354381,3.86546227061342,46.4489717802639));
#164507=CARTESIAN_POINT('Ctrl Pts',(79.5854860625327,3.67837097280466,46.4305855440169));
#164508=CARTESIAN_POINT('Ctrl Pts',(79.6223755925697,3.58871765375311,46.4220527381548));
#164509=CARTESIAN_POINT('Ctrl Pts',(79.7060833465627,3.37596885746274,46.4024522319571));
#164510=CARTESIAN_POINT('Ctrl Pts',(79.7517196413179,3.25241364226893,46.391572517949));
#164511=CARTESIAN_POINT('Ctrl Pts',(79.9224884864789,2.75835612932782,46.3500488300955));
#164512=CARTESIAN_POINT('Ctrl Pts',(80.027129980208,2.38092459736502,46.3226735320467));
#164513=CARTESIAN_POINT('Ctrl Pts',(80.1719215452331,1.69582363312823,46.2808826249113));
#164514=CARTESIAN_POINT('Ctrl Pts',(80.2209447227862,1.39070876900675,46.2649814678225));
#164515=CARTESIAN_POINT('Ctrl Pts',(80.2738681521203,0.913647685411539,
46.2445656265649));
#164516=CARTESIAN_POINT('Ctrl Pts',(80.288132803381,0.743153784572283,46.2381421771222));
#164517=CARTESIAN_POINT('Ctrl Pts',(80.304532047063,0.453263255336513,46.2287656175665));
#164518=CARTESIAN_POINT('Ctrl Pts',(80.3090306207632,0.334057623561011,
46.2253516693286));
#164519=CARTESIAN_POINT('Ctrl Pts',(80.3124213869859,0.155197929449151,
46.2209140455259));
#164520=CARTESIAN_POINT('Ctrl Pts',(80.3129924750905,0.0955961728885822,
46.2195492289462));
#164521=CARTESIAN_POINT('Ctrl Pts',(80.3130163234586,-0.0158780266130571,
46.2172134153308));
#164522=CARTESIAN_POINT('Ctrl Pts',(80.3126046991915,-0.067746912733556,
46.2162147521974));
#164523=CARTESIAN_POINT('Ctrl Pts',(80.3105092968841,-0.19797558035514,
46.213925863527));
#164524=CARTESIAN_POINT('Ctrl Pts',(80.3082830027052,-0.276324636184175,
46.2127471856332));
#164525=CARTESIAN_POINT('Ctrl Pts',(80.2937134039405,-0.633772313972398,
46.2082512290248));
#164526=CARTESIAN_POINT('Ctrl Pts',(80.2700730893575,-0.912294168723618,
46.2071995336871));
#164527=CARTESIAN_POINT('Ctrl Pts',(80.1919557585515,-1.51567466321251,
46.209796991434));
#164528=CARTESIAN_POINT('Ctrl Pts',(80.1328000113206,-1.83954712985001,
46.2143092903021));
#164529=CARTESIAN_POINT('Ctrl Pts',(80.0023306136439,-2.38999819416391,
46.2269079630008));
#164530=CARTESIAN_POINT('Ctrl Pts',(79.9391208300848,-2.61820054004301,
46.2336352004851));
#164531=CARTESIAN_POINT('Ctrl Pts',(79.8125054852325,-3.01653380177633,
46.2479386877612));
#164532=CARTESIAN_POINT('Ctrl Pts',(79.7526318855361,-3.18767624308534,
46.254945725055));
#164533=CARTESIAN_POINT('Ctrl Pts',(79.6501821527119,-3.45551185792078,
46.2672589687228));
#164534=CARTESIAN_POINT('Ctrl Pts',(79.6108385348436,-3.5534151923753,46.2720518942478));
#164535=CARTESIAN_POINT('Ctrl Pts',(79.5319155756486,-3.74066543713012,
46.2817814396745));
#164536=CARTESIAN_POINT('Ctrl Pts',(79.4925727328799,-3.83009902499393,
46.2866807712271));
#164537=CARTESIAN_POINT('Ctrl Pts',(79.3951400077755,-4.04255726005623,
46.2989262925733));
#164538=CARTESIAN_POINT('Ctrl Pts',(79.3357666809084,-4.16495683091177,
46.3064762468881));
#164539=CARTESIAN_POINT('Ctrl Pts',(79.0461303983591,-4.7305125978204,46.3437067515372));
#164540=CARTESIAN_POINT('Ctrl Pts',(78.7836260362418,-5.15589905359773,
46.378507326741));
#164541=CARTESIAN_POINT('Ctrl Pts',(78.3503391416087,-5.7471037034835,46.4380273062544));
#164542=CARTESIAN_POINT('Ctrl Pts',(78.2048289431449,-5.93080101249349,
46.4583032428461));
#164543=CARTESIAN_POINT('Ctrl Pts',(77.9577242224753,-6.21983192978189,
46.4933360897385));
#164544=CARTESIAN_POINT('Ctrl Pts',(77.8602194457785,-6.32862361521281,
46.5072978747265));
#164545=CARTESIAN_POINT('Ctrl Pts',(77.7147884479232,-6.48344998692486,
46.5283586161441));
#164546=CARTESIAN_POINT('Ctrl Pts',(77.6688237383768,-6.53135291642249,
46.5350478520553));
#164547=CARTESIAN_POINT('Ctrl Pts',(77.5833344811941,-6.61857131071789,
46.5475539777387));
#164548=CARTESIAN_POINT('Ctrl Pts',(77.5439588808796,-6.65803188752971,
46.5533393458536));
#164549=CARTESIAN_POINT('Ctrl Pts',(77.4439647724282,-6.75646607602563,
46.5680907127401));
#164550=CARTESIAN_POINT('Ctrl Pts',(77.3829017163821,-6.81496634178941,
46.5771523100776));
#164551=CARTESIAN_POINT('Ctrl Pts',(76.9827612931862,-7.18802061279908,
46.636829370977));
#164552=CARTESIAN_POINT('Ctrl Pts',(76.621863103432,-7.47747297852509,46.691984389129));
#164553=CARTESIAN_POINT('Ctrl Pts',(76.0238653105896,-7.88763974300305,
46.7838680296034));
#164554=CARTESIAN_POINT('Ctrl Pts',(75.8003531756628,-8.02728247982002,
46.8183141296595));
#164555=CARTESIAN_POINT('Ctrl Pts',(75.4057300777903,-8.25091992701731,
46.8791042998619));
#164556=CARTESIAN_POINT('Ctrl Pts',(75.2373778417391,-8.33955198849032,
46.9050314609777));
#164557=CARTESIAN_POINT('Ctrl Pts',(74.971038675581,-8.46938769702689,46.9459959166003));
#164558=CARTESIAN_POINT('Ctrl Pts',(74.8748492383376,-8.51423379967115,
46.9607801587711));
#164559=CARTESIAN_POINT('Ctrl Pts',(74.6898802860195,-8.59660126536383,
46.9891849457625));
#164560=CARTESIAN_POINT('Ctrl Pts',(74.601242162031,-8.63441206673753,47.0027860521301));
#164561=CARTESIAN_POINT('Ctrl Pts',(74.3908977116618,-8.72025170403977,
47.0350348832982));
#164562=CARTESIAN_POINT('Ctrl Pts',(74.2687351398084,-8.76708392344454,
47.0537426368055));
#164563=CARTESIAN_POINT('Ctrl Pts',(73.7802318125389,-8.94246891886013,
47.1284664205816));
#164564=CARTESIAN_POINT('Ctrl Pts',(73.4070081890647,-9.0502743437919,47.185351635835));
#164565=CARTESIAN_POINT('Ctrl Pts',(72.7295347816975,-9.20012311448153,
47.288548228622));
#164566=CARTESIAN_POINT('Ctrl Pts',(72.4278142695469,-9.2511627267719,47.3344926473394));
#164567=CARTESIAN_POINT('Ctrl Pts',(71.9561053379196,-9.3068273039169,47.4065836462716));
#164568=CARTESIAN_POINT('Ctrl Pts',(71.7875332798937,-9.32199066335528,
47.4323992417412));
#164569=CARTESIAN_POINT('Ctrl Pts',(71.5009378508252,-9.33976898814924,
47.4764488180039));
#164570=CARTESIAN_POINT('Ctrl Pts',(71.3830950495335,-9.34479204429503,
47.4946069550345));
#164571=CARTESIAN_POINT('Ctrl Pts',(71.2062960018439,-9.34890188244507,
47.5219416570739));
#164572=CARTESIAN_POINT('Ctrl Pts',(71.1473835529261,-9.34970129234971,
47.5310653929794));
#164573=CARTESIAN_POINT('Ctrl Pts',(71.0372041684618,-9.35013038818491,
47.5481613826737));
#164574=CARTESIAN_POINT('Ctrl Pts',(70.9859400938251,-9.34989843344841,
47.5561293785756));
#164575=CARTESIAN_POINT('Ctrl Pts',(70.8572352851513,-9.34823232635641,
47.5761651442588));
#164576=CARTESIAN_POINT('Ctrl Pts',(70.7798078307469,-9.34624452985634,
47.5882464598933));
#164577=CARTESIAN_POINT('Ctrl Pts',(70.4265824055313,-9.33267699071156,
47.6434646626661));
#164578=CARTESIAN_POINT('Ctrl Pts',(70.1513992305808,-9.30957845062919,
47.6867667604192));
#164579=CARTESIAN_POINT('Ctrl Pts',(69.5552741074706,-9.23219685386255,
47.78070296817));
#164580=CARTESIAN_POINT('Ctrl Pts',(69.2353098758472,-9.17315626289746,
47.8312028396341));
#164581=CARTESIAN_POINT('Ctrl Pts',(68.6914417661586,-9.04248125198924,
47.9166948590491));
#164582=CARTESIAN_POINT('Ctrl Pts',(68.4659507437593,-8.97906359452854,
47.9520366574021));
#164583=CARTESIAN_POINT('Ctrl Pts',(68.0722971797605,-8.85188804673559,
48.0134261875915));
#164584=CARTESIAN_POINT('Ctrl Pts',(67.9031476406525,-8.7917073022843,48.039701521345));
#164585=CARTESIAN_POINT('Ctrl Pts',(67.6383975018137,-8.68867583876348,
48.0806327055719));
#164586=CARTESIAN_POINT('Ctrl Pts',(67.5416148222849,-8.64909765606977,
48.0955536874141));
#164587=CARTESIAN_POINT('Ctrl Pts',(67.3564933613383,-8.56968419613098,
48.1240088940103));
#164588=CARTESIAN_POINT('Ctrl Pts',(67.2680699738037,-8.5300882995531,48.1375624498331));
#164589=CARTESIAN_POINT('Ctrl Pts',(67.057995608079,-8.43200938402033,48.1696697315726));
#164590=CARTESIAN_POINT('Ctrl Pts',(66.9369563551146,-8.3722270356035,48.1880930524492));
#164591=CARTESIAN_POINT('Ctrl Pts',(66.3776258395292,-8.08052596957712,
48.2728779269175));
#164592=CARTESIAN_POINT('Ctrl Pts',(65.9567377333837,-7.81596658190576,
48.335605829491));
#164593=CARTESIAN_POINT('Ctrl Pts',(65.371628127905,-7.37892675267048,48.4218962492074));
#164594=CARTESIAN_POINT('Ctrl Pts',(65.1898013139434,-7.23210630174306,
48.4485757849636));
#164595=CARTESIAN_POINT('Ctrl Pts',(64.9037012765419,-6.98267226715385,
48.4904845583228));
#164596=CARTESIAN_POINT('Ctrl Pts',(64.7960098583973,-6.88422436862999,
48.5062425230424));
#164597=CARTESIAN_POINT('Ctrl Pts',(64.6427519649519,-6.73734563509782,
48.5286833573295));
#164598=CARTESIAN_POINT('Ctrl Pts',(64.5953347097266,-6.69091765915269,
48.5356287162348));
#164599=CARTESIAN_POINT('Ctrl Pts',(64.5090022157491,-6.60455550995061,
48.5482835273164));
#164600=CARTESIAN_POINT('Ctrl Pts',(64.469943170351,-6.5647734948491,48.5540130782587));
#164601=CARTESIAN_POINT('Ctrl Pts',(64.3725118593432,-6.46373697359551,
48.5683125548094));
#164602=CARTESIAN_POINT('Ctrl Pts',(64.3146086920237,-6.40202807269846,
48.5768169785079));
#164603=CARTESIAN_POINT('Ctrl Pts',(63.9453616218992,-5.99760386866832,
48.6310467077339));
#164604=CARTESIAN_POINT('Ctrl Pts',(63.6588563395619,-5.6326109648648,48.6730842491332));
#164605=CARTESIAN_POINT('Ctrl Pts',(63.2526021180041,-5.0277426754259,48.7311583246122));
#164606=CARTESIAN_POINT('Ctrl Pts',(63.114231782687,-4.80164468962441,48.7505916282126));
#164607=CARTESIAN_POINT('Ctrl Pts',(62.8924882798499,-4.40246070115124,
48.7808984613986));
#164608=CARTESIAN_POINT('Ctrl Pts',(62.8045601031759,-4.23216390960435,
48.7926446909488));
#164609=CARTESIAN_POINT('Ctrl Pts',(62.675671116758,-3.96275763081257,48.8093729713809));
#164610=CARTESIAN_POINT('Ctrl Pts',(62.6311341150639,-3.86546227055174,
48.8150494955452));
#164611=CARTESIAN_POINT('Ctrl Pts',(62.5492980045406,-3.67837097274811,
48.8252691799311));
#164612=CARTESIAN_POINT('Ctrl Pts',(62.5117147938965,-3.58871765369472,
48.8298679275782));
#164613=CARTESIAN_POINT('Ctrl Pts',(62.4263514672228,-3.37596885738771,
48.8400792145593));
#164614=CARTESIAN_POINT('Ctrl Pts',(62.3797462964527,-3.2524136421795,48.845464159663));
#164615=CARTESIAN_POINT('Ctrl Pts',(62.2050741348317,-2.75835612839402,
48.8648510415287));
#164616=CARTESIAN_POINT('Ctrl Pts',(62.0973803917991,-2.38092459556769,
48.8749161746551));
#164617=CARTESIAN_POINT('Ctrl Pts',(61.9470274927069,-1.69582362201107,
48.885167199529));
#164618=CARTESIAN_POINT('Ctrl Pts',(61.8955222575518,-1.39070874928956,
48.8869919137234));
#164619=CARTESIAN_POINT('Ctrl Pts',(61.8388078736529,-0.913647662394935,
48.8859081769848));
#164620=CARTESIAN_POINT('Ctrl Pts',(61.8232065378916,-0.743153766970815,
48.8847509069901));
#164621=CARTESIAN_POINT('Ctrl Pts',(61.8045893182642,-0.4532632457609,48.8815486948721));
#164622=CARTESIAN_POINT('Ctrl Pts',(61.7991944029104,-0.334057616577517,
48.8798792357473));
#164623=CARTESIAN_POINT('Ctrl Pts',(61.7944903683467,-0.155197925530483,
48.8768689437948));
#164624=CARTESIAN_POINT('Ctrl Pts',(61.793486926338,-0.0955961694390742,
48.8757817593667));
#164625=CARTESIAN_POINT('Ctrl Pts',(61.7929593826893,-0.0239936871218512,
48.8743771329385));
#164626=CARTESIAN_POINT('Ctrl Pts',(61.7928938540372,-0.0119968230969001,
48.8741384678195));
#164627=CARTESIAN_POINT('Ctrl Pts',(61.7928511881971,-6.81909623538039E-10,
48.8738964978212));
#164628=CARTESIAN_POINT('Ctrl Pts',(61.763385699346,1.76224501330106E-11,
48.7067894065939));
#164629=CARTESIAN_POINT('Ctrl Pts',(61.7635670284536,-0.0509862958350187,
48.7078177750651));
#164630=CARTESIAN_POINT('Ctrl Pts',(61.7641568264916,-0.101971841470106,
48.7087610001154));
#164631=CARTESIAN_POINT('Ctrl Pts',(61.7669122876853,-0.242658808520474,
48.7111328664627));
#164632=CARTESIAN_POINT('Ctrl Pts',(61.7699345808252,-0.332340962945694,
48.7123858331844));
#164633=CARTESIAN_POINT('Ctrl Pts',(61.7950362740921,-0.857011440140505,
48.7182457033326));
#164634=CARTESIAN_POINT('Ctrl Pts',(61.8456440974283,-1.29015662006303,
48.7171819201477));
#164635=CARTESIAN_POINT('Ctrl Pts',(62.0144667619307,-2.19160907988531,
48.7041015590164));
#164636=CARTESIAN_POINT('Ctrl Pts',(62.139015048218,-2.65742979065379,48.6909733641217));
#164637=CARTESIAN_POINT('Ctrl Pts',(62.3429895304684,-3.23839599178517,
48.6670900963039));
#164638=CARTESIAN_POINT('Ctrl Pts',(62.3902242071645,-3.36426539534811,
48.6614426933651));
#164639=CARTESIAN_POINT('Ctrl Pts',(62.4763353451641,-3.57962734167984,
48.6509673174823));
#164640=CARTESIAN_POINT('Ctrl Pts',(62.5139443805906,-3.66961278424621,
48.6463401683691));
#164641=CARTESIAN_POINT('Ctrl Pts',(62.5953356218942,-3.8561660836585,48.6362240593866));
#164642=CARTESIAN_POINT('Ctrl Pts',(62.6393641644619,-3.95260924435909,
48.630695886835));
#164643=CARTESIAN_POINT('Ctrl Pts',(62.7650028927571,-4.21596093714083,
48.614772990969));
#164644=CARTESIAN_POINT('Ctrl Pts',(62.8499254993405,-4.38120253222522,
48.603851809218));
#164645=CARTESIAN_POINT('Ctrl Pts',(63.0615155416433,-4.76456688989362,
48.5762666886725));
#164646=CARTESIAN_POINT('Ctrl Pts',(63.1921565669718,-4.98028422351736,
48.5589593876354));
#164647=CARTESIAN_POINT('Ctrl Pts',(63.5843067069138,-5.57268493641918,
48.5061130236971));
#164648=CARTESIAN_POINT('Ctrl Pts',(63.8648115235453,-5.93563489524881,
48.4673466811831));
#164649=CARTESIAN_POINT('Ctrl Pts',(64.2367528203933,-6.35031862372333,
48.414052315818));
#164650=CARTESIAN_POINT('Ctrl Pts',(64.3042989974593,-6.42325704918564,
48.4043051116645));
#164651=CARTESIAN_POINT('Ctrl Pts',(64.4131880321295,-6.53714812778854,
48.3884704064834));
#164652=CARTESIAN_POINT('Ctrl Pts',(64.4537852915516,-6.57882545251053,
48.3825408498162));
#164653=CARTESIAN_POINT('Ctrl Pts',(64.5377846410195,-6.66346654316011,
48.3702156956732));
#164654=CARTESIAN_POINT('Ctrl Pts',(64.5812233838699,-6.70638843645338,
48.3638122150543));
#164655=CARTESIAN_POINT('Ctrl Pts',(64.707446729401,-6.82868894044251,48.3451278217));
#164656=CARTESIAN_POINT('Ctrl Pts',(64.7912592997073,-6.90695650860338,
48.3326275253081));
#164657=CARTESIAN_POINT('Ctrl Pts',(64.9959118518596,-7.09112224922956,
48.3019229821779));
#164658=CARTESIAN_POINT('Ctrl Pts',(65.1180664558918,-7.1954584903423,48.2834500157771));
#164659=CARTESIAN_POINT('Ctrl Pts',(65.7139136847808,-7.67825396945095,
48.1928635709965));
#164660=CARTESIAN_POINT('Ctrl Pts',(66.2206166288938,-8.0123958941104,48.1145283069838));
#164661=CARTESIAN_POINT('Ctrl Pts',(66.8797595207667,-8.3593594849516,48.0130437236489));
#164662=CARTESIAN_POINT('Ctrl Pts',(67.0050097002923,-8.42168388641225,
47.9937713297349));
#164663=CARTESIAN_POINT('Ctrl Pts',(67.21909549953,-8.52218497524791,47.9608641819839));
#164664=CARTESIAN_POINT('Ctrl Pts',(67.307212638376,-8.56186688076919,47.9473292384465));
#164665=CARTESIAN_POINT('Ctrl Pts',(67.4902443644734,-8.6408420836707,47.91923842343));
#164666=CARTESIAN_POINT('Ctrl Pts',(67.585224166658,-8.67994727941533,47.9046740078978));
#164667=CARTESIAN_POINT('Ctrl Pts',(67.8383058606871,-8.77921231266517,
47.8659014648516));
#164668=CARTESIAN_POINT('Ctrl Pts',(67.9974311542422,-8.83660130820626,
47.8415598974115));
#164669=CARTESIAN_POINT('Ctrl Pts',(68.3617729545538,-8.95672349711548,
47.7859011176601));
#164670=CARTESIAN_POINT('Ctrl Pts',(68.56777483729,-9.01671267829863,47.754484592589));
#164671=CARTESIAN_POINT('Ctrl Pts',(69.1160892795566,-9.15570560998501,
47.6709302037458));
#164672=CARTESIAN_POINT('Ctrl Pts',(69.4611193349979,-9.22233002612046,
47.6184280673959));
#164673=CARTESIAN_POINT('Ctrl Pts',(70.0925386879095,-9.30695659229467,
47.522031437863));
#164674=CARTESIAN_POINT('Ctrl Pts',(70.3776277853248,-9.33163081763205,
47.478389618091));
#164675=CARTESIAN_POINT('Ctrl Pts',(70.7422775623076,-9.34601401622623,
47.4221618743342));
#164676=CARTESIAN_POINT('Ctrl Pts',(70.8212514525622,-9.34810384537796,
47.4099597963782));
#164677=CARTESIAN_POINT('Ctrl Pts',(70.9512328939819,-9.34985700810057,
47.3898282004054));
#164678=CARTESIAN_POINT('Ctrl Pts',(71.0022312937868,-9.3501177631102,47.3819171730687));
#164679=CARTESIAN_POINT('Ctrl Pts',(71.1112515273485,-9.3497621152038,47.3649769000863));
#164680=CARTESIAN_POINT('Ctrl Pts',(71.1692696581125,-9.34901989622982,
47.3559447580405));
#164681=CARTESIAN_POINT('Ctrl Pts',(71.3403040034562,-9.3452012438635,47.3292754815737));
#164682=CARTESIAN_POINT('Ctrl Pts',(71.4532693916326,-9.34057877345878,
47.3116055248515));
#164683=CARTESIAN_POINT('Ctrl Pts',(71.7249238431665,-9.324403991855,47.2690202023061));
#164684=CARTESIAN_POINT('Ctrl Pts',(71.8834513615109,-9.31079879356123,
47.2440923134608));
#164685=CARTESIAN_POINT('Ctrl Pts',(72.6600239590159,-9.22365320535799,
47.1218122500596));
#164686=CARTESIAN_POINT('Ctrl Pts',(73.2699165952279,-9.09117713409731,
47.0253681320263));
#164687=CARTESIAN_POINT('Ctrl Pts',(74.0274098302864,-8.84367639097596,
46.9072902352787));
#164688=CARTESIAN_POINT('Ctrl Pts',(74.1910500952771,-8.78501521042553,
46.8818801140974));
#164689=CARTESIAN_POINT('Ctrl Pts',(74.4493987748614,-8.68404172740784,
46.8419480918929));
#164690=CARTESIAN_POINT('Ctrl Pts',(74.5451932851291,-8.64472338465233,
46.8271827159251));
#164691=CARTESIAN_POINT('Ctrl Pts',(74.7296923696413,-8.56533134070461,
46.7988287875768));
#164692=CARTESIAN_POINT('Ctrl Pts',(74.8184634640849,-8.52545248653272,
46.785224879625));
#164693=CARTESIAN_POINT('Ctrl Pts',(75.0315229739173,-8.4256518730757,46.752668947513));
#164694=CARTESIAN_POINT('Ctrl Pts',(75.1551476013034,-8.36432319250109,
46.733858365037));
#164695=CARTESIAN_POINT('Ctrl Pts',(75.3538259307227,-8.26014287355754,
46.703754929983));
#164696=CARTESIAN_POINT('Ctrl Pts',(75.4297149566855,-8.21898201114749,
46.6922872222443));
#164697=CARTESIAN_POINT('Ctrl Pts',(75.7197956262946,-8.05634289497177,
46.6485674986653));
#164698=CARTESIAN_POINT('Ctrl Pts',(75.9297731803813,-7.92733080760436,
46.6171676408258));
#164699=CARTESIAN_POINT('Ctrl Pts',(76.5331395579719,-7.52257836313178,
46.5275192108297));
#164700=CARTESIAN_POINT('Ctrl Pts',(76.910829075248,-7.22427425532505,46.4721930274057));
#164701=CARTESIAN_POINT('Ctrl Pts',(77.3306039849859,-6.83621273399556,
46.4107438008237));
#164702=CARTESIAN_POINT('Ctrl Pts',(77.3963266071006,-6.77364568569467,
46.401122980671));
#164703=CARTESIAN_POINT('Ctrl Pts',(77.5011914531659,-6.67084555468564,
46.3857610659146));
#164704=CARTESIAN_POINT('Ctrl Pts',(77.5408987154452,-6.63120875084857,
46.3799414558447));
#164705=CARTESIAN_POINT('Ctrl Pts',(77.6247404834355,-6.54598599595001,
46.3676442855158));
#164706=CARTESIAN_POINT('Ctrl Pts',(77.668772809714,-6.50030227635002,46.3611810819779));
#164707=CARTESIAN_POINT('Ctrl Pts',(77.8002191509532,-6.36110420606446,
46.3418807496631));
#164708=CARTESIAN_POINT('Ctrl Pts',(77.8861885412103,-6.26621859480062,
46.3292494346646));
#164709=CARTESIAN_POINT('Ctrl Pts',(78.223761874539,-5.87785118844521,46.2797081354359));
#164710=CARTESIAN_POINT('Ctrl Pts',(78.4591252799246,-5.57045632262373,
46.2453138001229));
#164711=CARTESIAN_POINT('Ctrl Pts',(78.8944465099846,-4.92259419127054,
46.1830797513794));
#164712=CARTESIAN_POINT('Ctrl Pts',(79.0933171348304,-4.58232243093967,
46.1554242711111));
#164713=CARTESIAN_POINT('Ctrl Pts',(79.3271924237105,-4.11775821695195,
46.1244771651663));
#164714=CARTESIAN_POINT('Ctrl Pts',(79.381650120405,-4.00397454892205,46.1174066260347));
#164715=CARTESIAN_POINT('Ctrl Pts',(79.4738352804155,-3.80104638389385,
46.1056971715342));
#164716=CARTESIAN_POINT('Ctrl Pts',(79.5124966460578,-3.7123575962577,46.1008764184885));
#164717=CARTESIAN_POINT('Ctrl Pts',(79.5917481164606,-3.52267927447631,
46.0911956732692));
#164718=CARTESIAN_POINT('Ctrl Pts',(79.6319721350735,-3.42154870577104,
46.0864064186747));
#164719=CARTESIAN_POINT('Ctrl Pts',(79.7412901033082,-3.13230709027199,
46.0737607030887));
#164720=CARTESIAN_POINT('Ctrl Pts',(79.8061896202673,-2.94264012741909,
46.0667158387936));
#164721=CARTESIAN_POINT('Ctrl Pts',(79.9461141263053,-2.48712880831576,
46.0527074105073));
#164722=CARTESIAN_POINT('Ctrl Pts',(80.015654053396,-2.21976353624555,46.0467862408762));
#164723=CARTESIAN_POINT('Ctrl Pts',(80.1704346911762,-1.4966007572829,46.0366590034094));
#164724=CARTESIAN_POINT('Ctrl Pts',(80.2341508866223,-1.03693003125505,
46.0363702166018));
#164725=CARTESIAN_POINT('Ctrl Pts',(80.271659316106,-0.45496640189662,46.0427778767813));
#164726=CARTESIAN_POINT('Ctrl Pts',(80.2770938096886,-0.335299111565848,
46.0444509800905));
#164727=CARTESIAN_POINT('Ctrl Pts',(80.2818270006704,-0.155893663000213,
46.047468251547));
#164728=CARTESIAN_POINT('Ctrl Pts',(80.2828359808091,-0.0962084642501501,
46.048556351027));
#164729=CARTESIAN_POINT('Ctrl Pts',(80.2836639423684,0.0153215143246354,
46.05074332773));
#164730=CARTESIAN_POINT('Ctrl Pts',(80.2836218605704,0.067162709768048,
46.0518215192948));
#164731=CARTESIAN_POINT('Ctrl Pts',(80.2824460247315,0.197179514697998,
46.0546831336917));
#164732=CARTESIAN_POINT('Ctrl Pts',(80.2807684439539,0.275344499674537,
46.0565466762966));
#164733=CARTESIAN_POINT('Ctrl Pts',(80.2682167320729,0.645856198461007,
46.0660841262589));
#164734=CARTESIAN_POINT('Ctrl Pts',(80.2447462441237,0.937560895303463,
46.0756764433261));
#164735=CARTESIAN_POINT('Ctrl Pts',(80.1289917176439,1.8471016411204,46.1129169547145));
#164736=CARTESIAN_POINT('Ctrl Pts',(79.9891427673429,2.4567852965578,46.1487001419168));
#164737=CARTESIAN_POINT('Ctrl Pts',(79.7447561823636,3.1841200718594,46.2067990040271));
#164738=CARTESIAN_POINT('Ctrl Pts',(79.6957665761307,3.31957855970959,46.2183036590978));
#164739=CARTESIAN_POINT('Ctrl Pts',(79.6083575315831,3.54500672234546,46.2386209024404));
#164740=CARTESIAN_POINT('Ctrl Pts',(79.5715921601552,3.63561892100403,46.2471122455683));
#164741=CARTESIAN_POINT('Ctrl Pts',(79.4934890357583,3.81983480190213,46.2650465287439));
#164742=CARTESIAN_POINT('Ctrl Pts',(79.452023179409,3.91336737654442,46.2745141836652));
#164743=CARTESIAN_POINT('Ctrl Pts',(79.3395131363372,4.15638208589489,46.3000677296836));
#164744=CARTESIAN_POINT('Ctrl Pts',(79.2660535538036,4.30465598284,46.3166219564862));
#164745=CARTESIAN_POINT('Ctrl Pts',(79.0899349566932,4.63772012676089,46.3560171971819));
#164746=CARTESIAN_POINT('Ctrl Pts',(78.9848908265478,4.82109118340806,46.3793148004863));
#164747=CARTESIAN_POINT('Ctrl Pts',(78.6998728894683,5.28173156896326,46.4419682649492));
#164748=CARTESIAN_POINT('Ctrl Pts',(78.511324158854,5.55312666615649,46.4829148477562));
#164749=CARTESIAN_POINT('Ctrl Pts',(78.1620088578202,6.0027713619865,46.5576018043202));
#164750=CARTESIAN_POINT('Ctrl Pts',(78.0079285758451,6.18599058892275,46.5902093544676));
#164751=CARTESIAN_POINT('Ctrl Pts',(77.7936558180712,6.42156307501393,46.6349717577744));
#164752=CARTESIAN_POINT('Ctrl Pts',(77.7395648308506,6.47951189241012,46.6462252570751));
#164753=CARTESIAN_POINT('Ctrl Pts',(77.6467453452615,6.57641319025066,46.6654505844092));
#164754=CARTESIAN_POINT('Ctrl Pts',(77.6083987518249,6.61573549341447,46.6733688934481));
#164755=CARTESIAN_POINT('Ctrl Pts',(77.5211511102418,6.70361501719139,46.6913294666023));
#164756=CARTESIAN_POINT('Ctrl Pts',(77.4720552892529,6.75196734058799,46.7013986614867));
#164757=CARTESIAN_POINT('Ctrl Pts',(77.303415959847,6.9143611577255,46.7358721502811));
#164758=CARTESIAN_POINT('Ctrl Pts',(77.1813821199958,7.02569437679335,46.7606292502846));
#164759=CARTESIAN_POINT('Ctrl Pts',(76.8360214369066,7.32412590745934,46.8303198927398));
#164760=CARTESIAN_POINT('Ctrl Pts',(76.606798350837,7.5038831615887,46.8761682380887));
#164761=CARTESIAN_POINT('Ctrl Pts',(76.0463337726893,7.90184595470696,46.9878920041969));
#164762=CARTESIAN_POINT('Ctrl Pts',(75.7088465631406,8.10991443379385,47.0548913170773));
#164763=CARTESIAN_POINT('Ctrl Pts',(75.2367218954305,8.36020400012083,47.1487793658631));
#164764=CARTESIAN_POINT('Ctrl Pts',(75.1127163161697,8.42235767890001,47.1734512387016));
#164765=CARTESIAN_POINT('Ctrl Pts',(74.9006151022461,8.52266886312546,47.2156850673618));
#164766=CARTESIAN_POINT('Ctrl Pts',(74.8132228671696,8.56231946092364,47.2330963292774));
#164767=CARTESIAN_POINT('Ctrl Pts',(74.6315707577106,8.64129160482401,47.2693104563464));
#164768=CARTESIAN_POINT('Ctrl Pts',(74.5372448790734,8.68042064155764,47.2881279924881));
#164769=CARTESIAN_POINT('Ctrl Pts',(74.2855688325895,8.77987820004276,47.3383720629451));
#164770=CARTESIAN_POINT('Ctrl Pts',(74.1272027197919,8.83741098068447,47.3700251659421));
#164771=CARTESIAN_POINT('Ctrl Pts',(73.6842697534294,8.98447133026994,47.4586482778382));
#164772=CARTESIAN_POINT('Ctrl Pts',(73.3968578410585,9.06435450313553,47.5162634325406));
#164773=CARTESIAN_POINT('Ctrl Pts',(72.588628063085,9.24642150572165,47.6783341370818));
#164774=CARTESIAN_POINT('Ctrl Pts',(72.0621839683428,9.31703470328471,47.7839968533797));
#164775=CARTESIAN_POINT('Ctrl Pts',(71.4462111432439,9.34477529788262,47.9064224007076));
#164776=CARTESIAN_POINT('Ctrl Pts',(71.3598304288511,9.34741946180787,47.9235617906978));
#164777=CARTESIAN_POINT('Ctrl Pts',(71.2260315324177,9.34958686887705,47.95005489349));
#164778=CARTESIAN_POINT('Ctrl Pts',(71.1786365410979,9.34998023070964,47.9594287712936));
#164779=CARTESIAN_POINT('Ctrl Pts',(71.077870729738,9.35002071453647,47.9793334044545));
#164780=CARTESIAN_POINT('Ctrl Pts',(71.0245010799648,9.34956760886984,47.9898607001912));
#164781=CARTESIAN_POINT('Ctrl Pts',(70.880606384687,9.34706638420263,48.0182088608707));
#164782=CARTESIAN_POINT('Ctrl Pts',(70.7900975252442,9.34412735863316,48.0360018900547));
#164783=CARTESIAN_POINT('Ctrl Pts',(70.3982657166123,9.32548577265104,48.1129063480163));
#164784=CARTESIAN_POINT('Ctrl Pts',(70.0977095135343,9.29601287225383,48.1715796033842));
#164785=CARTESIAN_POINT('Ctrl Pts',(69.2142188657888,9.16433907346765,48.3439768441029));
#164786=CARTESIAN_POINT('Ctrl Pts',(68.6389457528607,9.01980846731191,48.4562179985451));
#164787=CARTESIAN_POINT('Ctrl Pts',(67.9559191568667,8.77488452073174,48.5911161960689));
#164788=CARTESIAN_POINT('Ctrl Pts',(67.8312720941397,8.72705065872341,48.6157987874264));
#164789=CARTESIAN_POINT('Ctrl Pts',(67.6186834530462,8.64002832520788,48.6580182804227));
#164790=CARTESIAN_POINT('Ctrl Pts',(67.5302361831385,8.60216721727257,48.675620924733));
#164791=CARTESIAN_POINT('Ctrl Pts',(67.3474664984434,8.52046298533827,48.7120758426276));
#164792=CARTESIAN_POINT('Ctrl Pts',(67.2532590537562,8.47638961103273,48.7309117291574));
#164793=CARTESIAN_POINT('Ctrl Pts',(66.9977112251717,8.35143644758021,48.7821316084636));
#164794=CARTESIAN_POINT('Ctrl Pts',(66.8379561619777,8.26733248382455,48.8142914856332));
#164795=CARTESIAN_POINT('Ctrl Pts',(66.4690842617132,8.05887909828604,48.888860198392));
#164796=CARTESIAN_POINT('Ctrl Pts',(66.2621865760908,7.93076334932215,48.9309316614686));
#164797=CARTESIAN_POINT('Ctrl Pts',(65.6619146421346,7.52498492960308,49.0535781095235));
#164798=CARTESIAN_POINT('Ctrl Pts',(65.2847154445787,7.22410189965589,49.1314630440248));
#164799=CARTESIAN_POINT('Ctrl Pts',(64.866939956944,6.83349025458365,49.2177660955589));
#164800=CARTESIAN_POINT('Ctrl Pts',(64.8024995487228,6.7714617167852,49.2310779803241));
#164801=CARTESIAN_POINT('Ctrl Pts',(64.6993994913589,6.66929862117474,49.2523647504695));
#164802=CARTESIAN_POINT('Ctrl Pts',(64.6601965021077,6.62974462839217,49.2604560330086));
#164803=CARTESIAN_POINT('Ctrl Pts',(64.5771015214369,6.5443800044087,49.2775972288615));
#164804=CARTESIAN_POINT('Ctrl Pts',(64.533316503704,6.49846556657053,49.2866243942788));
#164805=CARTESIAN_POINT('Ctrl Pts',(64.4018221984846,6.3577113626466,49.3137283439525));
#164806=CARTESIAN_POINT('Ctrl Pts',(64.3155898362575,6.26145426016034,49.3314942582238));
#164807=CARTESIAN_POINT('Ctrl Pts',(63.9788741076746,5.86942007725401,49.4009272629691));
#164808=CARTESIAN_POINT('Ctrl Pts',(63.7447236835192,5.55957819783879,49.4493659168226));
#164809=CARTESIAN_POINT('Ctrl Pts',(63.3171227674431,4.91342939294318,49.5392371581422));
#164810=CARTESIAN_POINT('Ctrl Pts',(63.1238939789041,4.57790060375784,49.5806184944906));
#164811=CARTESIAN_POINT('Ctrl Pts',(62.8959726140578,4.11833577497276,49.6309876735791));
#164812=CARTESIAN_POINT('Ctrl Pts',(62.842333499432,4.00447026933959,49.6429792921954));
#164813=CARTESIAN_POINT('Ctrl Pts',(62.7516504306612,3.80145085382702,49.6635164143211));
#164814=CARTESIAN_POINT('Ctrl Pts',(62.7136635844201,3.71275418739621,49.672210954206));
#164815=CARTESIAN_POINT('Ctrl Pts',(62.6358873208469,3.52311655419153,49.6902174456147));
#164816=CARTESIAN_POINT('Ctrl Pts',(62.5964641786824,3.42203534210194,49.6994709655434));
#164817=CARTESIAN_POINT('Ctrl Pts',(62.489517734195,3.13312860802896,49.7249506785699));
#164818=CARTESIAN_POINT('Ctrl Pts',(62.426197133163,2.94375289465577,49.7405075524241));
#164819=CARTESIAN_POINT('Ctrl Pts',(62.2901216825293,2.48917447324313,49.7751430550551));
#164820=CARTESIAN_POINT('Ctrl Pts',(62.2228407528162,2.22246015261924,49.7933312560388));
#164821=CARTESIAN_POINT('Ctrl Pts',(62.0743447524768,1.5026287611099,49.8366007825257));
#164822=CARTESIAN_POINT('Ctrl Pts',(62.0143626435984,1.04569009449929,49.8580589365739));
#164823=CARTESIAN_POINT('Ctrl Pts',(61.9806176086439,0.463993601198438,
49.8770388888381));
#164824=CARTESIAN_POINT('Ctrl Pts',(61.9758895286163,0.341859245624509,
49.880560727444));
#164825=CARTESIAN_POINT('Ctrl Pts',(61.9723400736211,0.159540919171869,
49.8851031453375));
#164826=CARTESIAN_POINT('Ctrl Pts',(61.9717382329125,0.0994134776165123,
49.8864852986239));
#164827=CARTESIAN_POINT('Ctrl Pts',(61.971697316922,0.0261879178999035,
49.8880248982242));
#164828=CARTESIAN_POINT('Ctrl Pts',(61.9717169449031,0.013093935805121,
49.8882946119736));
#164829=CARTESIAN_POINT('Ctrl Pts',(61.9717635125435,8.13085086909029E-10,
49.8885587101925));
#164830=CARTESIAN_POINT('Origin',(73.0915550886457,-4.33680868994202E-16,
59.1075264962884));
#164831=CARTESIAN_POINT('',(82.3304102850288,-3.3346522467903E-11,56.7953584157516));
#164832=CARTESIAN_POINT('',(82.3383045685277,3.32536544680013E-11,56.8401291222381));
#164833=CARTESIAN_POINT('',(82.4472287422617,-1.59709532818419E-15,57.4578688084528));
#164834=CARTESIAN_POINT('',(64.0263520775732,-2.56296981511824,60.375952723877));
#164835=CARTESIAN_POINT('Ctrl Pts',(82.3304102850288,-6.66914478404779E-11,
56.7953584157516));
#164836=CARTESIAN_POINT('Ctrl Pts',(82.3304361494038,0.0136416783697664,
56.7955050999108));
#164837=CARTESIAN_POINT('Ctrl Pts',(82.3304329016124,0.0272833261406265,
56.7956558928931));
#164838=CARTESIAN_POINT('Ctrl Pts',(82.3303332321314,0.0693062246595365,
56.7961331583724));
#164839=CARTESIAN_POINT('Ctrl Pts',(82.3301399285843,0.0976868818918377,
56.796473400641));
#164840=CARTESIAN_POINT('Ctrl Pts',(82.3291325800309,0.187235805179669,
56.797604330781));
#164841=CARTESIAN_POINT('Ctrl Pts',(82.3278593968084,0.248396495000157,
56.7984612196501));
#164842=CARTESIAN_POINT('Ctrl Pts',(82.3181493776529,0.56799719273704,56.803394263009));
#164843=CARTESIAN_POINT('Ctrl Pts',(82.2998583057858,0.826005740413701,
56.8089357541939));
#164844=CARTESIAN_POINT('Ctrl Pts',(82.2031651117969,1.69300374792058,56.8334372425269));
#164845=CARTESIAN_POINT('Ctrl Pts',(82.0769427770516,2.29486224576347,56.8604095822293));
#164846=CARTESIAN_POINT('Ctrl Pts',(81.8356818752499,3.06905569972808,56.9105339377435));
#164847=CARTESIAN_POINT('Ctrl Pts',(81.7709902057922,3.25611438548073,56.9238851129339));
#164848=CARTESIAN_POINT('Ctrl Pts',(81.6762616274636,3.50488392340241,56.9433545301387));
#164849=CARTESIAN_POINT('Ctrl Pts',(81.6512449214178,3.56852828973571,56.9484894233616));
#164850=CARTESIAN_POINT('Ctrl Pts',(81.6088238179609,3.67315344280506,56.957186510578));
#164851=CARTESIAN_POINT('Ctrl Pts',(81.5918081416092,3.7142953613545,56.9606724714772));
#164852=CARTESIAN_POINT('Ctrl Pts',(81.5579566751273,3.79455773772598,56.9676027154383));
#164853=CARTESIAN_POINT('Ctrl Pts',(81.5411453064278,3.83368776072029,56.9710422037177));
#164854=CARTESIAN_POINT('Ctrl Pts',(81.5005809897616,3.92639702160487,56.9793361941018));
#164855=CARTESIAN_POINT('Ctrl Pts',(81.4765977448985,3.97986950870148,56.9842358674312));
#164856=CARTESIAN_POINT('Ctrl Pts',(81.3927236818395,4.16237034545123,57.001356961738));
#164857=CARTESIAN_POINT('Ctrl Pts',(81.3304666362066,4.29024605885254,57.0140421095172));
#164858=CARTESIAN_POINT('Ctrl Pts',(81.1698559134361,4.60226073224271,57.0467004299358));
#164859=CARTESIAN_POINT('Ctrl Pts',(81.0683017501658,4.78460127400127,57.0672953529085));
#164860=CARTESIAN_POINT('Ctrl Pts',(80.8119075485792,5.21136267709586,57.1190883190135));
#164861=CARTESIAN_POINT('Ctrl Pts',(80.6517985477197,5.45225106828773,57.1512790088409));
#164862=CARTESIAN_POINT('Ctrl Pts',(80.2803543201951,5.95917071584238,57.2253168712518));
#164863=CARTESIAN_POINT('Ctrl Pts',(80.0652284539025,6.22183124387477,57.2678150177474));
#164864=CARTESIAN_POINT('Ctrl Pts',(79.7910851622844,6.52186675418303,57.32110834585));
#164865=CARTESIAN_POINT('Ctrl Pts',(79.7450868029703,6.57113337166121,57.3300232694491));
#164866=CARTESIAN_POINT('Ctrl Pts',(79.6776116524779,6.64185875188562,57.3430568631205));
#164867=CARTESIAN_POINT('Ctrl Pts',(79.6565501373063,6.66372117959855,57.3471190818423));
#164868=CARTESIAN_POINT('Ctrl Pts',(79.6190475064207,6.70227325175643,57.3543411398114));
#164869=CARTESIAN_POINT('Ctrl Pts',(79.6026488522168,6.71900476719854,57.3574953250551));
#164870=CARTESIAN_POINT('Ctrl Pts',(79.5668198937393,6.75528768582968,57.3643784980096));
#164871=CARTESIAN_POINT('Ctrl Pts',(79.5473661473527,6.77481474216961,57.3681105873054));
#164872=CARTESIAN_POINT('Ctrl Pts',(79.4913568429418,6.8305409954225,57.3788415117707));
#164873=CARTESIAN_POINT('Ctrl Pts',(79.4545915323723,6.86652253971348,57.3858683370367));
#164874=CARTESIAN_POINT('Ctrl Pts',(79.1320123415624,7.17706352077828,57.4473881700254));
#164875=CARTESIAN_POINT('Ctrl Pts',(78.8295625835376,7.4333033625233,57.504180328059));
#164876=CARTESIAN_POINT('Ctrl Pts',(78.0897705792893,7.98344927222312,57.6426411375825));
#164877=CARTESIAN_POINT('Ctrl Pts',(77.6421906136065,8.26086009995398,57.7261220861622));
#164878=CARTESIAN_POINT('Ctrl Pts',(77.0952892025317,8.53880775881918,57.8288291045846));
#164879=CARTESIAN_POINT('Ctrl Pts',(77.0157871421151,8.57779082465693,57.8437738246327));
#164880=CARTESIAN_POINT('Ctrl Pts',(76.8876775618437,8.63834843166178,57.8678814549624));
#164881=CARTESIAN_POINT('Ctrl Pts',(76.8394099992647,8.66065846833518,57.8769701791974));
#164882=CARTESIAN_POINT('Ctrl Pts',(76.753133545694,8.69963913021958,57.8932265835412));
#164883=CARTESIAN_POINT('Ctrl Pts',(76.7151970925453,8.71647313777519,57.9003782859248));
#164884=CARTESIAN_POINT('Ctrl Pts',(76.6354165165366,8.7512351300743,57.9154261194031));
#164885=CARTESIAN_POINT('Ctrl Pts',(76.5935514800197,8.76911030138037,57.9233269469683));
#164886=CARTESIAN_POINT('Ctrl Pts',(76.482689803225,8.81548107329893,57.9442607664512));
#164887=CARTESIAN_POINT('Ctrl Pts',(76.4134848353773,8.84344856394623,57.9573406795673));
#164888=CARTESIAN_POINT('Ctrl Pts',(76.0683221564028,8.97809932576191,58.0226366693852));
#164889=CARTESIAN_POINT('Ctrl Pts',(75.7878639833882,9.07226092402586,58.0758864692123));
#164890=CARTESIAN_POINT('Ctrl Pts',(75.1696910987616,9.24722340595707,58.1935417090461));
#164891=CARTESIAN_POINT('Ctrl Pts',(74.8309858927555,9.32271167789953,58.2581874850533));
#164892=CARTESIAN_POINT('Ctrl Pts',(74.1085416052176,9.44129043426658,58.395918866406));
#164893=CARTESIAN_POINT('Ctrl Pts',(73.72469710605,9.47968808535207,58.4690073968196));
#164894=CARTESIAN_POINT('Ctrl Pts',(73.2721228765592,9.49629949493761,58.5544269878978));
#164895=CARTESIAN_POINT('Ctrl Pts',(73.2047059216205,9.49802993182143,58.5671312946173));
#164896=CARTESIAN_POINT('Ctrl Pts',(73.1109590975419,9.49940219306647,58.5847645326172));
#164897=CARTESIAN_POINT('Ctrl Pts',(73.0846438274134,9.49967417410826,58.5897106939471));
#164898=CARTESIAN_POINT('Ctrl Pts',(73.0366422277101,9.4999637943183,58.5987260355958));
#164899=CARTESIAN_POINT('Ctrl Pts',(73.0149564637516,9.50001777310221,58.6027963254881));
#164900=CARTESIAN_POINT('Ctrl Pts',(72.9698124696333,9.49997013946072,58.6112639834575));
#164901=CARTESIAN_POINT('Ctrl Pts',(72.9463544361966,9.49985545870626,58.6156608886584));
#164902=CARTESIAN_POINT('Ctrl Pts',(72.8843071099303,9.49931425884716,58.6272830451364));
#164903=CARTESIAN_POINT('Ctrl Pts',(72.8457186540859,9.49873431091007,58.634503100477));
#164904=CARTESIAN_POINT('Ctrl Pts',(72.6637228623521,9.49485114654243,58.6685209405539));
#164905=CARTESIAN_POINT('Ctrl Pts',(72.5203824559727,9.48843043595795,58.6952132140827));
#164906=CARTESIAN_POINT('Ctrl Pts',(72.088324422784,9.45892269382461,58.775473376981));
#164907=CARTESIAN_POINT('Ctrl Pts',(71.8004277725095,9.42553847742185,58.8286929365271));
#164908=CARTESIAN_POINT('Ctrl Pts',(70.9294339256922,9.28257215559893,58.9896690517043));
#164909=CARTESIAN_POINT('Ctrl Pts',(70.3546630487159,9.1301344367234,59.0959441166322));
#164910=CARTESIAN_POINT('Ctrl Pts',(69.7026687788365,8.88786067093953,59.2179772337934));
#164911=CARTESIAN_POINT('Ctrl Pts',(69.6077254164951,8.85077925764338,59.2357827832967));
#164912=CARTESIAN_POINT('Ctrl Pts',(69.4654057904454,8.79245932474628,59.2625293803556));
#164913=CARTESIAN_POINT('Ctrl Pts',(69.4175719163595,8.77238542969545,59.2715286399817));
#164914=CARTESIAN_POINT('Ctrl Pts',(69.3320019318184,8.73562417644508,59.2876450707456));
#164915=CARTESIAN_POINT('Ctrl Pts',(69.2942049269219,8.71908556271438,59.2947700795849));
#164916=CARTESIAN_POINT('Ctrl Pts',(69.2138103170834,8.68326417066188,59.3099384454211));
#164917=CARTESIAN_POINT('Ctrl Pts',(69.1712450524896,8.66390982151452,59.3179774919062));
#164918=CARTESIAN_POINT('Ctrl Pts',(69.0558598267407,8.61038392558845,59.3397916328093));
#164919=CARTESIAN_POINT('Ctrl Pts',(68.9833300901668,8.57558076856505,59.3535278008311));
#164920=CARTESIAN_POINT('Ctrl Pts',(68.5016419032388,8.33666294959657,59.4449115638139));
#164921=CARTESIAN_POINT('Ctrl Pts',(68.1073425803984,8.10324525509951,59.5205274318316));
#164922=CARTESIAN_POINT('Ctrl Pts',(67.3394430470525,7.56843792402817,59.668707780197));
#164923=CARTESIAN_POINT('Ctrl Pts',(66.9685695399479,7.26534081608214,59.7407822468252));
#164924=CARTESIAN_POINT('Ctrl Pts',(66.5776529437535,6.89261966482319,59.8162633882389));
#164925=CARTESIAN_POINT('Ctrl Pts',(66.5338127155536,6.84999734922753,59.8247202492948));
#164926=CARTESIAN_POINT('Ctrl Pts',(66.4694231049319,6.78616625869486,59.8371252345835));
#164927=CARTESIAN_POINT('Ctrl Pts',(66.4485602686789,6.7652893266537,59.8411420452457));
#164928=CARTESIAN_POINT('Ctrl Pts',(66.4113734985588,6.72772661838726,59.848296722624));
#164929=CARTESIAN_POINT('Ctrl Pts',(66.3950137437656,6.71107843117556,59.851442508499));
#164930=CARTESIAN_POINT('Ctrl Pts',(66.3587260892882,6.67387605473532,59.858416132229));
#164931=CARTESIAN_POINT('Ctrl Pts',(66.3388291033348,6.65329108414286,59.8622371672081));
#164932=CARTESIAN_POINT('Ctrl Pts',(66.2798530486098,6.59171792780605,59.8735557732884));
#164933=CARTESIAN_POINT('Ctrl Pts',(66.2410432714808,6.55046284603278,59.8809945845597));
#164934=CARTESIAN_POINT('Ctrl Pts',(66.1517045392773,6.45376725075649,59.898101171084));
#164935=CARTESIAN_POINT('Ctrl Pts',(66.1014546419472,6.39806376855125,59.9077098654265));
#164936=CARTESIAN_POINT('Ctrl Pts',(65.9269553932567,6.19993432325553,59.9410474258483));
#164937=CARTESIAN_POINT('Ctrl Pts',(65.8062572280701,6.0543205221251,59.9640525752478));
#164938=CARTESIAN_POINT('Ctrl Pts',(65.2845398860281,5.385053608281,60.0635606843777));
#164939=CARTESIAN_POINT('Ctrl Pts',(64.9338534711927,4.82315064312234,60.1307897232555));
#164940=CARTESIAN_POINT('Ctrl Pts',(64.6062546085833,4.15128264631376,60.1961459212992));
#164941=CARTESIAN_POINT('Ctrl Pts',(64.5695833887254,4.07341224577026,60.2035053404558));
#164942=CARTESIAN_POINT('Ctrl Pts',(64.5118915531841,3.94646975045704,60.2151582713883));
#164943=CARTESIAN_POINT('Ctrl Pts',(64.4902225432207,3.89770722079457,60.2195533944051));
#164944=CARTESIAN_POINT('Ctrl Pts',(64.4523015675538,3.81040424880979,60.2272785808646));
#164945=CARTESIAN_POINT('Ctrl Pts',(64.435892377755,3.77193584703927,60.2306332448688));
#164946=CARTESIAN_POINT('Ctrl Pts',(64.4016743780867,3.69023283095837,60.2376542853273));
#164947=CARTESIAN_POINT('Ctrl Pts',(64.3839290387559,3.6469719951683,60.2413107011729));
#164948=CARTESIAN_POINT('Ctrl Pts',(64.3371378072118,3.53046917569309,60.2509940480175));
#164949=CARTESIAN_POINT('Ctrl Pts',(64.3086771423989,3.45698858947454,60.2569292079204));
#164950=CARTESIAN_POINT('Ctrl Pts',(64.1578442276479,3.05277718437291,60.2886391438428));
#164951=CARTESIAN_POINT('Ctrl Pts',(64.0528856605776,2.71563461648298,60.3116835047421));
#164952=CARTESIAN_POINT('Ctrl Pts',(63.8903311078625,2.06981831953089,60.3493259349052));
#164953=CARTESIAN_POINT('Ctrl Pts',(63.8288103430972,1.76265196805594,60.3645597711951));
#164954=CARTESIAN_POINT('Ctrl Pts',(63.7272171137977,1.08540318133264,60.3919795022382));
#164955=CARTESIAN_POINT('Ctrl Pts',(63.6933763552644,0.71485472970121,60.4030443918243));
#164956=CARTESIAN_POINT('Ctrl Pts',(63.6786693728875,0.276017243088358,
60.4109924405149));
#164957=CARTESIAN_POINT('Ctrl Pts',(63.6771170195282,0.208815160069549,
60.4120669629704));
#164958=CARTESIAN_POINT('Ctrl Pts',(63.6759158954637,0.11423774835206,60.4133741165184));
#164959=CARTESIAN_POINT('Ctrl Pts',(63.6756841947258,0.0868734877545023,
60.4137281666744));
#164960=CARTESIAN_POINT('Ctrl Pts',(63.675474176648,0.0372991303843346,
60.4143254323333));
#164961=CARTESIAN_POINT('Ctrl Pts',(63.6754563435343,0.0150894428150445,
60.4145769581556));
#164962=CARTESIAN_POINT('Ctrl Pts',(63.6755767889806,-0.0307133606495606,
60.4150623408448));
#164963=CARTESIAN_POINT('Ctrl Pts',(63.6757248626156,-0.054306235738305,
60.4152941428821));
#164964=CARTESIAN_POINT('Ctrl Pts',(63.6763363450625,-0.115922537478582,
60.4158523503208));
#164965=CARTESIAN_POINT('Ctrl Pts',(63.676937235388,-0.153944434876264,
60.4161498820628));
#164966=CARTESIAN_POINT('Ctrl Pts',(63.6806354159257,-0.324465369262825,
60.4172766147717));
#164967=CARTESIAN_POINT('Ctrl Pts',(63.6862250977111,-0.456898873532166,
60.4175894071281));
#164968=CARTESIAN_POINT('Ctrl Pts',(63.7102807695795,-0.839965672217378,
60.4169396754294));
#164969=CARTESIAN_POINT('Ctrl Pts',(63.7357871571807,-1.09004065012715,
60.4145855794763));
#164970=CARTESIAN_POINT('Ctrl Pts',(63.8295460682105,-1.7520747728875,60.4036167386114));
#164971=CARTESIAN_POINT('Ctrl Pts',(63.9148127385724,-2.16101571447035,
60.3919202724443));
#164972=CARTESIAN_POINT('Ctrl Pts',(64.0263520775732,-2.56296981511824,
60.3759527238769));
#164973=CARTESIAN_POINT('',(64.0263520775731,2.56296981511791,60.375952723877));
#164974=CARTESIAN_POINT('Origin',(73.035119430904,-4.33680868994202E-16,
58.7874639765594));
#164975=CARTESIAN_POINT('Ctrl Pts',(64.0263520775731,2.56296981511784,60.375952723877));
#164976=CARTESIAN_POINT('Ctrl Pts',(64.1026158838864,2.84095531252864,60.3599465983121));
#164977=CARTESIAN_POINT('Ctrl Pts',(64.1912865984287,3.11523407478812,60.3415890269741));
#164978=CARTESIAN_POINT('Ctrl Pts',(64.3121166968048,3.43859313024599,60.316734836422));
#164979=CARTESIAN_POINT('Ctrl Pts',(64.3326292944016,3.49202629145127,60.3125204147557));
#164980=CARTESIAN_POINT('Ctrl Pts',(64.3691319167927,3.58462893357413,60.3050286346985));
#164981=CARTESIAN_POINT('Ctrl Pts',(64.384906673452,3.62388487384467,60.301793453566));
#164982=CARTESIAN_POINT('Ctrl Pts',(64.4171374354681,3.7025840307606,60.2951880246446));
#164983=CARTESIAN_POINT('Ctrl Pts',(64.4335984321683,3.7420240586799,60.2918168012444));
#164984=CARTESIAN_POINT('Ctrl Pts',(64.465605139931,3.81729204540382,60.2852661135502));
#164985=CARTESIAN_POINT('Ctrl Pts',(64.4811075118149,3.85313821728493,60.2820951550674));
#164986=CARTESIAN_POINT('Ctrl Pts',(64.5180810162231,3.93721827309926,60.2745366457046));
#164987=CARTESIAN_POINT('Ctrl Pts',(64.5397313429847,3.98536875392491,60.2701139508762));
#164988=CARTESIAN_POINT('Ctrl Pts',(64.6170383069826,4.15356906086304,60.2543334243197));
#164989=CARTESIAN_POINT('Ctrl Pts',(64.6747690233333,4.27261015339433,60.2425691636302));
#164990=CARTESIAN_POINT('Ctrl Pts',(64.8752502372591,4.66505394318771,60.2017924666812));
#164991=CARTESIAN_POINT('Ctrl Pts',(65.0286720176914,4.93256295969039,60.170701227291));
#164992=CARTESIAN_POINT('Ctrl Pts',(65.3784084299162,5.47906277106085,60.1002996592275));
#164993=CARTESIAN_POINT('Ctrl Pts',(65.5772991147117,5.75582346692115,60.060516620384));
#164994=CARTESIAN_POINT('Ctrl Pts',(65.8887249983978,6.14316301175874,59.9989998770026));
#164995=CARTESIAN_POINT('Ctrl Pts',(65.9899248847189,6.26279640139174,59.9791166211805));
#164996=CARTESIAN_POINT('Ctrl Pts',(66.1381820222008,6.42943037394125,59.9501891836551));
#164997=CARTESIAN_POINT('Ctrl Pts',(66.1828536172576,6.47857968011895,59.9414977986718));
#164998=CARTESIAN_POINT('Ctrl Pts',(66.2631268857357,6.56503777276278,59.925928732616));
#164999=CARTESIAN_POINT('Ctrl Pts',(66.2985243072835,6.60253766253368,59.9190798382392));
#165000=CARTESIAN_POINT('Ctrl Pts',(66.3533293691965,6.65964668342931,59.9085032102241));
#165001=CARTESIAN_POINT('Ctrl Pts',(66.3725199751832,6.67946812316823,59.9048047474849));
#165002=CARTESIAN_POINT('Ctrl Pts',(66.4081653352504,6.71596130276197,59.8979448358174));
#165003=CARTESIAN_POINT('Ctrl Pts',(66.4245957785227,6.73265679668973,59.894786645205));
#165004=CARTESIAN_POINT('Ctrl Pts',(66.4624375953624,6.77082165504112,59.8875214566757));
#165005=CARTESIAN_POINT('Ctrl Pts',(66.4838903579724,6.79224843342116,59.8834089948238));
#165006=CARTESIAN_POINT('Ctrl Pts',(66.5532233701834,6.86082823973365,59.8701367858147));
#165007=CARTESIAN_POINT('Ctrl Pts',(66.6015020342976,6.90756507122268,59.860923554787));
#165008=CARTESIAN_POINT('Ctrl Pts',(66.8922111241,7.18299217579198,59.8055936149524));
#165009=CARTESIAN_POINT('Ctrl Pts',(67.146045879201,7.3989718977528,59.7578766294237));
#165010=CARTESIAN_POINT('Ctrl Pts',(67.6347841056327,7.771770203166,59.6663354173845));
#165011=CARTESIAN_POINT('Ctrl Pts',(67.8664016884145,7.93239585626526,59.6230783364539));
#165012=CARTESIAN_POINT('Ctrl Pts',(68.2859011575263,8.19602138949855,59.544641764477));
#165013=CARTESIAN_POINT('Ctrl Pts',(68.4708131131366,8.30352124333549,59.5100398493929));
#165014=CARTESIAN_POINT('Ctrl Pts',(68.7861909734666,8.47259935880043,59.4508956317215));
#165015=CARTESIAN_POINT('Ctrl Pts',(68.9147412890686,8.53771126383773,59.4267541741647));
#165016=CARTESIAN_POINT('Ctrl Pts',(69.0974829948091,8.62498525819248,59.3923759285558));
#165017=CARTESIAN_POINT('Ctrl Pts',(69.1504870566599,8.64968583705695,59.3823976762416));
#165018=CARTESIAN_POINT('Ctrl Pts',(69.2421317857423,8.6913423680419,59.3651327296242));
#165019=CARTESIAN_POINT('Ctrl Pts',(69.2806647784383,8.70854058724726,59.3578697627547));
#165020=CARTESIAN_POINT('Ctrl Pts',(69.3594765051011,8.74307225362538,59.3430069905906));
#165021=CARTESIAN_POINT('Ctrl Pts',(69.3997632631269,8.7603839416773,59.3354053660714));
#165022=CARTESIAN_POINT('Ctrl Pts',(69.5017581447034,8.80335633743391,59.3161496575827));
#165023=CARTESIAN_POINT('Ctrl Pts',(69.5636185487956,8.82863364941053,59.3044613196241));
#165024=CARTESIAN_POINT('Ctrl Pts',(69.8016687807245,8.92290780269882,59.2594455518624));
#165025=CARTESIAN_POINT('Ctrl Pts',(69.9796211574574,8.98713361718635,59.2257163919939));
#165026=CARTESIAN_POINT('Ctrl Pts',(70.7411631041489,9.23581158035685,59.0810895768643));
#165027=CARTESIAN_POINT('Ctrl Pts',(71.3397562199109,9.36719190722697,58.9665975655292));
#165028=CARTESIAN_POINT('Ctrl Pts',(72.1991301160983,9.46755469557415,58.8030831991138));
#165029=CARTESIAN_POINT('Ctrl Pts',(72.4526317729423,9.48653004159974,58.7549709429072));
#165030=CARTESIAN_POINT('Ctrl Pts',(72.7667152643384,9.49694909165382,58.6957206744043));
#165031=CARTESIAN_POINT('Ctrl Pts',(72.8268225773865,9.49835171970258,58.6843981288054));
#165032=CARTESIAN_POINT('Ctrl Pts',(72.9148342969626,9.49954013994207,58.6678468103789));
#165033=CARTESIAN_POINT('Ctrl Pts',(72.9427284497063,9.4997895878609,58.6626051527566));
#165034=CARTESIAN_POINT('Ctrl Pts',(72.9920596382648,9.50000580113733,58.6533428463373));
#165035=CARTESIAN_POINT('Ctrl Pts',(73.0134958385132,9.5000246518641,58.6493206074091));
#165036=CARTESIAN_POINT('Ctrl Pts',(73.0601470328791,9.49990223896668,58.640572767602));
#165037=CARTESIAN_POINT('Ctrl Pts',(73.0853617591475,9.49973217395575,58.635848169112));
#165038=CARTESIAN_POINT('Ctrl Pts',(73.1559548792206,9.4989651516351,58.622630221057));
#165039=CARTESIAN_POINT('Ctrl Pts',(73.2013314827324,9.49813557559911,58.6141447288375));
#165040=CARTESIAN_POINT('Ctrl Pts',(73.4756717071102,9.49108498742324,58.5629014524727));
#165041=CARTESIAN_POINT('Ctrl Pts',(73.7043953227572,9.47663371187446,58.520424785588));
#165042=CARTESIAN_POINT('Ctrl Pts',(74.3917813650645,9.40732180445401,58.393091151301));
#165043=CARTESIAN_POINT('Ctrl Pts',(74.8472408255498,9.32642991849195,58.309125448333));
#165044=CARTESIAN_POINT('Ctrl Pts',(75.6180820042786,9.12874438023839,58.166267824476));
#165045=CARTESIAN_POINT('Ctrl Pts',(75.9366495404043,9.02832511309029,58.1070057134264));
#165046=CARTESIAN_POINT('Ctrl Pts',(76.3388574156216,8.87708762555163,58.0316901218072));
#165047=CARTESIAN_POINT('Ctrl Pts',(76.4280039083755,8.84197283064662,58.0149656603079));
#165048=CARTESIAN_POINT('Ctrl Pts',(76.5628067246537,8.78643424963575,57.9896255958651));
#165049=CARTESIAN_POINT('Ctrl Pts',(76.6088623295691,8.76702050247032,57.9809591105854));
#165050=CARTESIAN_POINT('Ctrl Pts',(76.6888663039483,8.73252899666594,57.9658884749638));
#165051=CARTESIAN_POINT('Ctrl Pts',(76.7228841115094,8.71761920191469,57.9594753548488));
#165052=CARTESIAN_POINT('Ctrl Pts',(76.7994668725098,8.68350139355711,57.9450262924261));
#165053=CARTESIAN_POINT('Ctrl Pts',(76.8419790785553,8.66417453909189,57.9369973369525));
#165054=CARTESIAN_POINT('Ctrl Pts',(76.9570610912391,8.61079983659528,57.9152407386684));
#165055=CARTESIAN_POINT('Ctrl Pts',(77.0293433770047,8.57612614010316,57.9015516568086));
#165056=CARTESIAN_POINT('Ctrl Pts',(77.4791503100287,8.35311436444787,57.8162181534779));
#165057=CARTESIAN_POINT('Ctrl Pts',(77.8441297628488,8.13994323877645,57.7462919457192));
#165058=CARTESIAN_POINT('Ctrl Pts',(78.4473444164101,7.73010710357301,57.6300039940216));
#165059=CARTESIAN_POINT('Ctrl Pts',(78.6925258560032,7.54519705412956,57.5825174256679));
#165060=CARTESIAN_POINT('Ctrl Pts',(79.0483369221912,7.24828745903619,57.5136000448928));
#165061=CARTESIAN_POINT('Ctrl Pts',(79.1658306746141,7.1451514156327,57.4908432673551));
#165062=CARTESIAN_POINT('Ctrl Pts',(79.3521655360193,6.97316513836637,57.4548150706156));
#165063=CARTESIAN_POINT('Ctrl Pts',(79.4225748466835,6.90612709784436,57.441216511164));
#165064=CARTESIAN_POINT('Ctrl Pts',(79.5172004461619,6.81319783560062,57.4229754134785));
#165065=CARTESIAN_POINT('Ctrl Pts',(79.5423080858706,6.78826108223574,57.4181387852745));
#165066=CARTESIAN_POINT('Ctrl Pts',(79.5842924771235,6.74609054399936,57.4100576752023));
#165067=CARTESIAN_POINT('Ctrl Pts',(79.6012430289379,6.72893380257166,57.4067968833195));
#165068=CARTESIAN_POINT('Ctrl Pts',(79.6337493060622,6.69577895143755,57.400547446014));
#165069=CARTESIAN_POINT('Ctrl Pts',(79.6493141742717,6.67979056201361,57.3975567301777));
#165070=CARTESIAN_POINT('Ctrl Pts',(79.6916039642043,6.63604086846163,57.3894351774488));
#165071=CARTESIAN_POINT('Ctrl Pts',(79.7182181437304,6.60816861267018,57.384328692972));
#165072=CARTESIAN_POINT('Ctrl Pts',(79.8217969324191,6.49835578827272,57.3644705497745));
#165073=CARTESIAN_POINT('Ctrl Pts',(79.8974917328053,6.41518117655755,57.3499923637494));
#165074=CARTESIAN_POINT('Ctrl Pts',(80.0629949456586,6.22667234011496,57.3183771873583));
#165075=CARTESIAN_POINT('Ctrl Pts',(80.1520256912976,6.12066379376989,57.3013982015584));
#165076=CARTESIAN_POINT('Ctrl Pts',(80.4886843335873,5.7014614296632,57.2371962021518));
#165077=CARTESIAN_POINT('Ctrl Pts',(80.7189754883046,5.37438790626149,57.193265298549));
#165078=CARTESIAN_POINT('Ctrl Pts',(81.0458748967027,4.84150598636741,57.1300555199009));
#165079=CARTESIAN_POINT('Ctrl Pts',(81.1568175176067,4.64534177307042,57.1084179589846));
#165080=CARTESIAN_POINT('Ctrl Pts',(81.3298969470347,4.31220727687835,57.074236822775));
#165081=CARTESIAN_POINT('Ctrl Pts',(81.395923056126,4.17742798080134,57.0610773912451));
#165082=CARTESIAN_POINT('Ctrl Pts',(81.4837841057505,3.98679968239584,57.043376120984));
#165083=CARTESIAN_POINT('Ctrl Pts',(81.5083049184154,3.93225307120993,57.0384133454154));
#165084=CARTESIAN_POINT('Ctrl Pts',(81.5494931035746,3.83827451042939,57.0300370307397));
#165085=CARTESIAN_POINT('Ctrl Pts',(81.5664100024378,3.79895744709865,57.0265844343452));
#165086=CARTESIAN_POINT('Ctrl Pts',(81.5982249145753,3.72362240157526,57.0200673153515));
#165087=CARTESIAN_POINT('Ctrl Pts',(81.6131677746623,3.68762492107599,57.0169957859893));
#165088=CARTESIAN_POINT('Ctrl Pts',(81.6514789843151,3.59371158363027,57.0090928535899));
#165089=CARTESIAN_POINT('Ctrl Pts',(81.6745016502744,3.53565223819036,57.0043156373833));
#165090=CARTESIAN_POINT('Ctrl Pts',(81.7527903732086,3.3324222750149,56.98797038004));
#165091=CARTESIAN_POINT('Ctrl Pts',(81.8050946220889,3.18610056891873,56.9768673450826));
#165092=CARTESIAN_POINT('Ctrl Pts',(82.0631810709142,2.40449066319536,56.9210693824057));
#165093=CARTESIAN_POINT('Ctrl Pts',(82.2057506654363,1.74961261556576,56.8862942838766));
#165094=CARTESIAN_POINT('Ctrl Pts',(82.3079845722295,0.827387173183443,
56.8556309596769));
#165095=CARTESIAN_POINT('Ctrl Pts',(82.3261564031287,0.568832582543673,
56.8490056737307));
#165096=CARTESIAN_POINT('Ctrl Pts',(82.3357834278011,0.248617195333988,
56.8434315861521));
#165097=CARTESIAN_POINT('Ctrl Pts',(82.337043428599,0.187394098147142,56.8424846281103));
#165098=CARTESIAN_POINT('Ctrl Pts',(82.3380389453491,0.0977708298033094,
56.841275725671));
#165099=CARTESIAN_POINT('Ctrl Pts',(82.3382296473736,0.069378543540619,
56.8409187928242));
#165100=CARTESIAN_POINT('Ctrl Pts',(82.3383275266771,0.0273237477979618,
56.8404290385353));
#165101=CARTESIAN_POINT('Ctrl Pts',(82.3383304712431,0.0136619004602319,
56.8402760238369));
#165102=CARTESIAN_POINT('Ctrl Pts',(82.3383045685277,6.65089060313308E-11,
56.8401291222381));
#165103=CARTESIAN_POINT('Origin',(73.0915550886457,-4.33680868994202E-16,
59.1075264962884));
#165104=CARTESIAN_POINT('',(82.2175389695453,-3.85097900598694E-11,56.1552333762936));
#165105=CARTESIAN_POINT('',(82.2254332530441,2.22253630170976E-12,56.2000040827795));
#165106=CARTESIAN_POINT('',(82.4472287422617,-1.59709532818419E-15,57.4578688084528));
#165107=CARTESIAN_POINT('Ctrl Pts',(82.2175389695453,-7.70179830244106E-11,
56.1552333762936));
#165108=CARTESIAN_POINT('Ctrl Pts',(82.2175620745244,0.0121862868716635,
56.1553644111411));
#165109=CARTESIAN_POINT('Ctrl Pts',(82.2175619477936,0.0243725649192966,
56.1554987250275));
#165110=CARTESIAN_POINT('Ctrl Pts',(82.2174857455006,0.0641335245306346,
56.155947728003));
#165111=CARTESIAN_POINT('Ctrl Pts',(82.2173139668202,0.0917076673255851,
56.1562760091775));
#165112=CARTESIAN_POINT('Ctrl Pts',(82.2165566947319,0.163543738420088,
56.1571759083335));
#165113=CARTESIAN_POINT('Ctrl Pts',(82.2157837221288,0.207802678087244,
56.1577745261521));
#165114=CARTESIAN_POINT('Ctrl Pts',(82.2061983382007,0.600873698792638,
56.1634922608861));
#165115=CARTESIAN_POINT('Ctrl Pts',(82.1786784220398,0.948923478496095,
56.1713709101551));
#165116=CARTESIAN_POINT('Ctrl Pts',(82.0538629847073,1.88018669068649,56.2012266847151));
#165117=CARTESIAN_POINT('Ctrl Pts',(81.9216856181147,2.45697178307319,56.229201204761));
#165118=CARTESIAN_POINT('Ctrl Pts',(81.6875862658055,3.17034383592015,56.2776770403699));
#165119=CARTESIAN_POINT('Ctrl Pts',(81.6336012798549,3.3219020002445,56.2888037339773));
#165120=CARTESIAN_POINT('Ctrl Pts',(81.5531229118076,3.53107093947884,56.3053371858243));
#165121=CARTESIAN_POINT('Ctrl Pts',(81.5298083402281,3.58992378570806,56.3101212559712));
#165122=CARTESIAN_POINT('Ctrl Pts',(81.491146103596,3.68476798626927,56.3180461257499));
#165123=CARTESIAN_POINT('Ctrl Pts',(81.4761553594863,3.72090851966491,56.3211169235837));
#165124=CARTESIAN_POINT('Ctrl Pts',(81.4443550207683,3.79626858230797,56.3276271313064));
#165125=CARTESIAN_POINT('Ctrl Pts',(81.4275041822755,3.83546905362349,56.3310746299236));
#165126=CARTESIAN_POINT('Ctrl Pts',(81.3867044148995,3.92866293587459,56.3394165991324));
#165127=CARTESIAN_POINT('Ctrl Pts',(81.3625185207907,3.98254646306949,56.3443575486508));
#165128=CARTESIAN_POINT('Ctrl Pts',(81.2771522854187,4.16812074730835,56.3617826966859));
#165129=CARTESIAN_POINT('Ctrl Pts',(81.2134940697439,4.29860307490458,56.3747524956992));
#165130=CARTESIAN_POINT('Ctrl Pts',(81.0482941283829,4.61852375479393,56.4083401359228));
#165131=CARTESIAN_POINT('Ctrl Pts',(80.9433123773971,4.806022412251,56.4296260573174));
#165132=CARTESIAN_POINT('Ctrl Pts',(80.6865899462031,5.23021834429121,56.4814658488889));
#165133=CARTESIAN_POINT('Ctrl Pts',(80.530558490987,5.46398204266914,56.5128259906746));
#165134=CARTESIAN_POINT('Ctrl Pts',(80.1648041338178,5.96244627766321,56.5857209756538));
#165135=CARTESIAN_POINT('Ctrl Pts',(79.9508678511729,6.22347209507369,56.6279797701092));
#165136=CARTESIAN_POINT('Ctrl Pts',(79.678105468441,6.521983184975,56.6810043200086));
#165137=CARTESIAN_POINT('Ctrl Pts',(79.6321377388087,6.57121556460514,56.6899132678471));
#165138=CARTESIAN_POINT('Ctrl Pts',(79.5646994463674,6.64190129658138,56.7029397132091));
#165139=CARTESIAN_POINT('Ctrl Pts',(79.5436435040226,6.66375768332045,56.7070008495884));
#165140=CARTESIAN_POINT('Ctrl Pts',(79.5061469828496,6.70230312436851,56.7142217205384));
#165141=CARTESIAN_POINT('Ctrl Pts',(79.4897488133509,6.71903399741452,56.7173758080022));
#165142=CARTESIAN_POINT('Ctrl Pts',(79.4539161931046,6.75532031285381,56.7242596750609));
#165143=CARTESIAN_POINT('Ctrl Pts',(79.434458260369,6.77485136752792,56.7279925614772));
#165144=CARTESIAN_POINT('Ctrl Pts',(79.3784249260081,6.83060084423773,56.7387280702822));
#165145=CARTESIAN_POINT('Ctrl Pts',(79.3416394927014,6.86660132105009,56.7457587203696));
#165146=CARTESIAN_POINT('Ctrl Pts',(79.0175287495276,7.1786073355827,56.8075703968907));
#165147=CARTESIAN_POINT('Ctrl Pts',(78.7133905672762,7.43609472433736,56.8646752078561));
#165148=CARTESIAN_POINT('Ctrl Pts',(77.9735201813484,7.98551216630177,57.0031456553133));
#165149=CARTESIAN_POINT('Ctrl Pts',(77.5279529581351,8.26149527837192,57.0862542394029));
#165150=CARTESIAN_POINT('Ctrl Pts',(76.983102419283,8.53846986069015,57.1885754105908));
#165151=CARTESIAN_POINT('Ctrl Pts',(76.9034471491996,8.57753525660988,57.203548851024));
#165152=CARTESIAN_POINT('Ctrl Pts',(76.7751386798869,8.6381939205145,57.2276938284204));
#165153=CARTESIAN_POINT('Ctrl Pts',(76.7268272047935,8.66052641760476,57.2367907960276));
#165154=CARTESIAN_POINT('Ctrl Pts',(76.6405008350899,8.69953263960527,57.2530565700462));
#165155=CARTESIAN_POINT('Ctrl Pts',(76.6025586872288,8.71637043882293,57.2602093307856));
#165156=CARTESIAN_POINT('Ctrl Pts',(76.5227956256994,8.75112733978341,57.2752538299828));
#165157=CARTESIAN_POINT('Ctrl Pts',(76.4809539725674,8.76899405052932,57.2831502259788));
#165158=CARTESIAN_POINT('Ctrl Pts',(76.3702229493109,8.81531470475086,57.3040593187258));
#165159=CARTESIAN_POINT('Ctrl Pts',(76.3011261214664,8.84324279410233,57.3171187399343));
#165160=CARTESIAN_POINT('Ctrl Pts',(75.9576090925401,8.97728014827677,57.3821030649231));
#165161=CARTESIAN_POINT('Ctrl Pts',(75.678739035092,9.07101369527477,57.4350499334955));
#165162=CARTESIAN_POINT('Ctrl Pts',(75.0612281700856,9.2461931608153,57.5525758406731));
#165163=CARTESIAN_POINT('Ctrl Pts',(74.721520829263,9.32205977431937,57.6174126566182));
#165164=CARTESIAN_POINT('Ctrl Pts',(73.9972657324468,9.44113101204135,57.7554901024172));
#165165=CARTESIAN_POINT('Ctrl Pts',(73.6126189152372,9.47965962981043,57.8287326794291));
#165166=CARTESIAN_POINT('Ctrl Pts',(73.1592396026607,9.496299819408,57.9143042024002));
#165167=CARTESIAN_POINT('Ctrl Pts',(73.0918262416238,9.49803008931145,57.9270078295874));
#165168=CARTESIAN_POINT('Ctrl Pts',(72.9980835743534,9.49940224097944,57.9446402841706));
#165169=CARTESIAN_POINT('Ctrl Pts',(72.9717688650273,9.49967420496134,57.9495863397234));
#165170=CARTESIAN_POINT('Ctrl Pts',(72.9237679607012,9.49996380483364,57.9586015502288));
#165171=CARTESIAN_POINT('Ctrl Pts',(72.9020823312584,9.50001777646759,57.9626718146363));
#165172=CARTESIAN_POINT('Ctrl Pts',(72.856938195237,9.49997012948229,57.971139498765));
#165173=CARTESIAN_POINT('Ctrl Pts',(72.8334798853964,9.49985543946105,57.9755364555061));
#165174=CARTESIAN_POINT('Ctrl Pts',(72.771431030582,9.49931420252947,57.9871588975185));
#165175=CARTESIAN_POINT('Ctrl Pts',(72.7328413227241,9.49873421311251,57.9943791863935));
#165176=CARTESIAN_POINT('Ctrl Pts',(72.5508299589987,9.49485057232465,58.0283999328086));
#165177=CARTESIAN_POINT('Ctrl Pts',(72.4074752508745,9.48842877138747,58.0550948567981));
#165178=CARTESIAN_POINT('Ctrl Pts',(71.9753540438651,9.45891434027047,58.1353667090422));
#165179=CARTESIAN_POINT('Ctrl Pts',(71.6874089123619,9.42552056815721,58.1885951733545));
#165180=CARTESIAN_POINT('Ctrl Pts',(70.8161170126059,9.28248609388585,58.3496263522637));
#165181=CARTESIAN_POINT('Ctrl Pts',(70.2411063311084,9.12994596080931,58.4559460771608));
#165182=CARTESIAN_POINT('Ctrl Pts',(69.5890838328112,8.88758409169151,58.5779859853179));
#165183=CARTESIAN_POINT('Ctrl Pts',(69.4943290835659,8.85056846763861,58.5957563229759));
#165184=CARTESIAN_POINT('Ctrl Pts',(69.3522345542083,8.79233419362202,58.6224607516421));
#165185=CARTESIAN_POINT('Ctrl Pts',(69.3044392768821,8.77227464282157,58.6314527881624));
#165186=CARTESIAN_POINT('Ctrl Pts',(69.2189114661975,8.73552884529499,58.647561331022));
#165187=CARTESIAN_POINT('Ctrl Pts',(69.1811182813761,8.71899074709797,58.6546856437987));
#165188=CARTESIAN_POINT('Ctrl Pts',(69.1007034504526,8.68315792932284,58.6698578751031));
#165189=CARTESIAN_POINT('Ctrl Pts',(69.0581143296217,8.66379122099352,58.6779014586559));
#165190=CARTESIAN_POINT('Ctrl Pts',(68.9425927259727,8.61019732111228,58.6997414808514));
#165191=CARTESIAN_POINT('Ctrl Pts',(68.8699516874946,8.57533592037105,58.7134988282191));
#165192=CARTESIAN_POINT('Ctrl Pts',(68.3808720939099,8.33270658786113,58.8062857783619));
#165193=CARTESIAN_POINT('Ctrl Pts',(67.9798541986424,8.09455740946324,58.8832076541506));
#165194=CARTESIAN_POINT('Ctrl Pts',(67.2147222754163,7.55860487548355,59.0308855936294));
#165195=CARTESIAN_POINT('Ctrl Pts',(66.8518098591758,7.26133843998112,59.101405090164));
#165196=CARTESIAN_POINT('Ctrl Pts',(66.4671849021322,6.89494858120251,59.1756746766675));
#165197=CARTESIAN_POINT('Ctrl Pts',(66.4226725371892,6.85169931982702,59.1842615147789));
#165198=CARTESIAN_POINT('Ctrl Pts',(66.3574947827016,6.78710758881896,59.1968186068262));
#165199=CARTESIAN_POINT('Ctrl Pts',(66.3365047582742,6.76610892278493,59.2008599820277));
#165200=CARTESIAN_POINT('Ctrl Pts',(66.2991860104668,6.72842073324678,59.2080401643776));
#165201=CARTESIAN_POINT('Ctrl Pts',(66.2828203404166,6.7117699534582,59.2111871401934));
#165202=CARTESIAN_POINT('Ctrl Pts',(66.2466333623729,6.67467835505118,59.2181415256148));
#165203=CARTESIAN_POINT('Ctrl Pts',(66.22684194196,6.65420778762587,59.2219423594693));
#165204=CARTESIAN_POINT('Ctrl Pts',(66.1684990950266,6.59331417175923,59.233139679782));
#165205=CARTESIAN_POINT('Ctrl Pts',(66.1302081089394,6.55263290968459,59.2404793232206));
#165206=CARTESIAN_POINT('Ctrl Pts',(66.0422595881523,6.45751774152815,59.2573204728252));
#165207=CARTESIAN_POINT('Ctrl Pts',(65.9928682087842,6.4028328036149,59.2667655933367));
#165208=CARTESIAN_POINT('Ctrl Pts',(65.8225424895113,6.20976098797361,59.2993078670539));
#165209=CARTESIAN_POINT('Ctrl Pts',(65.704949852707,6.06836792413911,59.3217230911174));
#165210=CARTESIAN_POINT('Ctrl Pts',(65.215870483904,5.44415901253735,59.4150013797009));
#165211=CARTESIAN_POINT('Ctrl Pts',(64.8867595558317,4.92884250935033,59.478011582582));
#165212=CARTESIAN_POINT('Ctrl Pts',(64.5493840775644,4.26797225134133,59.5448194755039));
#165213=CARTESIAN_POINT('Ctrl Pts',(64.4921291875201,4.14984913494886,59.5562517085704));
#165214=CARTESIAN_POINT('Ctrl Pts',(64.4154356828987,3.98291536388703,59.571712058257));
#165215=CARTESIAN_POINT('Ctrl Pts',(64.3939421956042,3.93509557823367,59.5760622783589));
#165216=CARTESIAN_POINT('Ctrl Pts',(64.3571627202203,3.85142731528745,59.5835377245434));
#165217=CARTESIAN_POINT('Ctrl Pts',(64.3417008356567,3.81566004262481,59.586690486836));
#165218=CARTESIAN_POINT('Ctrl Pts',(64.3097097940619,3.74039323108995,59.5932353433659));
#165219=CARTESIAN_POINT('Ctrl Pts',(64.2932262911236,3.70087462195001,59.5966202714521));
#165220=CARTESIAN_POINT('Ctrl Pts',(64.2543319561201,3.605830728441,59.6046383323961));
#165221=CARTESIAN_POINT('Ctrl Pts',(64.2321754608835,3.55020002443238,59.6092315914428));
#165222=CARTESIAN_POINT('Ctrl Pts',(64.1563921844887,3.35458757211139,59.6250345028206));
#165223=CARTESIAN_POINT('Ctrl Pts',(64.1055283720938,3.21352487109014,59.6358104759258));
#165224=CARTESIAN_POINT('Ctrl Pts',(63.988065760597,2.86205745497629,59.6611334279503));
#165225=CARTESIAN_POINT('Ctrl Pts',(63.9253765203239,2.65039565983729,59.6750591981307));
#165226=CARTESIAN_POINT('Ctrl Pts',(63.7884368219202,2.12161140682363,59.7065306162399));
#165227=CARTESIAN_POINT('Ctrl Pts',(63.7228996629691,1.80243963382905,59.722643823742));
#165228=CARTESIAN_POINT('Ctrl Pts',(63.6160865447336,1.10414900362851,59.7512898850749));
#165229=CARTESIAN_POINT('Ctrl Pts',(63.5808610013559,0.724622868931706,
59.7627366078957));
#165230=CARTESIAN_POINT('Ctrl Pts',(63.565811873296,0.276579473032023,59.7708582425205));
#165231=CARTESIAN_POINT('Ctrl Pts',(63.5642523957128,0.209213552212095,
59.771936077013));
#165232=CARTESIAN_POINT('Ctrl Pts',(63.5630465374347,0.114443810012844,
59.7732463666027));
#165233=CARTESIAN_POINT('Ctrl Pts',(63.5628140543119,0.0870511349330532,
59.7736008980186));
#165234=CARTESIAN_POINT('Ctrl Pts',(63.5626031218862,0.0374410612222554,
59.7741987545936));
#165235=CARTESIAN_POINT('Ctrl Pts',(63.5625849663477,0.0152240743026672,
59.7744504300767));
#165236=CARTESIAN_POINT('Ctrl Pts',(63.5627047979013,-0.0305737816256809,
59.7749358875716));
#165237=CARTESIAN_POINT('Ctrl Pts',(63.5628524406064,-0.0541544114140678,
59.7751676439857));
#165238=CARTESIAN_POINT('Ctrl Pts',(63.5634622090994,-0.115702896466913,
59.77572545554));
#165239=CARTESIAN_POINT('Ctrl Pts',(63.5640612526523,-0.153669231067783,
59.7760227548591));
#165240=CARTESIAN_POINT('Ctrl Pts',(63.5677400631327,-0.323564379696103,
59.777146552675));
#165241=CARTESIAN_POINT('Ctrl Pts',(63.5732895440022,-0.455428398293493,
59.7774613206361));
#165242=CARTESIAN_POINT('Ctrl Pts',(63.5971206372631,-0.836202868321354,
59.7768313736759));
#165243=CARTESIAN_POINT('Ctrl Pts',(63.6223320867661,-1.08456573484011,
59.7745165900299));
#165244=CARTESIAN_POINT('Ctrl Pts',(63.7443233637202,-1.95062406346372,
59.7602871509199));
#165245=CARTESIAN_POINT('Ctrl Pts',(63.8914315948919,-2.55945440010806,
59.7393107377751));
#165246=CARTESIAN_POINT('Ctrl Pts',(64.1385327652096,-3.26990492891155,
59.703122990503));
#165247=CARTESIAN_POINT('Ctrl Pts',(64.1828933734677,-3.38967454326454,
59.6965973917688));
#165248=CARTESIAN_POINT('Ctrl Pts',(64.2487108750063,-3.55701877615604,
59.6868826856176));
#165249=CARTESIAN_POINT('Ctrl Pts',(64.2681873933737,-3.60537513089997,
59.6840042273985));
#165250=CARTESIAN_POINT('Ctrl Pts',(64.3028981612861,-3.68956340370318,
59.6788681789778));
#165251=CARTESIAN_POINT('Ctrl Pts',(64.3179584121365,-3.72546734379838,
59.6766378467166));
#165252=CARTESIAN_POINT('Ctrl Pts',(64.3500969183202,-3.80079360850932,
59.6718744257086));
#165253=CARTESIAN_POINT('Ctrl Pts',(64.367222281152,-3.84019441151532,59.6693339571896));
#165254=CARTESIAN_POINT('Ctrl Pts',(64.4090693029255,-3.93472540099453,
59.663120875671));
#165255=CARTESIAN_POINT('Ctrl Pts',(64.4340481639736,-3.98973699671165,
59.6594079725064));
#165256=CARTESIAN_POINT('Ctrl Pts',(64.5244805229854,-4.18398537948775,
59.6459507146065));
#165257=CARTESIAN_POINT('Ctrl Pts',(64.5927608270677,-4.32184840076192,
59.6357630694951));
#165258=CARTESIAN_POINT('Ctrl Pts',(64.7729616938718,-4.6646132255352,59.6087960152249));
#165259=CARTESIAN_POINT('Ctrl Pts',(64.8891032179446,-4.86712635008318,
59.5913466483073));
#165260=CARTESIAN_POINT('Ctrl Pts',(65.2529335065035,-5.45082121639412,
59.5363472454328));
#165261=CARTESIAN_POINT('Ctrl Pts',(65.5204482048142,-5.81854141906376,
59.4955236191868));
#165262=CARTESIAN_POINT('Ctrl Pts',(65.9247370630333,-6.29813185639718,
59.4323873901518));
#165263=CARTESIAN_POINT('Ctrl Pts',(66.0401874079234,-6.4277107235389,59.4142141817589));
#165264=CARTESIAN_POINT('Ctrl Pts',(66.1897635683192,-6.58661150715075,
59.3904271706775));
#165265=CARTESIAN_POINT('Ctrl Pts',(66.2206889708783,-6.61900258610501,
59.3854966324181));
#165266=CARTESIAN_POINT('Ctrl Pts',(66.2700517067541,-6.66997796876365,
59.3776053745324));
#165267=CARTESIAN_POINT('Ctrl Pts',(66.2883413064505,-6.68870939939189,
59.3746770105363));
#165268=CARTESIAN_POINT('Ctrl Pts',(66.3234458981832,-6.72436576901142,
59.3690473612066));
#165269=CARTESIAN_POINT('Ctrl Pts',(66.3402478009024,-6.74130354862017,
59.3663489302962));
#165270=CARTESIAN_POINT('Ctrl Pts',(66.3809259913035,-6.7820025415984,59.3598067384754));
#165271=CARTESIAN_POINT('Ctrl Pts',(66.4048642247952,-6.80569921666708,
59.3559492727713));
#165272=CARTESIAN_POINT('Ctrl Pts',(66.4897143304273,-6.8888024955165,59.3422515156564));
#165273=CARTESIAN_POINT('Ctrl Pts',(66.5512873626772,-6.94750424524676,
59.3322668481808));
#165274=CARTESIAN_POINT('Ctrl Pts',(66.7084096821243,-7.0933063414243,59.3066948451297));
#165275=CARTESIAN_POINT('Ctrl Pts',(66.8049508350474,-7.17927490182089,
59.290898343425));
#165276=CARTESIAN_POINT('Ctrl Pts',(67.1613982950677,-7.48378914760924,
59.2323604180414));
#165277=CARTESIAN_POINT('Ctrl Pts',(67.4311086149228,-7.69007459519244,
59.1876745378135));
#165278=CARTESIAN_POINT('Ctrl Pts',(68.071693917673,-8.1270845017641,59.0814904797406));
#165279=CARTESIAN_POINT('Ctrl Pts',(68.4486107637276,-8.34730051285811,
59.0189927479848));
#165280=CARTESIAN_POINT('Ctrl Pts',(68.9115515542384,-8.57588875258249,
58.9427127267715));
#165281=CARTESIAN_POINT('Ctrl Pts',(68.9842489482258,-8.61061878555466,
58.9307464776536));
#165282=CARTESIAN_POINT('Ctrl Pts',(69.0999490490133,-8.66405919435124,
58.911722998239));
#165283=CARTESIAN_POINT('Ctrl Pts',(69.1426632811826,-8.68339801746371,
58.9047043961044));
#165284=CARTESIAN_POINT('Ctrl Pts',(69.2195870056219,-8.71752688826053,
58.8920729666375));
#165285=CARTESIAN_POINT('Ctrl Pts',(69.2537436153409,-8.73243619010334,
58.8864671222394));
#165286=CARTESIAN_POINT('Ctrl Pts',(69.3340446243686,-8.76691437695578,
58.8732949155118));
#165287=CARTESIAN_POINT('Ctrl Pts',(69.3802581938401,-8.78631576454893,
58.865719597622));
#165288=CARTESIAN_POINT('Ctrl Pts',(69.5154216480485,-8.84177899321317,
58.8435793224506));
#165289=CARTESIAN_POINT('Ctrl Pts',(69.604768676677,-8.87683519159539,58.8289636824492));
#165290=CARTESIAN_POINT('Ctrl Pts',(70.0072702993052,-9.02760911525914,
58.7632075382063));
#165291=CARTESIAN_POINT('Ctrl Pts',(70.3258850950275,-9.12774502686906,
58.7113985139972));
#165292=CARTESIAN_POINT('Ctrl Pts',(71.0969522993489,-9.32511883330916,
58.5863256146551));
#165293=CARTESIAN_POINT('Ctrl Pts',(71.5525869452587,-9.40608139030943,
58.5126788994558));
#165294=CARTESIAN_POINT('Ctrl Pts',(72.2438926967472,-9.47622088882419,
58.400244879462));
#165295=CARTESIAN_POINT('Ctrl Pts',(72.4763799309137,-9.49097891651943,
58.3623090960784));
#165296=CARTESIAN_POINT('Ctrl Pts',(72.7547908270631,-9.49812560070746,
58.3165745647492));
#165297=CARTESIAN_POINT('Ctrl Pts',(72.8004625647699,-9.49895958987249,
58.3090621959707));
#165298=CARTESIAN_POINT('Ctrl Pts',(72.8714751557372,-9.49973027764158,
58.2973645693163));
#165299=CARTESIAN_POINT('Ctrl Pts',(72.8968140488972,-9.49990115307864,
58.2931872194712));
#165300=CARTESIAN_POINT('Ctrl Pts',(72.9436688625342,-9.50002458677733,
58.2854561870684));
#165301=CARTESIAN_POINT('Ctrl Pts',(72.965184494514,-9.50000619109166,58.2819035101863));
#165302=CARTESIAN_POINT('Ctrl Pts',(73.0146645841112,-9.49979122393638,
58.2737274449891));
#165303=CARTESIAN_POINT('Ctrl Pts',(73.0426282400995,-9.49954289144836,
58.2691024635894));
#165304=CARTESIAN_POINT('Ctrl Pts',(73.1307367887179,-9.49836072409547,
58.2545173298241));
#165305=CARTESIAN_POINT('Ctrl Pts',(73.1908717925495,-9.49696688684111,
58.244544276516));
#165306=CARTESIAN_POINT('Ctrl Pts',(73.5041701253002,-9.48664528586601,
58.1925026773694));
#165307=CARTESIAN_POINT('Ctrl Pts',(73.7568704128003,-9.46790241810498,
58.150247235287));
#165308=CARTESIAN_POINT('Ctrl Pts',(74.6603698854748,-9.36341819237609,
57.9988155375674));
#165309=CARTESIAN_POINT('Ctrl Pts',(75.3025413293082,-9.21882108871517,
57.8906637770959));
#165310=CARTESIAN_POINT('Ctrl Pts',(76.0751313925175,-8.95629786087919,
57.7623404957863));
#165311=CARTESIAN_POINT('Ctrl Pts',(76.224168511168,-8.90135887875654,57.7376640911452));
#165312=CARTESIAN_POINT('Ctrl Pts',(76.4300017368328,-8.81944076371623,
57.7037070194924));
#165313=CARTESIAN_POINT('Ctrl Pts',(76.4880018947259,-8.79567680527895,
57.6941523172009));
#165314=CARTESIAN_POINT('Ctrl Pts',(76.5815080802493,-8.75625874296686,
57.6787713768637));
#165315=CARTESIAN_POINT('Ctrl Pts',(76.6171592983647,-8.74096698003743,
57.6729124962143));
#165316=CARTESIAN_POINT('Ctrl Pts',(76.6915260106254,-8.70851809124034,
57.6607026041018));
#165317=CARTESIAN_POINT('Ctrl Pts',(76.7302227439204,-8.69131863301243,
57.6543557230571));
#165318=CARTESIAN_POINT('Ctrl Pts',(76.8222676616797,-8.64965472452142,
57.6392745429163));
#165319=CARTESIAN_POINT('Ctrl Pts',(76.8755079820579,-8.62494783429335,
57.6305639782182));
#165320=CARTESIAN_POINT('Ctrl Pts',(77.0591192468841,-8.5376265410225,57.6005672169524));
#165321=CARTESIAN_POINT('Ctrl Pts',(77.1883002213919,-8.47247045301536,
57.5795398580098));
#165322=CARTESIAN_POINT('Ctrl Pts',(77.505290310716,-8.30324638365334,57.5281223737234));
#165323=CARTESIAN_POINT('Ctrl Pts',(77.6911784217267,-8.19563718395348,
57.4981331107367));
#165324=CARTESIAN_POINT('Ctrl Pts',(78.1125317238058,-7.93197826357809,
57.4304529739996));
#165325=CARTESIAN_POINT('Ctrl Pts',(78.3450435113787,-7.77145544903179,
57.3933335561804));
#165326=CARTESIAN_POINT('Ctrl Pts',(78.8358689351876,-7.39883103005937,
57.3151697379637));
#165327=CARTESIAN_POINT('Ctrl Pts',(79.0908960030443,-7.18291245339915,
57.2746861830794));
#165328=CARTESIAN_POINT('Ctrl Pts',(79.3830623834846,-6.90755410413531,
57.2280539009541));
#165329=CARTESIAN_POINT('Ctrl Pts',(79.4315945600879,-6.86082045483507,
57.2202984410942));
#165330=CARTESIAN_POINT('Ctrl Pts',(79.5012967023609,-6.79224424901472,
57.209141605724));
#165331=CARTESIAN_POINT('Ctrl Pts',(79.522864787333,-6.77081804980244,57.2056867114393));
#165332=CARTESIAN_POINT('Ctrl Pts',(79.5609114469926,-6.73265380055672,
57.1995869903538));
#165333=CARTESIAN_POINT('Ctrl Pts',(79.5774313805395,-6.71595835660609,
57.1969366955561));
#165334=CARTESIAN_POINT('Ctrl Pts',(79.6132720921959,-6.67946480850964,
57.1911827495876));
#165335=CARTESIAN_POINT('Ctrl Pts',(79.6325685684232,-6.65964293273335,
57.1880823450334));
#165336=CARTESIAN_POINT('Ctrl Pts',(79.6876784168167,-6.60253152853697,
57.1792212366246));
#165337=CARTESIAN_POINT('Ctrl Pts',(79.7232748410593,-6.56502954200024,
57.1734897490192));
#165338=CARTESIAN_POINT('Ctrl Pts',(79.8040039113589,-6.47856586838472,
57.1604767127394));
#165339=CARTESIAN_POINT('Ctrl Pts',(79.8489323281395,-6.42941297542616,
57.1532238516866));
#165340=CARTESIAN_POINT('Ctrl Pts',(79.9980546995396,-6.26276313442566,
57.1291258705521));
#165341=CARTESIAN_POINT('Ctrl Pts',(80.0998629457856,-6.14311628286953,
57.1126323285365));
#165342=CARTESIAN_POINT('Ctrl Pts',(80.3929830460275,-5.78074458578222,
57.0651409734119));
#165343=CARTESIAN_POINT('Ctrl Pts',(80.5755427005811,-5.53102836071804,
57.0355623913189));
#165344=CARTESIAN_POINT('Ctrl Pts',(80.9802669564043,-4.91675757855925,
56.9705976841673));
#165345=CARTESIAN_POINT('Ctrl Pts',(81.1908643999103,-4.54517358206381,
56.9373313267025));
#165346=CARTESIAN_POINT('Ctrl Pts',(81.4113813377762,-4.08738135032824,
56.903668062532));
#165347=CARTESIAN_POINT('Ctrl Pts',(81.4456740060786,-4.01381968472663,
56.8984723920213));
#165348=CARTESIAN_POINT('Ctrl Pts',(81.4984732922601,-3.89670774432487,
56.8905385038862));
#165349=CARTESIAN_POINT('Ctrl Pts',(81.517594267403,-3.85344708955096,56.887679769165));
#165350=CARTESIAN_POINT('Ctrl Pts',(81.5513531681741,-3.77551870635186,
56.8826592486652));
#165351=CARTESIAN_POINT('Ctrl Pts',(81.5661077480066,-3.74090409221866,
56.8804745596192));
#165352=CARTESIAN_POINT('Ctrl Pts',(81.6002440999726,-3.65949864885815,
56.8754429062316));
#165353=CARTESIAN_POINT('Ctrl Pts',(81.6194609877526,-3.61263794251452,
56.8726282660487));
#165354=CARTESIAN_POINT('Ctrl Pts',(81.6744455782646,-3.47548322584599,
56.864628232049));
#165355=CARTESIAN_POINT('Ctrl Pts',(81.7092217585729,-3.38478754154093,
56.8596371019274));
#165356=CARTESIAN_POINT('Ctrl Pts',(81.8590565514482,-2.97561238638222,
56.8384509770979));
#165357=CARTESIAN_POINT('Ctrl Pts',(81.958699239592,-2.6515985568033,56.8252708302773));
#165358=CARTESIAN_POINT('Ctrl Pts',(82.1552523845467,-1.86766016950789,
56.8015427679651));
#165359=CARTESIAN_POINT('Ctrl Pts',(82.2360663723526,-1.40452785883608,
56.7940116455042));
#165360=CARTESIAN_POINT('Ctrl Pts',(82.3059376725285,-0.705470276392925,
56.7911260463762));
#165361=CARTESIAN_POINT('Ctrl Pts',(82.3206849691564,-0.472851123781757,
56.7915423018543));
#165362=CARTESIAN_POINT('Ctrl Pts',(82.3281960917859,-0.193782709245965,
56.7935378153007));
#165363=CARTESIAN_POINT('Ctrl Pts',(82.3291052846221,-0.147622223252684,
56.7939167965575));
#165364=CARTESIAN_POINT('Ctrl Pts',(82.3300012247138,-0.0758064396675572,
56.7945808515836));
#165365=CARTESIAN_POINT('Ctrl Pts',(82.3302183408803,-0.050154416533749,
56.7948328187476));
#165366=CARTESIAN_POINT('Ctrl Pts',(82.3303688796997,-0.0163346475376253,
56.7951842479547));
#165367=CARTESIAN_POINT('Ctrl Pts',(82.3303947999415,-0.00816731830620228,
56.7952705954578));
#165368=CARTESIAN_POINT('Ctrl Pts',(82.3304102850288,-6.66914478404779E-11,
56.7953584157516));
#165369=CARTESIAN_POINT('Ctrl Pts',(82.3383045685277,6.65089060313308E-11,
56.8401291222381));
#165370=CARTESIAN_POINT('Ctrl Pts',(82.3382891198383,-0.00814812083209077,
56.8400415083665));
#165371=CARTESIAN_POINT('Ctrl Pts',(82.3382634099389,-0.0162962606031404,
56.8399560689772));
#165372=CARTESIAN_POINT('Ctrl Pts',(82.3381142235792,-0.0500886157455977,
56.8396107235002));
#165373=CARTESIAN_POINT('Ctrl Pts',(82.3378993598792,-0.0757324820082624,
56.8393701306411));
#165374=CARTESIAN_POINT('Ctrl Pts',(82.3370133961438,-0.147503556506034,
56.8387563346514));
#165375=CARTESIAN_POINT('Ctrl Pts',(82.3361149589866,-0.193627645666198,
56.8384307441625));
#165376=CARTESIAN_POINT('Ctrl Pts',(82.3287105975161,-0.471784942100996,
56.8368758697467));
#165377=CARTESIAN_POINT('Ctrl Pts',(82.3142028398022,-0.703535625737106,
56.8372945169323));
#165378=CARTESIAN_POINT('Ctrl Pts',(82.2451559517499,-1.40204384123383,
56.8433425556184));
#165379=CARTESIAN_POINT('Ctrl Pts',(82.1649285806936,-1.86548886623128,
56.8538309024253));
#165380=CARTESIAN_POINT('Ctrl Pts',(81.9690154662661,-2.65026386832995,
56.8814326097488));
#165381=CARTESIAN_POINT('Ctrl Pts',(81.8694801133853,-2.97478760329092,
56.8958893521575));
#165382=CARTESIAN_POINT('Ctrl Pts',(81.7196022110395,-3.38452010758047,
56.917915740973));
#165383=CARTESIAN_POINT('Ctrl Pts',(81.6848255031272,-3.47528461757496,
56.9230415830219));
#165384=CARTESIAN_POINT('Ctrl Pts',(81.6298318777468,-3.61252089360705,
56.9311668709349));
#165385=CARTESIAN_POINT('Ctrl Pts',(81.6106148190805,-3.6593954274055,56.9340095719962));
#165386=CARTESIAN_POINT('Ctrl Pts',(81.5764771614856,-3.74081598299976,
56.9390650279483));
#165387=CARTESIAN_POINT('Ctrl Pts',(81.5617227328761,-3.77543202779978,
56.9412517604641));
#165388=CARTESIAN_POINT('Ctrl Pts',(81.5279659739346,-3.85335226620104,
56.9462586496192));
#165389=CARTESIAN_POINT('Ctrl Pts',(81.5088463702305,-3.89660337226774,
56.9490971738732));
#165390=CARTESIAN_POINT('Ctrl Pts',(81.4560582893587,-4.01366099589013,
56.9569413162896));
#165391=CARTESIAN_POINT('Ctrl Pts',(81.4217723907162,-4.08717814071998,
56.9620436852196));
#165392=CARTESIAN_POINT('Ctrl Pts',(81.2022765377962,-4.54260135140602,
56.9947577934366));
#165393=CARTESIAN_POINT('Ctrl Pts',(80.9928312549118,-4.9120155174059,57.0261554780359));
#165394=CARTESIAN_POINT('Ctrl Pts',(80.4917720065388,-5.6727623075419,57.1022244479419));
#165395=CARTESIAN_POINT('Ctrl Pts',(80.1933065189435,-6.05801669622355,
57.148060138746));
#165396=CARTESIAN_POINT('Ctrl Pts',(79.8102897917012,-6.48109335088491,
57.2085567934619));
#165397=CARTESIAN_POINT('Ctrl Pts',(79.7526440586559,-6.54308221655692,
57.2177026258355));
#165398=CARTESIAN_POINT('Ctrl Pts',(79.6709682595171,-6.62859098653333,
57.2307261813518));
#165399=CARTESIAN_POINT('Ctrl Pts',(79.6476187347245,-6.65277776772802,
57.2344566311803));
#165400=CARTESIAN_POINT('Ctrl Pts',(79.6074889607966,-6.69390710144073,
57.2408810574269));
#165401=CARTESIAN_POINT('Ctrl Pts',(79.5907713126838,-6.71091248007769,
57.2435612451249));
#165402=CARTESIAN_POINT('Ctrl Pts',(79.5555464442626,-6.74647455622879,
57.2492167994907));
#165403=CARTESIAN_POINT('Ctrl Pts',(79.5370264080459,-6.76501760683904,
57.2521949918781));
#165404=CARTESIAN_POINT('Ctrl Pts',(79.486560666629,-6.8151289741064,57.260322450614));
#165405=CARTESIAN_POINT('Ctrl Pts',(79.4544697775737,-6.84654490320242,
57.265503702611));
#165406=CARTESIAN_POINT('Ctrl Pts',(79.2959633071769,-6.99952600169218,
57.2911537617373));
#165407=CARTESIAN_POINT('Ctrl Pts',(79.1664680583497,-7.11773790032335,
57.312288758826));
#165408=CARTESIAN_POINT('Ctrl Pts',(78.6947239030557,-7.52488294235893,
57.389690861074));
#165409=CARTESIAN_POINT('Ctrl Pts',(78.33560004559,-7.79268367816114,57.4493206218922));
#165410=CARTESIAN_POINT('Ctrl Pts',(77.7626713821278,-8.15921882331197,
57.5442831301041));
#165411=CARTESIAN_POINT('Ctrl Pts',(77.561765893465,-8.27740376737075,57.5775603803411));
#165412=CARTESIAN_POINT('Ctrl Pts',(77.2218963972632,-8.46056403265779,
57.6337081930567));
#165413=CARTESIAN_POINT('Ctrl Pts',(77.0853321787573,-8.52987368028322,
57.6562322506337));
#165414=CARTESIAN_POINT('Ctrl Pts',(76.8930291014963,-8.62158123135433,
57.6878834588329));
#165415=CARTESIAN_POINT('Ctrl Pts',(76.8386639716943,-8.64686570101434,
57.6968242991517));
#165416=CARTESIAN_POINT('Ctrl Pts',(76.7452835752686,-8.6892029638159,57.7121687408336));
#165417=CARTESIAN_POINT('Ctrl Pts',(76.7063864910668,-8.70651743802117,
57.7185566226445));
#165418=CARTESIAN_POINT('Ctrl Pts',(76.632050345331,-8.73899753144086,57.7307571678895));
#165419=CARTESIAN_POINT('Ctrl Pts',(76.5966327910462,-8.75421122066174,
57.7365669923477));
#165420=CARTESIAN_POINT('Ctrl Pts',(76.5136263863602,-8.78925715945195,
57.7501757716148));
#165421=CARTESIAN_POINT('Ctrl Pts',(76.4659664357693,-8.80891415244796,
57.757983880163));
#165422=CARTESIAN_POINT('Ctrl Pts',(76.3012481704526,-8.87525330624797,
57.7849500283185));
#165423=CARTESIAN_POINT('Ctrl Pts',(76.1834195122918,-8.91994521349711,
57.8042057926309));
#165424=CARTESIAN_POINT('Ctrl Pts',(75.4821847703952,-9.16972679342884,
57.9186130025399));
#165425=CARTESIAN_POINT('Ctrl Pts',(74.8806828286827,-9.31841977507539,
58.0158504841562));
#165426=CARTESIAN_POINT('Ctrl Pts',(74.0251887455363,-9.44114770390028,
58.154604647467));
#165427=CARTESIAN_POINT('Ctrl Pts',(73.7799090336407,-9.46639748679715,
58.194456443081));
#165428=CARTESIAN_POINT('Ctrl Pts',(73.4039365392849,-9.48999050918296,
58.2558643071637));
#165429=CARTESIAN_POINT('Ctrl Pts',(73.2737602961642,-9.49540366951665,
58.2771853229029));
#165430=CARTESIAN_POINT('Ctrl Pts',(73.1060636457311,-9.49883267548552,
58.3047588904063));
#165431=CARTESIAN_POINT('Ctrl Pts',(73.0685954717932,-9.49937111005168,
58.3109265067517));
#165432=CARTESIAN_POINT('Ctrl Pts',(73.0078579930843,-9.49987485773845,
58.3209366329845));
#165433=CARTESIAN_POINT('Ctrl Pts',(72.9845894887032,-9.4999800408816,58.3247744019422));
#165434=CARTESIAN_POINT('Ctrl Pts',(72.9394000510039,-9.5000137932809,58.3322335828487));
#165435=CARTESIAN_POINT('Ctrl Pts',(72.9174793054033,-9.4999522333362,58.3358546435921));
#165436=CARTESIAN_POINT('Ctrl Pts',(72.8685329971397,-9.49964075421995,
58.34394581901));
#165437=CARTESIAN_POINT('Ctrl Pts',(72.8415080465706,-9.49935029565232,
58.3484171788094));
#165438=CARTESIAN_POINT('Ctrl Pts',(72.7480191127264,-9.49793557256114,
58.3638979962211));
#165439=CARTESIAN_POINT('Ctrl Pts',(72.681568961811,-9.49621312767748,58.3749238270209));
#165440=CARTESIAN_POINT('Ctrl Pts',(72.2401001081261,-9.48000410984894,
58.4483000399238));
#165441=CARTESIAN_POINT('Ctrl Pts',(71.8663044416641,-9.44341045802422,
58.5110154141277));
#165442=CARTESIAN_POINT('Ctrl Pts',(71.1799472255596,-9.33373857175741,
58.626223208806));
#165443=CARTESIAN_POINT('Ctrl Pts',(70.8669668489122,-9.26693797821629,
58.6787791897272));
#165444=CARTESIAN_POINT('Ctrl Pts',(70.345705704735,-9.12712855994394,58.7659368782599));
#165445=CARTESIAN_POINT('Ctrl Pts',(70.1355039027462,-9.06266400849372,
58.800980257732));
#165446=CARTESIAN_POINT('Ctrl Pts',(69.7867036701401,-8.94199618926502,
58.858875235428));
#165447=CARTESIAN_POINT('Ctrl Pts',(69.6468593818436,-8.8898161252199,58.8820169457841));
#165448=CARTESIAN_POINT('Ctrl Pts',(69.4530881736079,-8.81215633149435,
58.9139731088817));
#165449=CARTESIAN_POINT('Ctrl Pts',(69.3980940694496,-8.7895021137613,58.923030097148));
#165450=CARTESIAN_POINT('Ctrl Pts',(69.304186625981,-8.74976213341657,58.938473884576));
#165451=CARTESIAN_POINT('Ctrl Pts',(69.2651695850224,-8.73293535947142,
58.9448840077675));
#165452=CARTESIAN_POINT('Ctrl Pts',(69.1861929198891,-8.69823313779756,
58.9578457601869));
#165453=CARTESIAN_POINT('Ctrl Pts',(69.1462411574451,-8.68034180201397,
58.9643956967812));
#165454=CARTESIAN_POINT('Ctrl Pts',(69.0463833524403,-8.63477667329076,
58.9807494089848));
#165455=CARTESIAN_POINT('Ctrl Pts',(68.9866374197206,-8.60674526147473,
58.9905180043304));
#165456=CARTESIAN_POINT('Ctrl Pts',(68.7623644378776,-8.49860556379902,
59.0271272788361));
#165457=CARTESIAN_POINT('Ctrl Pts',(68.5998493962872,-8.41427389444658,
59.0535319548189));
#165458=CARTESIAN_POINT('Ctrl Pts',(68.0050549825197,-8.08311244600899,
59.1497548166022));
#165459=CARTESIAN_POINT('Ctrl Pts',(67.589761679224,-7.80647073900792,59.2160517040286));
#165460=CARTESIAN_POINT('Ctrl Pts',(66.9770061171303,-7.32378912219253,
59.3135578327648));
#165461=CARTESIAN_POINT('Ctrl Pts',(66.763799892022,-7.13977014183352,59.3474297706064));
#165462=CARTESIAN_POINT('Ctrl Pts',(66.5118336070239,-6.90175497267654,
59.3876509196392));
#165463=CARTESIAN_POINT('Ctrl Pts',(66.4650570060535,-6.8566430830874,59.3951266518842));
#165464=CARTESIAN_POINT('Ctrl Pts',(66.3971643764735,-6.78979618803113,
59.40599449451));
#165465=CARTESIAN_POINT('Ctrl Pts',(66.3756841422253,-6.76844174794148,
59.4094355249902));
#165466=CARTESIAN_POINT('Ctrl Pts',(66.3393414064274,-6.73196149866272,
59.4152624260524));
#165467=CARTESIAN_POINT('Ctrl Pts',(66.3244268651676,-6.71688905260032,
59.4176551600178));
#165468=CARTESIAN_POINT('Ctrl Pts',(66.2905247219258,-6.68239573820875,
59.423097503339));
#165469=CARTESIAN_POINT('Ctrl Pts',(66.2715697401444,-6.66294263334712,
59.4261427903341));
#165470=CARTESIAN_POINT('Ctrl Pts',(66.2193479518454,-6.60888280405673,
59.4345387651169));
#165471=CARTESIAN_POINT('Ctrl Pts',(66.1862591988292,-6.57410152573327,
59.4398655088593));
#165472=CARTESIAN_POINT('Ctrl Pts',(65.9895407200568,-6.36413328023457,
59.4715677476172));
#165473=CARTESIAN_POINT('Ctrl Pts',(65.8323053909597,-6.18294182417754,
59.4970470434239));
#165474=CARTESIAN_POINT('Ctrl Pts',(65.4139768909903,-5.66217158899336,
59.564824962373));
#165475=CARTESIAN_POINT('Ctrl Pts',(65.1685917171156,-5.31039660839245,
59.6045502507485));
#165476=CARTESIAN_POINT('Ctrl Pts',(64.8421678676457,-4.76800559669767,
59.6564144319839));
#165477=CARTESIAN_POINT('Ctrl Pts',(64.7424525298315,-4.58962278672968,
59.6720952268352));
#165478=CARTESIAN_POINT('Ctrl Pts',(64.5840594199962,-4.28369563725791,
59.6966455880169));
#165479=CARTESIAN_POINT('Ctrl Pts',(64.5223581216261,-4.15784495367329,
59.706103591619));
#165480=CARTESIAN_POINT('Ctrl Pts',(64.4388942640089,-3.97773640434789,
59.7187304472165));
#165481=CARTESIAN_POINT('Ctrl Pts',(64.4148501530161,-3.92458792715902,
59.7223466376905));
#165482=CARTESIAN_POINT('Ctrl Pts',(64.3740895103105,-3.83225968033606,
59.728438731005));
#165483=CARTESIAN_POINT('Ctrl Pts',(64.3571478838635,-3.79318411912509,
59.7309588142063));
#165484=CARTESIAN_POINT('Ctrl Pts',(64.3229580128775,-3.71286833168708,
59.7360194070704));
#165485=CARTESIAN_POINT('Ctrl Pts',(64.3057364256814,-3.671617581086,59.7385547068335));
#165486=CARTESIAN_POINT('Ctrl Pts',(64.2626582208189,-3.56637601683405,
59.7448608344492));
#165487=CARTESIAN_POINT('Ctrl Pts',(64.2371996887342,-3.5022204508791,59.7485536388536));
#165488=CARTESIAN_POINT('Ctrl Pts',(64.1396494799542,-3.24846897680569,
59.7625658668281));
#165489=CARTESIAN_POINT('Ctrl Pts',(64.0728462955235,-3.05684167186129,
59.7718500956756));
#165490=CARTESIAN_POINT('Ctrl Pts',(63.8302999026047,-2.28335826072466,
59.8042539588884));
#165491=CARTESIAN_POINT('Ctrl Pts',(63.7035572942958,-1.6872577654847,59.8178608246046));
#165492=CARTESIAN_POINT('Ctrl Pts',(63.6042199759272,-0.826161271478044,
59.8235794039326));
#165493=CARTESIAN_POINT('Ctrl Pts',(63.584941015755,-0.568092738134471,
59.8235648025054));
#165494=CARTESIAN_POINT('Ctrl Pts',(63.5740151111343,-0.24842110306705,
59.8216215683852));
#165495=CARTESIAN_POINT('Ctrl Pts',(63.5725096607896,-0.187253550499851,
59.8211629249535));
#165496=CARTESIAN_POINT('Ctrl Pts',(63.5711624976983,-0.0976961981605212,
59.8203678857497));
#165497=CARTESIAN_POINT('Ctrl Pts',(63.5708615335676,-0.0693142617862874,
59.8200977716372));
#165498=CARTESIAN_POINT('Ctrl Pts',(63.5705521286986,-0.0191226706383749,
59.8195884233807));
#165499=CARTESIAN_POINT('Ctrl Pts',(63.5704920855359,0.00268643736458375,
59.8193565502891));
#165500=CARTESIAN_POINT('Ctrl Pts',(63.5705233418788,0.0501471080253307,
59.8188290714159));
#165501=CARTESIAN_POINT('Ctrl Pts',(63.5706431601227,0.0757982329107289,
59.8185293918815));
#165502=CARTESIAN_POINT('Ctrl Pts',(63.571266653737,0.147608961795316,59.8176490302096));
#165503=CARTESIAN_POINT('Ctrl Pts',(63.5720006498833,0.193765439259529,
59.8170352762708));
#165504=CARTESIAN_POINT('Ctrl Pts',(63.5784502802361,0.472730219005996,
59.8130294096185));
#165505=CARTESIAN_POINT('Ctrl Pts',(63.5923046411714,0.705253654915414,
59.8084408079444));
#165506=CARTESIAN_POINT('Ctrl Pts',(63.6594860003008,1.40425150710594,59.7904661814547));
#165507=CARTESIAN_POINT('Ctrl Pts',(63.7385182906675,1.86741632043335,59.7728744661237));
#165508=CARTESIAN_POINT('Ctrl Pts',(63.9320210802418,2.65145158777694,59.73181650814));
#165509=CARTESIAN_POINT('Ctrl Pts',(64.0303980899176,2.97552323593261,59.7113795106899));
#165510=CARTESIAN_POINT('Ctrl Pts',(64.1786056606585,3.384757610258,59.6808504330921));
#165511=CARTESIAN_POINT('Ctrl Pts',(64.2130174665081,3.4754611109181,59.6737771000189));
#165512=CARTESIAN_POINT('Ctrl Pts',(64.2674468321649,3.61262476229139,59.6626089507711));
#165513=CARTESIAN_POINT('Ctrl Pts',(64.2864728454777,3.65948703939793,59.6587084964783));
#165514=CARTESIAN_POINT('Ctrl Pts',(64.3202760882699,3.74089414323485,59.6517842797708));
#165515=CARTESIAN_POINT('Ctrl Pts',(64.334888444784,3.77550891937578,59.6487928633556));
#165516=CARTESIAN_POINT('Ctrl Pts',(64.3683257847376,3.85343641493831,59.6419515151001));
#165517=CARTESIAN_POINT('Ctrl Pts',(64.3872673913714,3.8966959826217,59.638078705817));
#165518=CARTESIAN_POINT('Ctrl Pts',(64.4395780297585,4.01380194499636,59.6273904696222));
#165519=CARTESIAN_POINT('Ctrl Pts',(64.4735612223689,4.08735854101666,59.620454614892));
#165520=CARTESIAN_POINT('Ctrl Pts',(64.6920282388881,4.5448871158386,59.5759160712281));
#165521=CARTESIAN_POINT('Ctrl Pts',(64.9008496716447,4.91622406437002,59.5335288811215));
#165522=CARTESIAN_POINT('Ctrl Pts',(65.3021916909747,5.52972072239749,59.4528495573519));
#165523=CARTESIAN_POINT('Ctrl Pts',(65.4831327492413,5.77893126066466,59.4166994414878));
#165524=CARTESIAN_POINT('Ctrl Pts',(65.7743387200406,6.14135779497294,59.3591727318873));
#165525=CARTESIAN_POINT('Ctrl Pts',(65.8759260072531,6.26150186322094,59.3392122245946));
#165526=CARTESIAN_POINT('Ctrl Pts',(66.0247073585395,6.42876363235173,59.3101816008895));
#165527=CARTESIAN_POINT('Ctrl Pts',(66.0694945033245,6.47804861258835,59.3014675179556));
#165528=CARTESIAN_POINT('Ctrl Pts',(66.1499567393336,6.56472028971193,59.2858615364453));
#165529=CARTESIAN_POINT('Ctrl Pts',(66.1854260945617,6.60229945594327,59.2789986377992));
#165530=CARTESIAN_POINT('Ctrl Pts',(66.2403193947665,6.65950313591282,59.2684049029855));
#165531=CARTESIAN_POINT('Ctrl Pts',(66.2595251783984,6.67934105018914,59.2647034915859));
#165532=CARTESIAN_POINT('Ctrl Pts',(66.2951834870417,6.71584869304943,59.2578410516431));
#165533=CARTESIAN_POINT('Ctrl Pts',(66.3116115446323,6.73254233068394,59.2546833021266));
#165534=CARTESIAN_POINT('Ctrl Pts',(66.3494284177101,6.77068336620272,59.2474228628374));
#165535=CARTESIAN_POINT('Ctrl Pts',(66.3708584232646,6.79208837954643,59.2433147354011));
#165536=CARTESIAN_POINT('Ctrl Pts',(66.4400423635843,6.86052450730752,59.2300709566091));
#165537=CARTESIAN_POINT('Ctrl Pts',(66.4881923278073,6.90714194437685,59.2208821445063));
#165538=CARTESIAN_POINT('Ctrl Pts',(66.7752858461878,7.17918920175889,59.1662392248061));
#165539=CARTESIAN_POINT('Ctrl Pts',(67.0253014182388,7.39228551958493,59.1192318487562));
#165540=CARTESIAN_POINT('Ctrl Pts',(67.5034472448691,7.75822600399336,59.0296645377486));
#165541=CARTESIAN_POINT('Ctrl Pts',(67.7281875487765,7.91504007874153,58.9876878795011));
#165542=CARTESIAN_POINT('Ctrl Pts',(68.146618551493,8.18041205986879,58.9094577242688));
#165543=CARTESIAN_POINT('Ctrl Pts',(68.3379754705029,8.29239626911787,58.8736555114032));
#165544=CARTESIAN_POINT('Ctrl Pts',(68.663183631851,8.46742300652365,58.812673695601));
#165545=CARTESIAN_POINT('Ctrl Pts',(68.7949331382456,8.53432572416359,58.7879333130593));
#165546=CARTESIAN_POINT('Ctrl Pts',(68.9814384712572,8.62349745290284,58.7528481575374));
#165547=CARTESIAN_POINT('Ctrl Pts',(69.0349368293633,8.64845105545213,58.7427771152779));
#165548=CARTESIAN_POINT('Ctrl Pts',(69.1271664341179,8.69040220825668,58.7254023231396));
#165549=CARTESIAN_POINT('Ctrl Pts',(69.1657862312919,8.70765039960893,58.7181231292446));
#165550=CARTESIAN_POINT('Ctrl Pts',(69.2398247200556,8.74011063280711,58.7041607633761));
#165551=CARTESIAN_POINT('Ctrl Pts',(69.2752236142209,8.75536749592927,58.6974819722294));
#165552=CARTESIAN_POINT('Ctrl Pts',(69.3676642982094,8.79452643052515,58.6800326065029));
#165553=CARTESIAN_POINT('Ctrl Pts',(69.4248471276524,8.81807638992534,58.6692303525148));
#165554=CARTESIAN_POINT('Ctrl Pts',(69.6255041614652,8.89837022196516,58.6312958932814));
#165555=CARTESIAN_POINT('Ctrl Pts',(69.7701161991164,8.95207794735394,58.6039050835263));
#165556=CARTESIAN_POINT('Ctrl Pts',(70.6011859479906,9.23725048906812,58.4462252347092));
#165557=CARTESIAN_POINT('Ctrl Pts',(71.3106780489233,9.3905309173788,58.3103429840408));
#165558=CARTESIAN_POINT('Ctrl Pts',(72.2449468095197,9.47926456171249,58.1328559682745));
#165559=CARTESIAN_POINT('Ctrl Pts',(72.4599516368399,9.49206922263139,58.0921278131034));
#165560=CARTESIAN_POINT('Ctrl Pts',(72.7186518143162,9.49835056324411,58.0433913083779));
#165561=CARTESIAN_POINT('Ctrl Pts',(72.7620738516078,9.49909645472195,58.0352201700255));
#165562=CARTESIAN_POINT('Ctrl Pts',(72.8300183963571,9.49978114026535,58.0224501711866));
#165563=CARTESIAN_POINT('Ctrl Pts',(72.8545369998379,9.49992994799619,58.0178451772617));
#165564=CARTESIAN_POINT('Ctrl Pts',(72.9006137882423,9.50002493860347,58.0091975680271));
#165565=CARTESIAN_POINT('Ctrl Pts',(72.9221714581237,9.49999342872577,58.00515431673));
#165566=CARTESIAN_POINT('Ctrl Pts',(72.972237131677,9.49974386434254,57.9957702280188));
#165567=CARTESIAN_POINT('Ctrl Pts',(73.0007449635042,9.4994689461167,57.9904313259286));
#165568=CARTESIAN_POINT('Ctrl Pts',(73.0944403425512,9.49812885153303,57.9728979660669));
#165569=CARTESIAN_POINT('Ctrl Pts',(73.1596213860029,9.49650203545229,57.9607224300517));
#165570=CARTESIAN_POINT('Ctrl Pts',(73.6905987997138,9.47758921615189,57.8616886448402));
#165571=CARTESIAN_POINT('Ctrl Pts',(74.1547034234038,9.42554973535961,57.7760402505727));
#165572=CARTESIAN_POINT('Ctrl Pts',(74.976701941755,9.269418330822,57.6241005958556));
#165573=CARTESIAN_POINT('Ctrl Pts',(75.3360069089991,9.17843376406987,57.5576039317642));
#165574=CARTESIAN_POINT('Ctrl Pts',(75.8226786152275,9.02344725629384,57.4669836179226));
#165575=CARTESIAN_POINT('Ctrl Pts',(75.9553995694799,8.97781831081514,57.4422141097941));
#165576=CARTESIAN_POINT('Ctrl Pts',(76.1871659049851,8.89217458746428,57.3988439013957));
#165577=CARTESIAN_POINT('Ctrl Pts',(76.2866456572561,8.85343931488086,57.3801900238829));
#165578=CARTESIAN_POINT('Ctrl Pts',(76.4336824453425,8.79322826421129,57.352557772604));
#165579=CARTESIAN_POINT('Ctrl Pts',(76.4817550428722,8.77306563835036,57.3435138373673));
#165580=CARTESIAN_POINT('Ctrl Pts',(76.5675866365434,8.73620838376513,57.3273484743898));
#165581=CARTESIAN_POINT('Ctrl Pts',(76.6054080296809,8.71966618636268,57.3202190156399));
#165582=CARTESIAN_POINT('Ctrl Pts',(76.6856813345046,8.68391360245852,57.3050738440368));
#165583=CARTESIAN_POINT('Ctrl Pts',(76.7281020312591,8.66463418988177,57.2970622928444));
#165584=CARTESIAN_POINT('Ctrl Pts',(76.8426614179813,8.61152008301531,57.2754048764274));
#165585=CARTESIAN_POINT('Ctrl Pts',(76.9145172207303,8.57706941804644,57.261796945921));
#165586=CARTESIAN_POINT('Ctrl Pts',(77.3325421105607,8.36996425748812,57.1824958930809));
#165587=CARTESIAN_POINT('Ctrl Pts',(77.6682672510631,8.17655306018609,57.1182350869084));
#165588=CARTESIAN_POINT('Ctrl Pts',(78.3312476390071,7.73726114210876,56.9905613950194));
#165589=CARTESIAN_POINT('Ctrl Pts',(78.6564104796808,7.48961277926842,56.92750984377));
#165590=CARTESIAN_POINT('Ctrl Pts',(79.0522314517669,7.14501840411167,56.8508670390811));
#165591=CARTESIAN_POINT('Ctrl Pts',(79.1383460244719,7.0671947692833,56.8342015903395));
#165592=CARTESIAN_POINT('Ctrl Pts',(79.2803633647217,6.9339911678635,56.8067593531978));
#165593=CARTESIAN_POINT('Ctrl Pts',(79.3370361894769,6.87948480197323,56.7958200432123));
#165594=CARTESIAN_POINT('Ctrl Pts',(79.4162520879116,6.80136525864896,56.7805534928331));
#165595=CARTESIAN_POINT('Ctrl Pts',(79.4393531020409,6.77834638070063,56.7761044202744));
#165596=CARTESIAN_POINT('Ctrl Pts',(79.4789944061098,6.73843429083015,56.7684756399244));
#165597=CARTESIAN_POINT('Ctrl Pts',(79.4955902603309,6.72159904241294,56.7652836436591));
#165598=CARTESIAN_POINT('Ctrl Pts',(79.5306951413774,6.68571922095411,56.7585357184119));
#165599=CARTESIAN_POINT('Ctrl Pts',(79.5491876312736,6.66665832687759,56.7549834124743));
#165600=CARTESIAN_POINT('Ctrl Pts',(79.5999882052794,6.61385237897887,56.7452307976009));
#165601=CARTESIAN_POINT('Ctrl Pts',(79.6321300693549,6.57994177901792,56.7390668921501));
#165602=CARTESIAN_POINT('Ctrl Pts',(79.8040858434861,6.39580631426493,56.7061201172949));
#165603=CARTESIAN_POINT('Ctrl Pts',(79.9393158075709,6.24120296649171,56.6803154441407));
#165604=CARTESIAN_POINT('Ctrl Pts',(80.3381543162808,5.75408163218469,56.6042483564325));
#165605=CARTESIAN_POINT('Ctrl Pts',(80.5847868217296,5.40786272369264,56.5572470308202));
#165606=CARTESIAN_POINT('Ctrl Pts',(80.9272043107022,4.85161065398208,56.4910595926873));
#165607=CARTESIAN_POINT('Ctrl Pts',(81.039838065784,4.65295149327204,56.4690996094166));
#165608=CARTESIAN_POINT('Ctrl Pts',(81.2151400404554,4.31602767871536,56.4344871328666));
#165609=CARTESIAN_POINT('Ctrl Pts',(81.2818261734697,4.18003010464455,56.4211983095346));
#165610=CARTESIAN_POINT('Ctrl Pts',(81.3703830547394,3.98797118853472,56.4033581788618));
#165611=CARTESIAN_POINT('Ctrl Pts',(81.3949950949096,3.93323980533567,56.3983772483707));
#165612=CARTESIAN_POINT('Ctrl Pts',(81.4362896825713,3.83904195294486,56.3899796958115));
#165613=CARTESIAN_POINT('Ctrl Pts',(81.4532248170859,3.7996917995099,56.3865235370366));
#165614=CARTESIAN_POINT('Ctrl Pts',(81.485044986955,3.72436107648079,56.3800056294664));
#165615=CARTESIAN_POINT('Ctrl Pts',(81.4999757761343,3.68840140854937,56.3769367318689));
#165616=CARTESIAN_POINT('Ctrl Pts',(81.5344447817902,3.60392884233406,56.3698267634644));
#165617=CARTESIAN_POINT('Ctrl Pts',(81.5538059317664,3.55534275064033,56.3658134551046));
#165618=CARTESIAN_POINT('Ctrl Pts',(81.6199209245155,3.38538030802865,56.3520386517122));
#165619=CARTESIAN_POINT('Ctrl Pts',(81.6646015774089,3.26318715824792,56.3426025471791));
#165620=CARTESIAN_POINT('Ctrl Pts',(81.9081947070157,2.55232658456308,56.2903944682411));
#165621=CARTESIAN_POINT('Ctrl Pts',(82.0519999541262,1.94575083504966,56.2562514419592));
#165622=CARTESIAN_POINT('Ctrl Pts',(82.1700432709274,1.08265002634678,56.2233954359544));
#165623=CARTESIAN_POINT('Ctrl Pts',(82.1942092311057,0.834886255511459,
56.215747290998));
#165624=CARTESIAN_POINT('Ctrl Pts',(82.2165188377026,0.454913275955093,
56.2069402107331));
#165625=CARTESIAN_POINT('Ctrl Pts',(82.221554786607,0.323249158030819,56.2044227986111));
#165626=CARTESIAN_POINT('Ctrl Pts',(82.2245833168324,0.153572390931381,
56.2018960425162));
#165627=CARTESIAN_POINT('Ctrl Pts',(82.2250378102207,0.115625620642261,
56.2013771506365));
#165628=CARTESIAN_POINT('Ctrl Pts',(82.2254136705754,0.0541009240409631,
56.2006116824008));
#165629=CARTESIAN_POINT('Ctrl Pts',(82.2254717611267,0.0305246054823433,
56.2003364058397));
#165630=CARTESIAN_POINT('Ctrl Pts',(82.2254412063335,0.00463207216118171,
56.2000540655189));
#165631=CARTESIAN_POINT('Ctrl Pts',(82.2254376442054,0.00231603550137483,
56.2000289862928));
#165632=CARTESIAN_POINT('Ctrl Pts',(82.2254332530441,4.44666969874771E-12,
56.2000040827795));
#165633=CARTESIAN_POINT('Origin',(73.0915550886457,-4.33680868994202E-16,
59.1075264962884));
#165634=CARTESIAN_POINT('',(82.1046676540618,-3.33476494482013E-11,55.5151083368357));
#165635=CARTESIAN_POINT('',(82.1125619375607,3.32220049501518E-11,55.5598790433222));
#165636=CARTESIAN_POINT('',(82.4472287422617,-1.59709532818419E-15,57.4578688084528));
#165637=CARTESIAN_POINT('Ctrl Pts',(82.1046676540618,-6.66937018010743E-11,
55.5151083368358));
#165638=CARTESIAN_POINT('Ctrl Pts',(82.1046831372505,0.0081663167848822,
55.515196146362));
#165639=CARTESIAN_POINT('Ctrl Pts',(82.1046881878999,0.0163326525156036,
55.5152854286388));
#165640=CARTESIAN_POINT('Ctrl Pts',(82.1046659042388,0.0501509387005742,
55.5156612874468));
#165641=CARTESIAN_POINT('Ctrl Pts',(82.1045460728912,0.0758025391846987,
55.5159609740892));
#165642=CARTESIAN_POINT('Ctrl Pts',(82.1039225209125,0.147615866527537,
55.5168413727629));
#165643=CARTESIAN_POINT('Ctrl Pts',(82.1031884526744,0.193774466373888,
55.5174551604751));
#165644=CARTESIAN_POINT('Ctrl Pts',(82.0967372734946,0.472792206847775,
55.521461835382));
#165645=CARTESIAN_POINT('Ctrl Pts',(82.0828777668914,0.705366327036288,
55.5260517536033));
#165646=CARTESIAN_POINT('Ctrl Pts',(82.0156816707158,1.40439261100474,55.5440290744549));
#165647=CARTESIAN_POINT('Ctrl Pts',(81.9366466032295,1.86753543376037,55.561621141297));
#165648=CARTESIAN_POINT('Ctrl Pts',(81.7431472263391,2.65152174651733,55.6026781636042));
#165649=CARTESIAN_POINT('Ctrl Pts',(81.6447761325593,2.97556669470496,55.6231139082363));
#165650=CARTESIAN_POINT('Ctrl Pts',(81.4965783113512,3.38477164741177,55.6536409687357));
#165651=CARTESIAN_POINT('Ctrl Pts',(81.4621677317308,3.47547154308474,55.6607140485646));
#165652=CARTESIAN_POINT('Ctrl Pts',(81.4077399467971,3.61263090299337,55.6718818724966));
#165653=CARTESIAN_POINT('Ctrl Pts',(81.388714192095,3.6594924557385,55.6757822735029));
#165654=CARTESIAN_POINT('Ctrl Pts',(81.3549112287724,3.74089876470706,55.6827064325909));
#165655=CARTESIAN_POINT('Ctrl Pts',(81.340298882702,3.77551346599158,55.6856978467158));
#165656=CARTESIAN_POINT('Ctrl Pts',(81.3068613116053,3.85344139111431,55.6925392419322));
#165657=CARTESIAN_POINT('Ctrl Pts',(81.2879194550937,3.89670145941487,55.6964121020932));
#165658=CARTESIAN_POINT('Ctrl Pts',(81.2356074432632,4.01381028176885,55.707100618256));
#165659=CARTESIAN_POINT('Ctrl Pts',(81.2016230747816,4.08736921194466,55.7140367123288));
#165660=CARTESIAN_POINT('Ctrl Pts',(80.9830923733534,4.54502939209053,55.7585882335667));
#165661=CARTESIAN_POINT('Ctrl Pts',(80.774191550578,4.91648662986971,55.800991498181));
#165662=CARTESIAN_POINT('Ctrl Pts',(80.3725625843288,5.53035930142778,55.8817279775636));
#165663=CARTESIAN_POINT('Ctrl Pts',(80.1914036554021,5.77981803456371,55.9179211194196));
#165664=CARTESIAN_POINT('Ctrl Pts',(79.9001286772755,6.14221806075194,55.9754595280785));
#165665=CARTESIAN_POINT('Ctrl Pts',(79.7987260380884,6.26211867664327,55.9953832139142));
#165666=CARTESIAN_POINT('Ctrl Pts',(79.6501945337465,6.42908120607563,56.0243646572932));
#165667=CARTESIAN_POINT('Ctrl Pts',(79.6054624396068,6.4783015434828,56.0330679262799));
#165668=CARTESIAN_POINT('Ctrl Pts',(79.5250902268847,6.56487146582401,56.0486563213353));
#165669=CARTESIAN_POINT('Ctrl Pts',(79.4896551364686,6.60241286861436,56.055512549177));
#165670=CARTESIAN_POINT('Ctrl Pts',(79.4348038664856,6.65957145977612,56.0660981355676));
#165671=CARTESIAN_POINT('Ctrl Pts',(79.415605311105,6.67940152823924,56.06979814269));
#165672=CARTESIAN_POINT('Ctrl Pts',(79.3799531745488,6.71590227784108,56.0766593775266));
#165673=CARTESIAN_POINT('Ctrl Pts',(79.3635239862352,6.73259679424968,56.0798173360737));
#165674=CARTESIAN_POINT('Ctrl Pts',(79.3256952573172,6.77074915242421,56.0870800326776));
#165675=CARTESIAN_POINT('Ctrl Pts',(79.3042544320404,6.7921645138499,56.0911902208889));
#165676=CARTESIAN_POINT('Ctrl Pts',(79.2349996431662,6.86066892745571,56.1044475115628));
#165677=CARTESIAN_POINT('Ctrl Pts',(79.1867885175033,6.90734310605114,56.1136479282141));
#165678=CARTESIAN_POINT('Ctrl Pts',(78.8976964697032,7.18126229419028,56.1686706934064));
#165679=CARTESIAN_POINT('Ctrl Pts',(78.645559001247,7.39596465874361,56.2160723888613));
#165680=CARTESIAN_POINT('Ctrl Pts',(78.1619015270093,7.76544087215151,56.3066664954445));
#165681=CARTESIAN_POINT('Ctrl Pts',(77.933738825979,7.9241295867861,56.3492802804894));
#165682=CARTESIAN_POINT('Ctrl Pts',(77.5149074666914,8.18850050147076,56.4275886032426));
#165683=CARTESIAN_POINT('Ctrl Pts',(77.3268952595357,8.29815221108524,56.4627679327325));
#165684=CARTESIAN_POINT('Ctrl Pts',(77.0067828052513,8.47009189980756,56.5227972191076));
#165685=CARTESIAN_POINT('Ctrl Pts',(76.8766863766069,8.53606849880377,56.5472281349927));
#165686=CARTESIAN_POINT('Ctrl Pts',(76.6921247735683,8.62426000440992,56.5819482073274));
#165687=CARTESIAN_POINT('Ctrl Pts',(76.6388805668218,8.64908349941913,56.5919715400614));
#165688=CARTESIAN_POINT('Ctrl Pts',(76.5469519373623,8.69088307927248,56.6092898055402));
#165689=CARTESIAN_POINT('Ctrl Pts',(76.5083770192802,8.70810549192532,56.616560609147));
#165690=CARTESIAN_POINT('Ctrl Pts',(76.4343297779943,8.74055935311842,56.6305247489454));
#165691=CARTESIAN_POINT('Ctrl Pts',(76.3988766978219,8.75583431961461,56.6372138274678));
#165692=CARTESIAN_POINT('Ctrl Pts',(76.3152861227901,8.79123101965565,56.6529927835154));
#165693=CARTESIAN_POINT('Ctrl Pts',(76.2670746326234,8.81116716675332,56.6620992907729));
#165694=CARTESIAN_POINT('Ctrl Pts',(76.0977892732844,8.87949795525368,56.6940956311411));
#165695=CARTESIAN_POINT('Ctrl Pts',(75.9758933647215,8.92572653882055,56.7171718631662));
#165696=CARTESIAN_POINT('Ctrl Pts',(75.2776492345973,9.17375978534379,56.8495538811731));
#165697=CARTESIAN_POINT('Ctrl Pts',(74.6840739425484,9.32031763958669,56.9629710726892));
#165698=CARTESIAN_POINT('Ctrl Pts',(73.8391287839856,9.44160111273542,57.1239553230159));
#165699=CARTESIAN_POINT('Ctrl Pts',(73.5963183040112,9.46662071876087,57.1701471231172));
#165700=CARTESIAN_POINT('Ctrl Pts',(73.2237691952166,9.49003939628665,57.2406995557542));
#165701=CARTESIAN_POINT('Ctrl Pts',(73.0945879536231,9.49542146990205,57.2651043896395));
#165702=CARTESIAN_POINT('Ctrl Pts',(72.928053995339,9.49883599086951,57.2964588184468));
#165703=CARTESIAN_POINT('Ctrl Pts',(72.8907787502528,9.4993730333388,57.3034699553758));
#165704=CARTESIAN_POINT('Ctrl Pts',(72.8303327293459,9.49987551265791,57.3148271185292));
#165705=CARTESIAN_POINT('Ctrl Pts',(72.807164317804,9.49998036921824,57.3191773133001));
#165706=CARTESIAN_POINT('Ctrl Pts',(72.7621527105507,9.50001363679289,57.3276229509993));
#165707=CARTESIAN_POINT('Ctrl Pts',(72.740309809437,9.49995180678593,57.3317186564709));
#165708=CARTESIAN_POINT('Ctrl Pts',(72.6915203269276,9.49963953831488,57.3408612233654));
#165709=CARTESIAN_POINT('Ctrl Pts',(72.6645738958548,9.49934840727279,57.3459067001559));
#165710=CARTESIAN_POINT('Ctrl Pts',(72.5712792404284,9.49792957809917,57.3633624175714));
#165711=CARTESIAN_POINT('Ctrl Pts',(72.5049384604776,9.49620114058441,57.3757524555154));
#165712=CARTESIAN_POINT('Ctrl Pts',(72.0593651423265,9.47975728250069,57.4588421737555));
#165713=CARTESIAN_POINT('Ctrl Pts',(71.6811945947327,9.44226038275326,57.5287569015261));
#165714=CARTESIAN_POINT('Ctrl Pts',(70.9739692781486,9.3275776154078,57.6594673389788));
#165715=CARTESIAN_POINT('Ctrl Pts',(70.6447295853202,9.25546248748561,57.7203015539361));
#165716=CARTESIAN_POINT('Ctrl Pts',(70.1224736982051,9.11064479072532,57.8172237670461));
#165717=CARTESIAN_POINT('Ctrl Pts',(69.9267089411425,9.0492544918558,57.8536510059286));
#165718=CARTESIAN_POINT('Ctrl Pts',(69.5992900501307,8.93444408773968,57.9148035215196));
#165719=CARTESIAN_POINT('Ctrl Pts',(69.4665475187724,8.88443107039321,57.9396606190141));
#165720=CARTESIAN_POINT('Ctrl Pts',(69.2810064387629,8.80959638202293,57.9745055375095));
#165721=CARTESIAN_POINT('Ctrl Pts',(69.2272295146504,8.7873127720697,57.9846170245872));
#165722=CARTESIAN_POINT('Ctrl Pts',(69.1348783782127,8.74801777648703,58.0020027698529));
#165723=CARTESIAN_POINT('Ctrl Pts',(69.0962053286749,8.73124896084119,58.0092897352786));
#165724=CARTESIAN_POINT('Ctrl Pts',(69.0222280031529,8.69856865200554,58.0232414644762));
#165725=CARTESIAN_POINT('Ctrl Pts',(68.9869066647666,8.68269892143716,58.0299084195651));
#165726=CARTESIAN_POINT('Ctrl Pts',(68.903793248601,8.64472670475603,58.0456093004335));
#165727=CARTESIAN_POINT('Ctrl Pts',(68.8560864770542,8.62243607656902,58.0546318394442));
#165728=CARTESIAN_POINT('Ctrl Pts',(68.6880416112906,8.54216209003482,58.0864495549736));
#165729=CARTESIAN_POINT('Ctrl Pts',(68.5687505773935,8.48196965267659,58.1091026585753));
#165730=CARTESIAN_POINT('Ctrl Pts',(67.8620360902405,8.10595933642776,58.2436841110684));
#165731=CARTESIAN_POINT('Ctrl Pts',(67.3081640330838,7.72964916123593,58.3509193445901));
#165732=CARTESIAN_POINT('Ctrl Pts',(66.6919868223647,7.20644801995258,58.4702599631192));
#165733=CARTESIAN_POINT('Ctrl Pts',(66.5877223417527,7.11383692795435,58.4904483094891));
#165734=CARTESIAN_POINT('Ctrl Pts',(66.4197861244975,6.95784719479171,58.5229115247445));
#165735=CARTESIAN_POINT('Ctrl Pts',(66.3549175998932,6.89584140615282,58.5354372139019));
#165736=CARTESIAN_POINT('Ctrl Pts',(66.2664560913634,6.80883177659919,58.5524884106032));
#165737=CARTESIAN_POINT('Ctrl Pts',(66.2421150705354,6.78462733301814,58.5571769721059));
#165738=CARTESIAN_POINT('Ctrl Pts',(66.2010356331124,6.74333005224545,58.5650833981811));
#165739=CARTESIAN_POINT('Ctrl Pts',(66.1842304851331,6.72630683448447,58.5683160154738));
#165740=CARTESIAN_POINT('Ctrl Pts',(66.1494220374238,6.6907776199164,58.5750076626894));
#165741=CARTESIAN_POINT('Ctrl Pts',(66.1314294404848,6.67226116211173,58.5784643550833));
#165742=CARTESIAN_POINT('Ctrl Pts',(66.0834453141416,6.62247302469418,58.587677477598));
#165743=CARTESIAN_POINT('Ctrl Pts',(66.0535898977672,6.5910655260915,58.5934040525778));
#165744=CARTESIAN_POINT('Ctrl Pts',(65.9159484399966,6.44425865080944,58.6197826292321));
#165745=CARTESIAN_POINT('Ctrl Pts',(65.8107995817224,6.32632082078509,58.6398697160837));
#165746=CARTESIAN_POINT('Ctrl Pts',(65.447187312382,5.89730224878749,58.7092560063207));
#165747=CARTESIAN_POINT('Ctrl Pts',(65.2055034651842,5.5720571763071,58.7552481396823));
#165748=CARTESIAN_POINT('Ctrl Pts',(64.7808138047891,4.91669049455642,58.8369564969829));
#165749=CARTESIAN_POINT('Ctrl Pts',(64.5952023813503,4.58922749354895,58.8731033986191));
#165750=CARTESIAN_POINT('Ctrl Pts',(64.3849917464723,4.16100425652833,58.9149934297197));
#165751=CARTESIAN_POINT('Ctrl Pts',(64.3420553102035,4.06991394828237,58.9236086251639));
#165752=CARTESIAN_POINT('Ctrl Pts',(64.2794368460239,3.93141580287353,58.9362687519412));
#165753=CARTESIAN_POINT('Ctrl Pts',(64.258685942999,3.8845146726464,58.9404811439993));
#165754=CARTESIAN_POINT('Ctrl Pts',(64.2217726030343,3.79922974446169,58.9480062209492));
#165755=CARTESIAN_POINT('Ctrl Pts',(64.2054818540183,3.76090469970925,58.951338978688));
#165756=CARTESIAN_POINT('Ctrl Pts',(64.1709011699647,3.67804817051531,58.9584393886893));
#165757=CARTESIAN_POINT('Ctrl Pts',(64.1526958543573,3.63348150617339,58.9621937671403));
#165758=CARTESIAN_POINT('Ctrl Pts',(64.1040270418712,3.51171581159866,58.9722758391137));
#165759=CARTESIAN_POINT('Ctrl Pts',(64.0742290339685,3.43424684793218,58.9784991616309));
#165760=CARTESIAN_POINT('Ctrl Pts',(63.8821866410214,2.91486465460458,59.0189543440854));
#165761=CARTESIAN_POINT('Ctrl Pts',(63.7516782296472,2.46153848179776,59.0482232182268));
#165762=CARTESIAN_POINT('Ctrl Pts',(63.5850256595648,1.66677409635791,59.0888193295504));
#165763=CARTESIAN_POINT('Ctrl Pts',(63.5328667405273,1.32975184675359,59.1028295217104));
#165764=CARTESIAN_POINT('Ctrl Pts',(63.4732790652233,0.739351186250466,
59.1213514861095));
#165765=CARTESIAN_POINT('Ctrl Pts',(63.4577808905696,0.487180544235924,
59.1273738831734));
#165766=CARTESIAN_POINT('Ctrl Pts',(63.451130350729,0.188969836213798,59.1320893438065));
#165767=CARTESIAN_POINT('Ctrl Pts',(63.4504344815118,0.143273027569161,
59.1327452370923));
#165768=CARTESIAN_POINT('Ctrl Pts',(63.44985533765,0.0723001197369106,59.1336587975064));
#165769=CARTESIAN_POINT('Ctrl Pts',(63.4497478738907,0.0470271383427463,
59.1339634119294));
#165770=CARTESIAN_POINT('Ctrl Pts',(63.4497315844953,-0.000111857181628876,
59.1344926467005));
#165771=CARTESIAN_POINT('Ctrl Pts',(63.4497979227852,-0.0219774458935335,
59.1347224763209));
#165772=CARTESIAN_POINT('Ctrl Pts',(63.4501207371716,-0.0723079847418672,
59.1352156021532));
#165773=CARTESIAN_POINT('Ctrl Pts',(63.4504285637723,-0.100772441046243,
59.1354680870719));
#165774=CARTESIAN_POINT('Ctrl Pts',(63.4518247001461,-0.192520906325654,
59.1361976654566));
#165775=CARTESIAN_POINT('Ctrl Pts',(63.4534070938291,-0.255796486702477,
59.1365716201473));
#165776=CARTESIAN_POINT('Ctrl Pts',(63.4734969926213,-0.832898076404157,
59.1388295792473));
#165777=CARTESIAN_POINT('Ctrl Pts',(63.532248671359,-1.34450388879123,59.1325340977909));
#165778=CARTESIAN_POINT('Ctrl Pts',(63.6993547987218,-2.19348172572141,
59.1102140452665));
#165779=CARTESIAN_POINT('Ctrl Pts',(63.7859840566445,-2.53407443213869,
59.0979090671673));
#165780=CARTESIAN_POINT('Ctrl Pts',(63.9523549740527,-3.06450153426549,
59.0737571105813));
#165781=CARTESIAN_POINT('Ctrl Pts',(64.0198954654271,-3.25790799180822,
59.0638571323772));
#165782=CARTESIAN_POINT('Ctrl Pts',(64.1177203463775,-3.5115913955153,59.0494341331305));
#165783=CARTESIAN_POINT('Ctrl Pts',(64.1425305199046,-3.57396758640219,
59.0457698072429));
#165784=CARTESIAN_POINT('Ctrl Pts',(64.1847994231312,-3.67706542313569,
59.0395171815474));
#165785=CARTESIAN_POINT('Ctrl Pts',(64.2018896681755,-3.71793896794379,
59.0369866118446));
#165786=CARTESIAN_POINT('Ctrl Pts',(64.2358664409931,-3.79763866887981,
59.0319509276408));
#165787=CARTESIAN_POINT('Ctrl Pts',(64.2527281633351,-3.83647451939185,
59.0294496941545));
#165788=CARTESIAN_POINT('Ctrl Pts',(64.2938328790742,-3.92945162299446,
59.0233471949904));
#165789=CARTESIAN_POINT('Ctrl Pts',(64.318321969458,-3.98347956943434,59.0197073794883));
#165790=CARTESIAN_POINT('Ctrl Pts',(64.4005075619662,-4.16039963263101,
59.0074785224434));
#165791=CARTESIAN_POINT('Ctrl Pts',(64.4603109116928,-4.28227123182679,
58.9985590624346));
#165792=CARTESIAN_POINT('Ctrl Pts',(64.8302564832783,-4.99722774000309,
58.9432396329212));
#165793=CARTESIAN_POINT('Ctrl Pts',(65.1991912428121,-5.55704924364375,
58.8876724094771));
#165794=CARTESIAN_POINT('Ctrl Pts',(65.713789053458,-6.18341508401888,58.8076088935999));
#165795=CARTESIAN_POINT('Ctrl Pts',(65.807055753738,-6.29185438975616,58.7930065567522));
#165796=CARTESIAN_POINT('Ctrl Pts',(65.9638401994224,-6.46603793241588,
58.7682668419714));
#165797=CARTESIAN_POINT('Ctrl Pts',(66.0259450869616,-6.53306410259867,
58.7584201202982));
#165798=CARTESIAN_POINT('Ctrl Pts',(66.1128893669043,-6.62422429119724,
58.7445602906985));
#165799=CARTESIAN_POINT('Ctrl Pts',(66.136921722301,-6.64914757106302,58.7407215974516));
#165800=CARTESIAN_POINT('Ctrl Pts',(66.1778565703575,-6.69113787880428,
58.7341693510924));
#165801=CARTESIAN_POINT('Ctrl Pts',(66.1946897427538,-6.70827445305186,
58.7314710617903));
#165802=CARTESIAN_POINT('Ctrl Pts',(66.2297466646922,-6.7436933071832,58.7258432743214));
#165803=CARTESIAN_POINT('Ctrl Pts',(66.2479800694958,-6.76196523509998,
58.7229116486028));
#165804=CARTESIAN_POINT('Ctrl Pts',(66.2968630664495,-6.81055323044644,
58.7150404917573));
#165805=CARTESIAN_POINT('Ctrl Pts',(66.3276428317794,-6.84073279924547,
58.7100722633174));
#165806=CARTESIAN_POINT('Ctrl Pts',(66.4697229047843,-6.97815348490206,
58.6870882135298));
#165807=CARTESIAN_POINT('Ctrl Pts',(66.5833881581997,-7.08282897644763,
58.6685600972062));
#165808=CARTESIAN_POINT('Ctrl Pts',(67.0598541869205,-7.50048208756614,
58.5904995629257));
#165809=CARTESIAN_POINT('Ctrl Pts',(67.443275480518,-7.78804695485937,58.5268146046099));
#165810=CARTESIAN_POINT('Ctrl Pts',(68.0396253335662,-8.16769251134123,
58.4279738930985));
#165811=CARTESIAN_POINT('Ctrl Pts',(68.2369862389141,-8.28338278802693,
58.3952868361985));
#165812=CARTESIAN_POINT('Ctrl Pts',(68.5714886110786,-8.46328341855298,
58.3400288204572));
#165813=CARTESIAN_POINT('Ctrl Pts',(68.706342788626,-8.53163420263656,58.3177878010472));
#165814=CARTESIAN_POINT('Ctrl Pts',(68.8966402770467,-8.6223335520558,58.2864672673073));
#165815=CARTESIAN_POINT('Ctrl Pts',(68.95074948605,-8.64748745445042,58.2775686487063));
#165816=CARTESIAN_POINT('Ctrl Pts',(69.0438255446409,-8.68967224322549,
58.262274386077));
#165817=CARTESIAN_POINT('Ctrl Pts',(69.0826762131982,-8.70696044170122,
58.2558941936876));
#165818=CARTESIAN_POINT('Ctrl Pts',(69.1570157440917,-8.73943209192528,
58.2436932119723));
#165819=CARTESIAN_POINT('Ctrl Pts',(69.1924836493893,-8.75466234255305,
58.2378751893835));
#165820=CARTESIAN_POINT('Ctrl Pts',(69.2757473516295,-8.78980424494869,
58.2242243807533));
#165821=CARTESIAN_POINT('Ctrl Pts',(69.3236153746011,-8.80953781953575,
58.2163822968633));
#165822=CARTESIAN_POINT('Ctrl Pts',(69.4897749866052,-8.87641871399374,
58.1891806589193));
#165823=CARTESIAN_POINT('Ctrl Pts',(69.6088545500402,-8.92152877525408,
58.1697211654617));
#165824=CARTESIAN_POINT('Ctrl Pts',(70.3101291570692,-9.17082972819739,
58.0553132013703));
#165825=CARTESIAN_POINT('Ctrl Pts',(70.9102826091913,-9.31893795512639,
57.9582944622942));
#165826=CARTESIAN_POINT('Ctrl Pts',(71.764016064951,-9.44127115823504,57.819824825256));
#165827=CARTESIAN_POINT('Ctrl Pts',(72.0089382817627,-9.46645823239192,
57.7800306574467));
#165828=CARTESIAN_POINT('Ctrl Pts',(72.3844319472909,-9.49000379832992,
57.71870062551));
#165829=CARTESIAN_POINT('Ctrl Pts',(72.5144890092581,-9.49540850518504,
57.6973990288106));
#165830=CARTESIAN_POINT('Ctrl Pts',(72.6820546923221,-9.49883357520942,
57.6698469575177));
#165831=CARTESIAN_POINT('Ctrl Pts',(72.7195112113965,-9.49937163194484,
57.6636812529279));
#165832=CARTESIAN_POINT('Ctrl Pts',(72.7802344656364,-9.49987503546522,
57.6536734635712));
#165833=CARTESIAN_POINT('Ctrl Pts',(72.8035004016127,-9.49998013002439,
57.6498361156224));
#165834=CARTESIAN_POINT('Ctrl Pts',(72.8486888084411,-9.50001375096868,
57.6423771003517));
#165835=CARTESIAN_POINT('Ctrl Pts',(72.8706110917601,-9.49995211783509,
57.6387557832221));
#165836=CARTESIAN_POINT('Ctrl Pts',(72.9195649160004,-9.49964042486989,
57.6306633598357));
#165837=CARTESIAN_POINT('Ctrl Pts',(72.9465958440896,-9.4993497841532,57.6261910072101));
#165838=CARTESIAN_POINT('Ctrl Pts',(73.0401252756043,-9.49793394946541,
57.6107034682325));
#165839=CARTESIAN_POINT('Ctrl Pts',(73.1066099269781,-9.49620988285458,
57.5996718911103));
#165840=CARTESIAN_POINT('Ctrl Pts',(73.5497324598121,-9.47993281031314,
57.5260206290239));
#165841=CARTESIAN_POINT('Ctrl Pts',(73.9251347111281,-9.44307601256934,
57.4630331891849));
#165842=CARTESIAN_POINT('Ctrl Pts',(74.6182284293805,-9.33194263293071,
57.3466939766465));
#165843=CARTESIAN_POINT('Ctrl Pts',(74.9362728467005,-9.26359772317145,
57.29328888963));
#165844=CARTESIAN_POINT('Ctrl Pts',(75.5643524840488,-9.09362735020921,
57.1882896720197));
#165845=CARTESIAN_POINT('Ctrl Pts',(75.8739539255729,-8.99209655483669,
57.1367692950126));
#165846=CARTESIAN_POINT('Ctrl Pts',(76.2493713887129,-8.84674209398468,
57.0747537356981));
#165847=CARTESIAN_POINT('Ctrl Pts',(76.3206236207922,-8.81813636116631,
57.0630038745012));
#165848=CARTESIAN_POINT('Ctrl Pts',(76.434073051199,-8.77095282666222,57.0443292166408));
#165849=CARTESIAN_POINT('Ctrl Pts',(76.4764930731016,-8.75294016323587,
57.0373541744268));
#165850=CARTESIAN_POINT('Ctrl Pts',(76.5569017188852,-8.71809049907456,
57.0241473977026));
#165851=CARTESIAN_POINT('Ctrl Pts',(76.5949140495991,-8.70131304058684,
57.0179103189341));
#165852=CARTESIAN_POINT('Ctrl Pts',(76.681585926515,-8.66236474551072,57.0037035963794));
#165853=CARTESIAN_POINT('Ctrl Pts',(76.7301717221771,-8.64002748184918,
56.9957501951603));
#165854=CARTESIAN_POINT('Ctrl Pts',(76.8575062155302,-8.58015464658321,
56.9749333050698));
#165855=CARTESIAN_POINT('Ctrl Pts',(76.9359347137147,-8.54192645023717,
56.9621396337513));
#165856=CARTESIAN_POINT('Ctrl Pts',(77.5027763721314,-8.25573693285314,
56.8698722743975));
#165857=CARTESIAN_POINT('Ctrl Pts',(77.9696845222031,-7.96606661635586,
56.7950366509687));
#165858=CARTESIAN_POINT('Ctrl Pts',(78.7086770974681,-7.412474549301,56.6773091172826));
#165859=CARTESIAN_POINT('Ctrl Pts',(78.9948260910236,-7.17017542567809,
56.631910123448));
#165860=CARTESIAN_POINT('Ctrl Pts',(79.3051312050996,-6.87385812327918,
56.5823445978682));
#165861=CARTESIAN_POINT('Ctrl Pts',(79.3440108968386,-6.83608389584711,
56.5761275783788));
#165862=CARTESIAN_POINT('Ctrl Pts',(79.4026074612306,-6.77816131282105,
56.5667448560018));
#165863=CARTESIAN_POINT('Ctrl Pts',(79.4225611359854,-6.75825927064249,
56.5635474787788));
#165864=CARTESIAN_POINT('Ctrl Pts',(79.4589415917199,-6.72164567551471,
56.5577131659297));
#165865=CARTESIAN_POINT('Ctrl Pts',(79.4753954821686,-6.70496226249003,
56.5550726376095));
#165866=CARTESIAN_POINT('Ctrl Pts',(79.5129227598308,-6.66662639344478,
56.5490461415989));
#165867=CARTESIAN_POINT('Ctrl Pts',(79.5339549054514,-6.64493327170735,
56.5456656563551));
#165868=CARTESIAN_POINT('Ctrl Pts',(79.5996144994989,-6.57655524275546,
56.5351039944811));
#165869=CARTESIAN_POINT('Ctrl Pts',(79.6438705318666,-6.52950854742274,
56.5279731602701));
#165870=CARTESIAN_POINT('Ctrl Pts',(79.9855428791404,-6.15873494632548,
56.4728501572721));
#165871=CARTESIAN_POINT('Ctrl Pts',(80.260728051821,-5.81478797497322,56.4280549634609));
#165872=CARTESIAN_POINT('Ctrl Pts',(80.7938629293535,-5.04443120862511,
56.3421351942791));
#165873=CARTESIAN_POINT('Ctrl Pts',(81.0443246187931,-4.61429916332988,
56.3023587383068));
#165874=CARTESIAN_POINT('Ctrl Pts',(81.2962839137847,-4.09212441356338,
56.263880837066));
#165875=CARTESIAN_POINT('Ctrl Pts',(81.3311071477423,-4.01751901645962,
56.2586031812913));
#165876=CARTESIAN_POINT('Ctrl Pts',(81.3845258927951,-3.89912838455132,
56.2505745858118));
#165877=CARTESIAN_POINT('Ctrl Pts',(81.4037593434249,-3.85564413146906,
56.2476985052862));
#165878=CARTESIAN_POINT('Ctrl Pts',(81.439283128616,-3.77369193169898,56.2424146519987));
#165879=CARTESIAN_POINT('Ctrl Pts',(81.4556465687234,-3.73525785157648,
56.2399925163393));
#165880=CARTESIAN_POINT('Ctrl Pts',(81.4919254014947,-3.64848326151286,
56.2346495645819));
#165881=CARTESIAN_POINT('Ctrl Pts',(81.5116987919796,-3.6000831566221,56.2317565795328));
#165882=CARTESIAN_POINT('Ctrl Pts',(81.5701357584086,-3.45364820506756,
56.223265848742));
#165883=CARTESIAN_POINT('Ctrl Pts',(81.6075896679452,-3.35512585625018,
56.2179050820122));
#165884=CARTESIAN_POINT('Ctrl Pts',(81.8441821977068,-2.70062994864765,
56.1845966892776));
#165885=CARTESIAN_POINT('Ctrl Pts',(81.9936263514858,-2.12757611206901,
56.1664208804195));
#165886=CARTESIAN_POINT('Ctrl Pts',(82.1596767102879,-1.11909655564106,
56.151342744878));
#165887=CARTESIAN_POINT('Ctrl Pts',(82.2011112941517,-0.689618758341124,
56.1499948221716));
#165888=CARTESIAN_POINT('Ctrl Pts',(82.215011841021,-0.208411550980801,
56.1532962934307));
#165889=CARTESIAN_POINT('Ctrl Pts',(82.2160710233358,-0.157971248743679,
56.1537009227633));
#165890=CARTESIAN_POINT('Ctrl Pts',(82.217076659079,-0.081253318392736,
56.1544033351846));
#165891=CARTESIAN_POINT('Ctrl Pts',(82.2173131050438,-0.0549800076835477,
56.1546593992613));
#165892=CARTESIAN_POINT('Ctrl Pts',(82.2174883617966,-0.0191374724957702,
56.1550296195407));
#165893=CARTESIAN_POINT('Ctrl Pts',(82.2175208274001,-0.00956873354244861,
56.1551304870759));
#165894=CARTESIAN_POINT('Ctrl Pts',(82.2175389695453,-7.70179830244106E-11,
56.1552333762936));
#165895=CARTESIAN_POINT('Ctrl Pts',(82.2254332530441,4.44666969874771E-12,
56.2000040827795));
#165896=CARTESIAN_POINT('Ctrl Pts',(82.2253955162052,-0.0199035864588712,
56.1997900665309));
#165897=CARTESIAN_POINT('Ctrl Pts',(82.2252965522329,-0.0398070870381526,
56.1995890272647));
#165898=CARTESIAN_POINT('Ctrl Pts',(82.2249157684035,-0.0871137839519527,
56.1991418195417));
#165899=CARTESIAN_POINT('Ctrl Pts',(82.2245790953923,-0.114516504828974,
56.1989071958335));
#165900=CARTESIAN_POINT('Ctrl Pts',(82.2230119138865,-0.209353958669355,
56.1981789048622));
#165901=CARTESIAN_POINT('Ctrl Pts',(82.2211941976636,-0.276777880483236,
56.1978076317294));
#165902=CARTESIAN_POINT('Ctrl Pts',(82.204333910507,-0.727478752833875,
56.196282364896));
#165903=CARTESIAN_POINT('Ctrl Pts',(82.1672510969061,-1.10959181644738,
56.1996048160965));
#165904=CARTESIAN_POINT('Ctrl Pts',(82.0557041387056,-1.81713780611838,
56.2133622885313));
#165905=CARTESIAN_POINT('Ctrl Pts',(81.9869103648884,-2.14289188473711,
56.2227894455887));
#165906=CARTESIAN_POINT('Ctrl Pts',(81.8178229056863,-2.77840528625268,
56.2468536484031));
#165907=CARTESIAN_POINT('Ctrl Pts',(81.7183993652482,-3.08793791222269,
56.2613499728732));
#165908=CARTESIAN_POINT('Ctrl Pts',(81.5761387521535,-3.46400593713413,
56.2823008088395));
#165909=CARTESIAN_POINT('Ctrl Pts',(81.5479180886168,-3.5359623843275,56.2864656992188));
#165910=CARTESIAN_POINT('Ctrl Pts',(81.5013383007465,-3.65062476754098,
56.2933527663705));
#165911=CARTESIAN_POINT('Ctrl Pts',(81.4835323305294,-3.69355676183597,
56.2959882599742));
#165912=CARTESIAN_POINT('Ctrl Pts',(81.4490588683304,-3.77499364385461,
56.3010958269628));
#165913=CARTESIAN_POINT('Ctrl Pts',(81.432449278758,-3.8135224077732,56.3035588362739));
#165914=CARTESIAN_POINT('Ctrl Pts',(81.3938545960449,-3.90145308925757,
56.3092867861315));
#165915=CARTESIAN_POINT('Ctrl Pts',(81.3717035388202,-3.9507788578324,56.3125777225235));
#165916=CARTESIAN_POINT('Ctrl Pts',(81.3122469461368,-4.08022628791294,
56.3214201090177));
#165917=CARTESIAN_POINT('Ctrl Pts',(81.2742493685627,-4.16001674333413,
56.3270800786198));
#165918=CARTESIAN_POINT('Ctrl Pts',(80.9929389801881,-4.73022065043414,
56.3690516585816));
#165919=CARTESIAN_POINT('Ctrl Pts',(80.7091515037419,-5.1990457639627,56.411670866996));
#165920=CARTESIAN_POINT('Ctrl Pts',(80.1632985133085,-5.94727017028107,
56.4953519264619));
#165921=CARTESIAN_POINT('Ctrl Pts',(79.9215006325915,-6.24016071407357,
56.5328718526995));
#165922=CARTESIAN_POINT('Ctrl Pts',(79.6260668652627,-6.55733592235234,
56.5797659783561));
#165923=CARTESIAN_POINT('Ctrl Pts',(79.5886785386282,-6.59679099859632,
56.5857185875736));
#165924=CARTESIAN_POINT('Ctrl Pts',(79.5313772010698,-6.6562294461383,56.5948712450172));
#165925=CARTESIAN_POINT('Ctrl Pts',(79.5117063169185,-6.6764527770008,56.5980184681503));
#165926=CARTESIAN_POINT('Ctrl Pts',(79.4755347925571,-6.71331003224424,
56.6038156651583));
#165927=CARTESIAN_POINT('Ctrl Pts',(79.4590618219615,-6.72997143915911,
56.606459565508));
#165928=CARTESIAN_POINT('Ctrl Pts',(79.4212306585479,-6.76795298820711,
56.6125399695534));
#165929=CARTESIAN_POINT('Ctrl Pts',(79.3998329159405,-6.78923176041793,
56.6159852278508));
#165930=CARTESIAN_POINT('Ctrl Pts',(79.3324587409256,-6.85559469885949,
56.6268512048442));
#165931=CARTESIAN_POINT('Ctrl Pts',(79.2861306689006,-6.90030655555888,
56.6343489896785));
#165932=CARTESIAN_POINT('Ctrl Pts',(78.9146862544009,-7.2515465451748,56.694644277855));
#165933=CARTESIAN_POINT('Ctrl Pts',(78.5690707915128,-7.53481074161679,
56.7518050996022));
#165934=CARTESIAN_POINT('Ctrl Pts',(77.8076719151865,-8.07302690735746,
56.8779693187153));
#165935=CARTESIAN_POINT('Ctrl Pts',(77.3895128398198,-8.32222894540669,
56.9473698915649));
#165936=CARTESIAN_POINT('Ctrl Pts',(76.8809355490933,-8.57375966340547,
57.0311738505378));
#165937=CARTESIAN_POINT('Ctrl Pts',(76.8072632540691,-8.60899784913653,
57.0433010510237));
#165938=CARTESIAN_POINT('Ctrl Pts',(76.6903687544093,-8.66303131409896,
57.0625213902721));
#165939=CARTESIAN_POINT('Ctrl Pts',(76.6474457059946,-8.68247781399196,
57.06957445866));
#165940=CARTESIAN_POINT('Ctrl Pts',(76.566561211271,-8.71838489330554,57.0828565240553));
#165941=CARTESIAN_POINT('Ctrl Pts',(76.5286334552846,-8.73492015715773,
57.0890810567793));
#165942=CARTESIAN_POINT('Ctrl Pts',(76.4430160384094,-8.77156866829192,
57.1031239821759));
#165943=CARTESIAN_POINT('Ctrl Pts',(76.395267320709,-8.79153750841962,57.1109500011659));
#165944=CARTESIAN_POINT('Ctrl Pts',(76.2508549171489,-8.85052004741923,
57.1346019131531));
#165945=CARTESIAN_POINT('Ctrl Pts',(76.1537081368881,-8.88830405527304,
57.1504893590829));
#165946=CARTESIAN_POINT('Ctrl Pts',(75.5067039672198,-9.12749706667559,
57.2561516370138));
#165947=CARTESIAN_POINT('Ctrl Pts',(74.9397802215985,-9.27805352121886,
57.3479215953453));
#165948=CARTESIAN_POINT('Ctrl Pts',(73.9439667610207,-9.44389509369572,
57.5093074319521));
#165949=CARTESIAN_POINT('Ctrl Pts',(73.5210000827707,-9.48476412561141,
57.5779457722092));
#165950=CARTESIAN_POINT('Ctrl Pts',(73.047144466932,-9.4978486805272,57.6557592949775));
#165951=CARTESIAN_POINT('Ctrl Pts',(72.9973819656997,-9.49882102592703,
57.6639425322809));
#165952=CARTESIAN_POINT('Ctrl Pts',(72.9216943573471,-9.49968903325272,
57.6764087503415));
#165953=CARTESIAN_POINT('Ctrl Pts',(72.8957718895608,-9.49987734448565,
57.680681856886));
#165954=CARTESIAN_POINT('Ctrl Pts',(72.8483832736218,-9.50002237968127,
57.6885002767504));
#165955=CARTESIAN_POINT('Ctrl Pts',(72.8269174283608,-9.50001334844315,
57.692044405234));
#165956=CARTESIAN_POINT('Ctrl Pts',(72.7782415360183,-9.49982340758179,
57.7000868573998));
#165957=CARTESIAN_POINT('Ctrl Pts',(72.7510322551577,-9.49959714264678,
57.704586564061));
#165958=CARTESIAN_POINT('Ctrl Pts',(72.680143022119,-9.49869473362846,57.7163197378305));
#165959=CARTESIAN_POINT('Ctrl Pts',(72.636467052151,-9.49782915050843,57.7235585642748));
#165960=CARTESIAN_POINT('Ctrl Pts',(72.2488883797173,-9.48739972769602,
57.7878738130109));
#165961=CARTESIAN_POINT('Ctrl Pts',(71.9058274434864,-9.4589580807626,57.845340194433));
#165962=CARTESIAN_POINT('Ctrl Pts',(70.9881031441345,-9.33101752781764,
57.9993182455476));
#165963=CARTESIAN_POINT('Ctrl Pts',(70.4197804593559,-9.19619900314946,
58.0948653460216));
#165964=CARTESIAN_POINT('Ctrl Pts',(69.7159478974758,-8.95740017155845,
58.2117748411039));
#165965=CARTESIAN_POINT('Ctrl Pts',(69.5658995930875,-8.90213758300391,
58.2366196633658));
#165966=CARTESIAN_POINT('Ctrl Pts',(69.3589219203545,-8.81979211963938,
58.270766107965));
#165967=CARTESIAN_POINT('Ctrl Pts',(69.3007710173797,-8.79597260492069,
58.2803457710644));
#165968=CARTESIAN_POINT('Ctrl Pts',(69.2070877663521,-8.75648712924794,
58.2957559864126));
#165969=CARTESIAN_POINT('Ctrl Pts',(69.1714091763204,-8.74118619755758,
58.3016194186712));
#165970=CARTESIAN_POINT('Ctrl Pts',(69.0970364615773,-8.70873966856432,
58.3138303997084));
#165971=CARTESIAN_POINT('Ctrl Pts',(69.0583608280893,-8.69155237292025,
58.3201738779777));
#165972=CARTESIAN_POINT('Ctrl Pts',(68.9664597646636,-8.64996066596164,
58.3352316354396));
#165973=CARTESIAN_POINT('Ctrl Pts',(68.9133412761308,-8.62531586063123,
58.3439223826436));
#165974=CARTESIAN_POINT('Ctrl Pts',(68.730647609949,-8.53845511514459,58.3737697325573));
#165975=CARTESIAN_POINT('Ctrl Pts',(68.6022456828645,-8.47373231820895,
58.3946711154594));
#165976=CARTESIAN_POINT('Ctrl Pts',(68.2876309439214,-8.30593524448026,
58.4457063579273));
#165977=CARTESIAN_POINT('Ctrl Pts',(68.1032959641086,-8.19939567851772,
58.4754482386249));
#165978=CARTESIAN_POINT('Ctrl Pts',(67.683390104038,-7.93722237801352,58.5429044841003));
#165979=CARTESIAN_POINT('Ctrl Pts',(67.4508270479315,-7.77701183523437,
58.580036018487));
#165980=CARTESIAN_POINT('Ctrl Pts',(66.9572753802927,-7.40312119395153,
58.6586383908438));
#165981=CARTESIAN_POINT('Ctrl Pts',(66.6997767536239,-7.18535010465191,
58.699512471634));
#165982=CARTESIAN_POINT('Ctrl Pts',(66.405273990402,-6.90781887102201,58.7465173880349));
#165983=CARTESIAN_POINT('Ctrl Pts',(66.3566607637489,-6.86101043103078,
58.7542857612975));
#165984=CARTESIAN_POINT('Ctrl Pts',(66.2868647553706,-6.79234423523244,
58.7654575914626));
#165985=CARTESIAN_POINT('Ctrl Pts',(66.2652823576705,-6.77090441929182,
58.768914770285));
#165986=CARTESIAN_POINT('Ctrl Pts',(66.2272199959874,-6.73272525092269,
58.775016997003));
#165987=CARTESIAN_POINT('Ctrl Pts',(66.2106985487345,-6.7160286307236,58.7776675293043));
#165988=CARTESIAN_POINT('Ctrl Pts',(66.1748659220609,-6.67954406521607,
58.7834201664776));
#165989=CARTESIAN_POINT('Ctrl Pts',(66.1555789469824,-6.65973244490992,
58.7865190376159));
#165990=CARTESIAN_POINT('Ctrl Pts',(66.1005243044022,-6.60267993284934,
58.7953712476851));
#165991=CARTESIAN_POINT('Ctrl Pts',(66.0649728854007,-6.56522726138834,
58.8010954656928));
#165992=CARTESIAN_POINT('Ctrl Pts',(65.7565366276555,-6.23490498020041,
58.8508132727081));
#165993=CARTESIAN_POINT('Ctrl Pts',(65.5020490795595,-5.92502819383749,
58.8922054022425));
#165994=CARTESIAN_POINT('Ctrl Pts',(64.9597925342817,-5.1723311809188,58.979809576188));
#165995=CARTESIAN_POINT('Ctrl Pts',(64.6875876356503,-4.71962774960106,
59.0232680778935));
#165996=CARTESIAN_POINT('Ctrl Pts',(64.4140003988791,-4.16582397143773,
59.0652657993448));
#165997=CARTESIAN_POINT('Ctrl Pts',(64.3753492468967,-4.08473939659121,
59.071152542755));
#165998=CARTESIAN_POINT('Ctrl Pts',(64.3153268503904,-3.95413642661544,
59.0802148035751));
#165999=CARTESIAN_POINT('Ctrl Pts',(64.2932291289846,-3.90496796953349,
59.0835327507685));
#166000=CARTESIAN_POINT('Ctrl Pts',(64.2546305702355,-3.81711575259759,
59.0892944688107));
#166001=CARTESIAN_POINT('Ctrl Pts',(64.2379685302801,-3.7785065003449,59.0917698858875));
#166002=CARTESIAN_POINT('Ctrl Pts',(64.2035733188108,-3.69734723674761,
59.0968546319753));
#166003=CARTESIAN_POINT('Ctrl Pts',(64.1858914669361,-3.6547760371065,59.0994539134053));
#166004=CARTESIAN_POINT('Ctrl Pts',(64.140050284931,-3.54212984967439,59.1061531492582));
#166005=CARTESIAN_POINT('Ctrl Pts',(64.1124065295386,-3.47184266590105,
59.1101520607643));
#166006=CARTESIAN_POINT('Ctrl Pts',(63.9798027934927,-3.12267875624334,
59.1291260463045));
#166007=CARTESIAN_POINT('Ctrl Pts',(63.8869542553808,-2.83925523774258,
59.1417289170361));
#166008=CARTESIAN_POINT('Ctrl Pts',(63.7129069177458,-2.21089146099731,
59.1637793026284));
#166009=CARTESIAN_POINT('Ctrl Pts',(63.6372555378738,-1.86483676705409,
59.1721779357039));
#166010=CARTESIAN_POINT('Ctrl Pts',(63.5180956564049,-1.12714682735523,
59.1828106063956));
#166011=CARTESIAN_POINT('Ctrl Pts',(63.4791919297343,-0.735415082438569,
59.1842481822503));
#166012=CARTESIAN_POINT('Ctrl Pts',(63.4618343046548,-0.273853639113625,
59.1816777182735));
#166013=CARTESIAN_POINT('Ctrl Pts',(63.4599906839625,-0.205259520316795,
59.1811859786441));
#166014=CARTESIAN_POINT('Ctrl Pts',(63.4584507715836,-0.109880378036844,
59.180354428042));
#166015=CARTESIAN_POINT('Ctrl Pts',(63.4581306047383,-0.0831067375661545,
59.1801048217527));
#166016=CARTESIAN_POINT('Ctrl Pts',(63.4577511232452,-0.0342698018506897,
59.1796203810379));
#166017=CARTESIAN_POINT('Ctrl Pts',(63.4576558191881,-0.0122068709101067,
59.1793906833755));
#166018=CARTESIAN_POINT('Ctrl Pts',(63.4576159489983,0.0337218633400005,
59.1788901583135));
#166019=CARTESIAN_POINT('Ctrl Pts',(63.457684329794,0.057587392495471,59.1786174763401));
#166020=CARTESIAN_POINT('Ctrl Pts',(63.4581008010244,0.120712245365185,
59.1778624818704));
#166021=CARTESIAN_POINT('Ctrl Pts',(63.4586008700874,0.159969842269242,
59.1773584203561));
#166022=CARTESIAN_POINT('Ctrl Pts',(63.4620960595867,0.345128205376628,
59.1748148461257));
#166023=CARTESIAN_POINT('Ctrl Pts',(63.468178171613,0.490944708985161,59.1723247478192));
#166024=CARTESIAN_POINT('Ctrl Pts',(63.4965488189744,0.93045841966588,59.163244855723));
#166025=CARTESIAN_POINT('Ctrl Pts',(63.5290179378633,1.22328611112202,59.1550636036953));
#166026=CARTESIAN_POINT('Ctrl Pts',(63.6686181643724,2.10929532762212,59.1230494862041));
#166027=CARTESIAN_POINT('Ctrl Pts',(63.8179937930836,2.69401063654907,59.0917808437044));
#166028=CARTESIAN_POINT('Ctrl Pts',(64.0554570573112,3.35730063841636,59.0428391276018));
#166029=CARTESIAN_POINT('Ctrl Pts',(64.0917292030743,3.45370334411235,59.0353808334483));
#166030=CARTESIAN_POINT('Ctrl Pts',(64.1487974626554,3.59827835157036,59.023668808162));
#166031=CARTESIAN_POINT('Ctrl Pts',(64.1684558640806,3.64690931156324,59.0196380582994));
#166032=CARTESIAN_POINT('Ctrl Pts',(64.2044678011045,3.73393536353802,59.0122604959219));
#166033=CARTESIAN_POINT('Ctrl Pts',(64.2206759275625,3.77239154330483,59.0089422111169));
#166034=CARTESIAN_POINT('Ctrl Pts',(64.2557944637189,3.8542191385288,59.0017569413866));
#166035=CARTESIAN_POINT('Ctrl Pts',(64.274775525406,3.89755777175095,58.9978760985742));
#166036=CARTESIAN_POINT('Ctrl Pts',(64.3273031571468,4.01511558334929,58.9871436296259));
#166037=CARTESIAN_POINT('Ctrl Pts',(64.3614721754089,4.0890409679415,58.9801699512999));
#166038=CARTESIAN_POINT('Ctrl Pts',(64.5992607382395,4.58673075596616,58.9316933437187));
#166039=CARTESIAN_POINT('Ctrl Pts',(64.8326852170686,4.99494823534751,58.8843238715129));
#166040=CARTESIAN_POINT('Ctrl Pts',(65.358300816401,5.77412544274659,58.7788790045957));
#166041=CARTESIAN_POINT('Ctrl Pts',(65.649988220925,6.14384609553888,58.7209169826352));
#166042=CARTESIAN_POINT('Ctrl Pts',(66.0097675065149,6.53558542780356,58.6510273826178));
#166043=CARTESIAN_POINT('Ctrl Pts',(66.05222831445,6.58090687953461,58.6428023858132));
#166044=CARTESIAN_POINT('Ctrl Pts',(66.1156504345957,6.64726820658499,58.6305549699009));
#166045=CARTESIAN_POINT('Ctrl Pts',(66.1362708934304,6.66864003795814,58.62657877699));
#166046=CARTESIAN_POINT('Ctrl Pts',(66.1732828920289,6.70663752490071,58.6194527015869));
#166047=CARTESIAN_POINT('Ctrl Pts',(66.1896360034283,6.7233009746769,58.616307941506));
#166048=CARTESIAN_POINT('Ctrl Pts',(66.2260668866879,6.76014664358343,58.6093105369019));
#166049=CARTESIAN_POINT('Ctrl Pts',(66.2461741871432,6.78029827867692,58.6054539918353));
#166050=CARTESIAN_POINT('Ctrl Pts',(66.3059925588714,6.83970444268061,58.593996417753));
#166051=CARTESIAN_POINT('Ctrl Pts',(66.3459598583983,6.87869254361963,58.5863611320225));
#166052=CARTESIAN_POINT('Ctrl Pts',(66.4394146701516,6.96824093468274,58.5685489086856));
#166053=CARTESIAN_POINT('Ctrl Pts',(66.4931511128061,7.01852921551875,58.5583375366121));
#166054=CARTESIAN_POINT('Ctrl Pts',(66.6829009485287,7.19195270944137,58.5223697847538));
#166055=CARTESIAN_POINT('Ctrl Pts',(66.8218921440944,7.31167686861458,58.4961810736965));
#166056=CARTESIAN_POINT('Ctrl Pts',(67.4356645422906,7.80970632140385,58.380913421749));
#166057=CARTESIAN_POINT('Ctrl Pts',(67.9425461031012,8.14487508335537,58.2865552367253));
#166058=CARTESIAN_POINT('Ctrl Pts',(68.5921948127466,8.48867485512041,58.1646835488871));
#166059=CARTESIAN_POINT('Ctrl Pts',(68.7080953465377,8.54693471289744,58.142912691477));
#166060=CARTESIAN_POINT('Ctrl Pts',(68.8719258426988,8.62502866111454,58.1120904502235));
#166061=CARTESIAN_POINT('Ctrl Pts',(68.9188907261812,8.64693427662143,58.1032493063875));
#166062=CARTESIAN_POINT('Ctrl Pts',(69.0010780212418,8.68443250504215,58.0877676998032));
#166063=CARTESIAN_POINT('Ctrl Pts',(69.0362212648362,8.70020266442263,58.0811446666722));
#166064=CARTESIAN_POINT('Ctrl Pts',(69.1101901815239,8.73284265346263,58.0671979567376));
#166065=CARTESIAN_POINT('Ctrl Pts',(69.1490345705707,8.74966607146115,58.0598700918789));
#166066=CARTESIAN_POINT('Ctrl Pts',(69.2424866468514,8.78938097557269,58.0422313740177));
#166067=CARTESIAN_POINT('Ctrl Pts',(69.2971975807493,8.81201435652634,58.0318973295296));
#166068=CARTESIAN_POINT('Ctrl Pts',(69.4897458104812,8.88951323494433,57.9955013836361));
#166069=CARTESIAN_POINT('Ctrl Pts',(69.6286431754133,8.94156962665868,57.9691988128118));
#166070=CARTESIAN_POINT('Ctrl Pts',(69.9748682489228,9.06190106629557,57.9035264465876));
#166071=CARTESIAN_POINT('Ctrl Pts',(70.1834304044669,9.12618978726953,57.863870368685));
#166072=CARTESIAN_POINT('Ctrl Pts',(70.7028002024069,9.26629221478336,57.7649666553917));
#166073=CARTESIAN_POINT('Ctrl Pts',(71.0155745061857,9.33339916284094,57.705270111172));
#166074=CARTESIAN_POINT('Ctrl Pts',(71.7005761738355,9.44334972702121,57.5746884034147));
#166075=CARTESIAN_POINT('Ctrl Pts',(72.0732182454311,9.47999121557342,57.5037495315944));
#166076=CARTESIAN_POINT('Ctrl Pts',(72.513290420408,9.49621256482875,57.4206877415447));
#166077=CARTESIAN_POINT('Ctrl Pts',(72.5794908998034,9.49793529243034,57.4082120144596));
#166078=CARTESIAN_POINT('Ctrl Pts',(72.6726276418172,9.49935020822693,57.3906918969534));
#166079=CARTESIAN_POINT('Ctrl Pts',(72.6995497270857,9.49964069820312,57.3856312785984));
#166080=CARTESIAN_POINT('Ctrl Pts',(72.7483092080848,9.49995221351492,57.3764730155845));
#166081=CARTESIAN_POINT('Ctrl Pts',(72.7701459677609,9.50001378619696,57.3723741342232));
#166082=CARTESIAN_POINT('Ctrl Pts',(72.8151615606201,9.4999800559609,57.3639300826564));
#166083=CARTESIAN_POINT('Ctrl Pts',(72.8383402134398,9.49987488822714,57.3595852674416));
#166084=CARTESIAN_POINT('Ctrl Pts',(72.8988418013406,9.49937119930833,57.3482518546046));
#166085=CARTESIAN_POINT('Ctrl Pts',(72.9361640276583,9.49883283030553,57.3412679960177));
#166086=CARTESIAN_POINT('Ctrl Pts',(73.10319284995,9.49540451543168,57.3100436522301));
#166087=CARTESIAN_POINT('Ctrl Pts',(73.2328486573126,9.48999284421492,57.2858883954586));
#166088=CARTESIAN_POINT('Ctrl Pts',(73.6072928003073,9.46640790572726,57.216291097849));
#166089=CARTESIAN_POINT('Ctrl Pts',(73.8515669108966,9.441168921131,57.1710879382823));
#166090=CARTESIAN_POINT('Ctrl Pts',(74.7034632924967,9.31850590757357,57.0135927396289));
#166091=CARTESIAN_POINT('Ctrl Pts',(75.3023796762721,9.16990982265294,56.9030231328975));
#166092=CARTESIAN_POINT('Ctrl Pts',(76.0007690120131,8.92021274348208,56.7724941712806));
#166093=CARTESIAN_POINT('Ctrl Pts',(76.1183267105528,8.87545021938119,56.7504709276739));
#166094=CARTESIAN_POINT('Ctrl Pts',(76.2826085955656,8.80901992753693,56.7196150568381));
#166095=CARTESIAN_POINT('Ctrl Pts',(76.330106822762,8.78934997369507,56.7106843669005));
#166096=CARTESIAN_POINT('Ctrl Pts',(76.4128125868205,8.75428783924872,56.69511709506));
#166097=CARTESIAN_POINT('Ctrl Pts',(76.4480914823061,8.73907136046434,56.6884713459493));
#166098=CARTESIAN_POINT('Ctrl Pts',(76.522118476229,8.70659275695773,56.6745149012532));
#166099=CARTESIAN_POINT('Ctrl Pts',(76.5608451456952,8.68928278384494,56.6672070542079));
#166100=CARTESIAN_POINT('Ctrl Pts',(76.6537825333726,8.6469715533625,56.6496534405775));
#166101=CARTESIAN_POINT('Ctrl Pts',(76.7078753199147,8.62170940100036,56.6394233953001));
#166102=CARTESIAN_POINT('Ctrl Pts',(76.8990236621945,8.53017444644027,56.6032266241227));
#166103=CARTESIAN_POINT('Ctrl Pts',(77.0347113767622,8.46102951430872,56.5774457164988));
#166104=CARTESIAN_POINT('Ctrl Pts',(77.372188359274,8.2784308202126,56.513120628478));
#166105=CARTESIAN_POINT('Ctrl Pts',(77.5715967846075,8.16067677074287,56.4749214948603));
#166106=CARTESIAN_POINT('Ctrl Pts',(78.1435115207567,7.79343686371792,56.3649417854438));
#166107=CARTESIAN_POINT('Ctrl Pts',(78.5029051506694,7.52414998124982,56.2952553351274));
#166108=CARTESIAN_POINT('Ctrl Pts',(78.9731276143691,7.11592841205867,56.2042026624885));
#166109=CARTESIAN_POINT('Ctrl Pts',(79.1011037590377,6.99844373604352,56.1794400529462));
#166110=CARTESIAN_POINT('Ctrl Pts',(79.2579034729459,6.84628899232401,56.1491920621841));
#166111=CARTESIAN_POINT('Ctrl Pts',(79.289764636081,6.81492843323477,56.1430507643067));
#166112=CARTESIAN_POINT('Ctrl Pts',(79.3398887488457,6.76488519594189,56.1333987718262));
#166113=CARTESIAN_POINT('Ctrl Pts',(79.3582961158376,6.74635426586193,56.1298562806674));
#166114=CARTESIAN_POINT('Ctrl Pts',(79.3933220572914,6.71079923891036,56.1231198966335));
#166115=CARTESIAN_POINT('Ctrl Pts',(79.4099533049714,6.69378865455075,56.1199232173048));
#166116=CARTESIAN_POINT('Ctrl Pts',(79.4498969180057,6.65262389789042,56.1122500527163));
#166117=CARTESIAN_POINT('Ctrl Pts',(79.4731464459963,6.62840658658628,56.1077874188129));
#166118=CARTESIAN_POINT('Ctrl Pts',(79.5545828876644,6.54266990921175,56.0921672264141));
#166119=CARTESIAN_POINT('Ctrl Pts',(79.6120847655959,6.48047858045167,56.0811580853381));
#166120=CARTESIAN_POINT('Ctrl Pts',(79.9932580253986,6.0569350518507,56.0082697235066));
#166121=CARTESIAN_POINT('Ctrl Pts',(80.2899998620266,5.67139016463378,55.9519340984355));
#166122=CARTESIAN_POINT('Ctrl Pts',(80.7872610621668,4.91081443741658,55.8563313444425));
#166123=CARTESIAN_POINT('Ctrl Pts',(80.9947410748632,4.54194499828788,55.8159041640985));
#166124=CARTESIAN_POINT('Ctrl Pts',(81.2120322527243,4.08712522786176,55.7724037211774));
#166125=CARTESIAN_POINT('Ctrl Pts',(81.2460056044337,4.01361957094386,55.7655628714518));
#166126=CARTESIAN_POINT('Ctrl Pts',(81.2983012757139,3.89657625643701,55.7549664623227));
#166127=CARTESIAN_POINT('Ctrl Pts',(81.3172408583193,3.85332761465832,55.7511142273554));
#166128=CARTESIAN_POINT('Ctrl Pts',(81.3506754159879,3.77540953365872,55.7442868377559));
#166129=CARTESIAN_POINT('Ctrl Pts',(81.3652876431223,3.74079311765809,55.74129333845));
#166130=CARTESIAN_POINT('Ctrl Pts',(81.3990929565398,3.65936857304152,55.7343447963729));
#166131=CARTESIAN_POINT('Ctrl Pts',(81.4181197947196,3.61249046291403,55.7304158120876));
#166132=CARTESIAN_POINT('Ctrl Pts',(81.4725625338198,3.47523262042645,55.7191195440899));
#166133=CARTESIAN_POINT('Ctrl Pts',(81.506977945323,3.38445030414383,55.7119091971599));
#166134=CARTESIAN_POINT('Ctrl Pts',(81.6552567033774,2.97456775411852,55.6805205439986));
#166135=CARTESIAN_POINT('Ctrl Pts',(81.753539505228,2.64991192052269,55.6587916894816));
#166136=CARTESIAN_POINT('Ctrl Pts',(81.9463990317789,1.8649415804742,55.6138400937547));
#166137=CARTESIAN_POINT('Ctrl Pts',(82.0248331947055,1.40143044588836,55.5932858276554));
#166138=CARTESIAN_POINT('Ctrl Pts',(82.0911569428425,0.703069833957399,
55.5721697258594));
#166139=CARTESIAN_POINT('Ctrl Pts',(82.1047641805439,0.471530348682286,
55.5667690652911));
#166140=CARTESIAN_POINT('Ctrl Pts',(82.1111072228302,0.193590158400646,
55.5623443144614));
#166141=CARTESIAN_POINT('Ctrl Pts',(82.1118304466039,0.147474929573563,
55.5616780488397));
#166142=CARTESIAN_POINT('Ctrl Pts',(82.1124440055481,0.0757145567867833,
55.5607484876857));
#166143=CARTESIAN_POINT('Ctrl Pts',(82.1125615741381,0.0500726765295319,
55.5604376291905));
#166144=CARTESIAN_POINT('Ctrl Pts',(82.1125825678391,0.0162869168660211,
55.5600563429909));
#166145=CARTESIAN_POINT('Ctrl Pts',(82.1125773773997,0.00814345295206416,
55.5599666070003));
#166146=CARTESIAN_POINT('Ctrl Pts',(82.1125619375607,6.64456069956318E-11,
55.5598790433222));
#166147=CARTESIAN_POINT('Origin',(73.0915550886457,-4.33680868994202E-16,
59.1075264962884));
#166148=CARTESIAN_POINT('',(81.9917963385783,-3.33461157104299E-11,54.8749832973778));
#166149=CARTESIAN_POINT('',(81.9996906220771,-1.55047049271929E-14,54.9197540038636));
#166150=CARTESIAN_POINT('',(82.4472287422617,-1.59709532818419E-15,57.4578688084528));
#166151=CARTESIAN_POINT('',(63.3368846312614,3.0524913646464E-5,58.4943608645448));
#166152=CARTESIAN_POINT('Ctrl Pts',(81.9917963385783,-6.66906343255317E-11,
54.8749832973778));
#166153=CARTESIAN_POINT('Ctrl Pts',(81.991822202953,0.0136416781824146,
54.8751299815349));
#166154=CARTESIAN_POINT('Ctrl Pts',(81.991818955162,0.0272833257654345,
54.8752807745152));
#166155=CARTESIAN_POINT('Ctrl Pts',(81.9917192856842,0.0693062239870782,
54.8757580399907));
#166156=CARTESIAN_POINT('Ctrl Pts',(81.99152598214,0.0976868811112656,54.8760982822577));
#166157=CARTESIAN_POINT('Ctrl Pts',(81.9905186336026,0.187235803710298,
54.8772292123879));
#166158=CARTESIAN_POINT('Ctrl Pts',(81.9892454504036,0.248396492949711,
54.8780861012472));
#166159=CARTESIAN_POINT('Ctrl Pts',(81.9795354315075,0.567997185026232,
54.8830191445056));
#166160=CARTESIAN_POINT('Ctrl Pts',(81.9612443602764,0.826005727639437,
54.8885606355397));
#166161=CARTESIAN_POINT('Ctrl Pts',(81.8645511642046,1.69300376845709,54.913062124542));
#166162=CARTESIAN_POINT('Ctrl Pts',(81.7383288190462,2.29486230360472,54.9400344663477));
#166163=CARTESIAN_POINT('Ctrl Pts',(81.497067905793,3.06905576684948,54.9901588241199));
#166164=CARTESIAN_POINT('Ctrl Pts',(81.432376243716,3.25611442761254,55.0035099977753));
#166165=CARTESIAN_POINT('Ctrl Pts',(81.3376476752165,3.50488393824609,55.022979412955));
#166166=CARTESIAN_POINT('Ctrl Pts',(81.3126309701757,3.56852830174184,55.0281143059707));
#166167=CARTESIAN_POINT('Ctrl Pts',(81.2702098679784,3.67315345139376,55.0368113929279));
#166168=CARTESIAN_POINT('Ctrl Pts',(81.253194191831,3.71429536934038,55.040297353785));
#166169=CARTESIAN_POINT('Ctrl Pts',(81.2193427253909,3.7945577454254,55.0472275977369));
#166170=CARTESIAN_POINT('Ctrl Pts',(81.2025313565162,3.83368776873125,55.0506670860519));
#166171=CARTESIAN_POINT('Ctrl Pts',(81.1619670388033,3.92639703176895,55.0589610766492));
#166172=CARTESIAN_POINT('Ctrl Pts',(81.1379837930375,3.97986952069685,55.0638607501625));
#166173=CARTESIAN_POINT('Ctrl Pts',(81.0541097233846,4.16237037103102,55.0809818458129));
#166174=CARTESIAN_POINT('Ctrl Pts',(80.9918526715719,4.29024609594483,55.0936669948476));
#166175=CARTESIAN_POINT('Ctrl Pts',(80.8312419286745,4.60226080407488,55.1263253193423));
#166176=CARTESIAN_POINT('Ctrl Pts',(80.7296877504282,4.78460136845639,55.1469202453345));
#166177=CARTESIAN_POINT('Ctrl Pts',(80.4732935602959,5.21136273873443,55.1987132090407));
#166178=CARTESIAN_POINT('Ctrl Pts',(80.3131845921018,5.45225107835511,55.2309038922635));
#166179=CARTESIAN_POINT('Ctrl Pts',(79.9417403939865,5.9591706910903,55.3049417488796));
#166180=CARTESIAN_POINT('Ctrl Pts',(79.7266145186263,6.22183123157583,55.3474398971995));
#166181=CARTESIAN_POINT('Ctrl Pts',(79.4524712165179,6.52186675344831,55.4007332273436));
#166182=CARTESIAN_POINT('Ctrl Pts',(79.4064728570105,6.57113337114255,55.4096481509804));
#166183=CARTESIAN_POINT('Ctrl Pts',(79.338997706285,6.64185875161774,55.422681744697));
#166184=CARTESIAN_POINT('Ctrl Pts',(79.3179361910792,6.66372117936767,55.4267439634255));
#166185=CARTESIAN_POINT('Ctrl Pts',(79.2804335601575,6.70227325156488,55.4339660214015));
#166186=CARTESIAN_POINT('Ctrl Pts',(79.2640349059499,6.71900476701175,55.437120206646));
#166187=CARTESIAN_POINT('Ctrl Pts',(79.2282059474958,6.75528768562118,55.4440033795961));
#166188=CARTESIAN_POINT('Ctrl Pts',(79.2087522011366,6.77481474193493,55.4477354688866));
#166189=CARTESIAN_POINT('Ctrl Pts',(79.1527428968766,6.83054099504196,55.4584663933232));
#166190=CARTESIAN_POINT('Ctrl Pts',(79.1159775864347,6.86652253921298,55.4654932185649));
#166191=CARTESIAN_POINT('Ctrl Pts',(78.7933984052931,7.17706351102956,55.5270130497113));
#166192=CARTESIAN_POINT('Ctrl Pts',(78.4909486579221,7.43330334489731,55.5838052057719));
#166193=CARTESIAN_POINT('Ctrl Pts',(77.7511566541425,7.98344925921708,55.7222660152397));
#166194=CARTESIAN_POINT('Ctrl Pts',(77.3035766757266,8.26086009597974,55.805746966175));
#166195=CARTESIAN_POINT('Ctrl Pts',(76.7566752516894,8.53880776098687,55.9084539870362));
#166196=CARTESIAN_POINT('Ctrl Pts',(76.6771731922565,8.57779082629611,55.9233987068999));
#166197=CARTESIAN_POINT('Ctrl Pts',(76.5490636132609,8.63834843265285,55.9475063369901));
#166198=CARTESIAN_POINT('Ctrl Pts',(76.500796050963,8.66065846918242,55.9565950611723));
#166199=CARTESIAN_POINT('Ctrl Pts',(76.4145195977121,8.69963913090307,55.9728514654561));
#166200=CARTESIAN_POINT('Ctrl Pts',(76.3765831446,8.71647313843432,55.9800031678328));
#166201=CARTESIAN_POINT('Ctrl Pts',(76.2968025684778,8.75123513076655,55.9950510013327));
#166202=CARTESIAN_POINT('Ctrl Pts',(76.2549375318103,8.76911030212713,56.0029518289265));
#166203=CARTESIAN_POINT('Ctrl Pts',(76.1440758541751,8.81548107436813,56.0238856485684));
#166204=CARTESIAN_POINT('Ctrl Pts',(76.0748708856314,8.84344856526899,56.0369655618164));
#166205=CARTESIAN_POINT('Ctrl Pts',(75.7297081960262,8.97809933104723,56.1022615536476));
#166206=CARTESIAN_POINT('Ctrl Pts',(75.4492500127483,9.07226093207452,56.1555113554325));
#166207=CARTESIAN_POINT('Ctrl Pts',(74.8310771239294,9.24722341257852,56.2731665960856));
#166208=CARTESIAN_POINT('Ctrl Pts',(74.4923719244879,9.32271168206536,56.3378123708414));
#166209=CARTESIAN_POINT('Ctrl Pts',(74.0129518046217,9.40140154366368,56.4292120766649));
#166210=CARTESIAN_POINT('Ctrl Pts',(73.8751021455843,9.4208187929465,56.45547904903));
#166211=CARTESIAN_POINT('Ctrl Pts',(73.7175404796332,9.43936722476629,56.4854602625635));
#166212=CARTESIAN_POINT('Ctrl Pts',(73.6982026510341,9.44158133535963,56.4891391895567));
#166213=CARTESIAN_POINT('Ctrl Pts',(73.4220823440751,9.47230612172538,56.5416584423132));
#166214=CARTESIAN_POINT('Ctrl Pts',(73.1642259668995,9.49001679707639,56.5905675372639));
#166215=CARTESIAN_POINT('Ctrl Pts',(72.8594630057541,9.49804316407024,56.6480002327844));
#166216=CARTESIAN_POINT('Ctrl Pts',(72.8129906181892,9.49891377063772,56.6567476616759));
#166217=CARTESIAN_POINT('Ctrl Pts',(72.7410540043522,9.49971469902503,56.6702704363055));
#166218=CARTESIAN_POINT('Ctrl Pts',(72.7155946351273,9.49989219977281,56.675052894336));
#166219=CARTESIAN_POINT('Ctrl Pts',(72.6687248088224,9.50002392434837,56.6838505462437));
#166220=CARTESIAN_POINT('Ctrl Pts',(72.6473149955808,9.50000918001051,56.6878666488272));
#166221=CARTESIAN_POINT('Ctrl Pts',(72.5983459483423,9.49980411519282,56.6970465111595));
#166222=CARTESIAN_POINT('Ctrl Pts',(72.5707869368163,9.49956458812455,56.7022085834119));
#166223=CARTESIAN_POINT('Ctrl Pts',(72.4848976354765,9.49843124767219,56.7182841912745));
#166224=CARTESIAN_POINT('Ctrl Pts',(72.4265717902344,9.49710551926816,56.7291831664741));
#166225=CARTESIAN_POINT('Ctrl Pts',(72.1296332775477,9.48752409589665,56.7845926839847));
#166226=CARTESIAN_POINT('Ctrl Pts',(71.8913397750163,9.47051927253352,56.8288058687247));
#166227=CARTESIAN_POINT('Ctrl Pts',(71.1171880893997,9.38484804840058,56.9721234769666));
#166228=CARTESIAN_POINT('Ctrl Pts',(70.5864432169096,9.27824049392138,57.0699384308583));
#166229=CARTESIAN_POINT('Ctrl Pts',(69.8156442116516,9.0513864358103,57.213171090579));
#166230=CARTESIAN_POINT('Ctrl Pts',(69.5666531002123,8.96637507420435,57.2596181024116));
#166231=CARTESIAN_POINT('Ctrl Pts',(69.2519054533381,8.84364950773871,57.3186429608563));
#166232=CARTESIAN_POINT('Ctrl Pts',(69.1825805723832,8.8156434547148,57.3316630610408));
#166233=CARTESIAN_POINT('Ctrl Pts',(69.0715775351641,8.76922371636642,57.3525433929398));
#166234=CARTESIAN_POINT('Ctrl Pts',(69.029686498261,8.7513402610294,57.360430878969));
#166235=CARTESIAN_POINT('Ctrl Pts',(68.9498867236237,8.71657325746769,57.3754705973699));
#166236=CARTESIAN_POINT('Ctrl Pts',(68.9119565312135,8.69974292344304,57.3826255719642));
#166237=CARTESIAN_POINT('Ctrl Pts',(68.8249146434011,8.66041682892671,57.399059404075));
#166238=CARTESIAN_POINT('Ctrl Pts',(68.775882588084,8.63774409131317,57.4083276623536));
#166239=CARTESIAN_POINT('Ctrl Pts',(68.6211333199697,8.56453366338655,57.4376132721707));
#166240=CARTESIAN_POINT('Ctrl Pts',(68.5161612741623,8.51240814632917,57.457529901406));
#166241=CARTESIAN_POINT('Ctrl Pts',(68.0223239866527,8.25537752182242,57.5514608053063));
#166242=CARTESIAN_POINT('Ctrl Pts',(67.647104262967,8.02479308931199,57.6235614884343));
#166243=CARTESIAN_POINT('Ctrl Pts',(66.9399448512522,7.51785093283388,57.7601611502722));
#166244=CARTESIAN_POINT('Ctrl Pts',(66.6080119512906,7.24331659887673,57.8246334087274));
#166245=CARTESIAN_POINT('Ctrl Pts',(66.2486458041058,6.90192052883975,57.8940346930678));
#166246=CARTESIAN_POINT('Ctrl Pts',(66.2020840203413,6.85676277896533,57.9030178785215));
#166247=CARTESIAN_POINT('Ctrl Pts',(66.1345113211875,6.78986044647605,57.9160371865043));
#166248=CARTESIAN_POINT('Ctrl Pts',(66.1131405661603,6.76849735758833,57.9201520934272));
#166249=CARTESIAN_POINT('Ctrl Pts',(66.0754199704642,6.73042629166389,57.9274099213748));
#166250=CARTESIAN_POINT('Ctrl Pts',(66.0590298253972,6.71376050645764,57.9305617550486));
#166251=CARTESIAN_POINT('Ctrl Pts',(66.0231142448563,6.67696861203359,57.9374642952437));
#166252=CARTESIAN_POINT('Ctrl Pts',(66.0036158180696,6.65681565072191,57.9412090632313));
#166253=CARTESIAN_POINT('Ctrl Pts',(65.9470124781257,6.59778835740629,57.9520731916278));
#166254=CARTESIAN_POINT('Ctrl Pts',(65.910144454658,6.55867893066332,57.9591408116212));
#166255=CARTESIAN_POINT('Ctrl Pts',(65.6269926458696,6.2531302195564,58.013368062779));
#166256=CARTESIAN_POINT('Ctrl Pts',(65.3956304170986,5.97272513253239,58.0573724679904));
#166257=CARTESIAN_POINT('Ctrl Pts',(64.8474171024937,5.22442921639762,58.1620855123274));
#166258=CARTESIAN_POINT('Ctrl Pts',(64.5548844302348,4.73991907109159,58.2184731058303));
#166259=CARTESIAN_POINT('Ctrl Pts',(64.2688475762087,4.15382796894945,58.2755288795974));
#166260=CARTESIAN_POINT('Ctrl Pts',(64.2318891786658,4.07540125109142,58.2829450348384));
#166261=CARTESIAN_POINT('Ctrl Pts',(64.1738420288055,3.9477326263978,58.2946687941808));
#166262=CARTESIAN_POINT('Ctrl Pts',(64.1520923378673,3.89880641086579,58.2990799771926));
#166263=CARTESIAN_POINT('Ctrl Pts',(64.1140813270938,3.81132173476508,58.3068230679135));
#166264=CARTESIAN_POINT('Ctrl Pts',(64.0976602374692,3.77283648832602,58.310179974861));
#166265=CARTESIAN_POINT('Ctrl Pts',(64.0634664255108,3.69121423632517,58.3171956561457));
#166266=CARTESIAN_POINT('Ctrl Pts',(64.045755523884,3.64805171104448,58.3208447283219));
#166267=CARTESIAN_POINT('Ctrl Pts',(63.9991674693799,3.53209939745555,58.3304852567978));
#166268=CARTESIAN_POINT('Ctrl Pts',(63.9708658961972,3.4590748500883,58.3363864556028));
#166269=CARTESIAN_POINT('Ctrl Pts',(63.8232071111125,3.06371322672641,58.3674231579553));
#166270=CARTESIAN_POINT('Ctrl Pts',(63.7203555870873,2.73528691767668,58.389970233282));
#166271=CARTESIAN_POINT('Ctrl Pts',(63.5567199579687,2.09351567700281,58.4277325472171));
#166272=CARTESIAN_POINT('Ctrl Pts',(63.4934588896194,1.7812977680813,58.4433452294117));
#166273=CARTESIAN_POINT('Ctrl Pts',(63.3872349261475,1.0799454195237,58.4719251273082));
#166274=CARTESIAN_POINT('Ctrl Pts',(63.3522544858942,0.690120749571852,
58.4834602951632));
#166275=CARTESIAN_POINT('Ctrl Pts',(63.3392591469475,0.241427481035377,
58.4911696626021));
#166276=CARTESIAN_POINT('Ctrl Pts',(63.3381031341895,0.183678751037265,
58.4920560999298));
#166277=CARTESIAN_POINT('Ctrl Pts',(63.3372051441276,0.102655098814244,
58.4931485860234));
#166278=CARTESIAN_POINT('Ctrl Pts',(63.3370309983082,0.0793874405663537,
58.493444825801));
#166279=CARTESIAN_POINT('Ctrl Pts',(63.3368678653725,0.0374198454953173,
58.493947359837));
#166280=CARTESIAN_POINT('Ctrl Pts',(63.3368492358014,0.0187302153537607,
58.494159780901));
#166281=CARTESIAN_POINT('Ctrl Pts',(63.3368846312614,3.05249101211109E-5,
58.4943608645448));
#166282=CARTESIAN_POINT('Ctrl Pts',(63.3368846312614,3.05249136617253E-5,
58.4943608645448));
#166283=CARTESIAN_POINT('Ctrl Pts',(63.3369208637748,-0.0191113871700155,
58.4945667035367));
#166284=CARTESIAN_POINT('Ctrl Pts',(63.3370136687594,-0.0382432773275274,
58.4947604411253));
#166285=CARTESIAN_POINT('Ctrl Pts',(63.3373508002251,-0.081412204403057,
58.4951707098884));
#166286=CARTESIAN_POINT('Ctrl Pts',(63.3376276930398,-0.105438922169356,
58.4953802730565));
#166287=CARTESIAN_POINT('Ctrl Pts',(63.3389067619386,-0.189363842556669,
58.4960472253987));
#166288=CARTESIAN_POINT('Ctrl Pts',(63.3403745355787,-0.249254289988703,
58.4964074262296));
#166289=CARTESIAN_POINT('Ctrl Pts',(63.3600723622294,-0.83227138533733,
58.4988104441391));
#166290=CARTESIAN_POINT('Ctrl Pts',(63.4201008376448,-1.35312302820521,
58.4923494029091));
#166291=CARTESIAN_POINT('Ctrl Pts',(63.5897881989267,-2.20684882306762,
58.469621999276));
#166292=CARTESIAN_POINT('Ctrl Pts',(63.6758097808222,-2.54333582905673,
58.4573954212617));
#166293=CARTESIAN_POINT('Ctrl Pts',(63.8408072476067,-3.06832455602437,
58.4334381770832));
#166294=CARTESIAN_POINT('Ctrl Pts',(63.9079247690089,-3.26030711162486,
58.4235995160826));
#166295=CARTESIAN_POINT('Ctrl Pts',(64.0051843994766,-3.51243991047723,
58.4092595788151));
#166296=CARTESIAN_POINT('Ctrl Pts',(64.0299377876326,-3.57465765612895,
58.4056035909721));
#166297=CARTESIAN_POINT('Ctrl Pts',(64.0721357637391,-3.67756484516007,
58.3993614027841));
#166298=CARTESIAN_POINT('Ctrl Pts',(64.0892146914298,-3.71840504596493,
58.3968324897989));
#166299=CARTESIAN_POINT('Ctrl Pts',(64.1231901244958,-3.79809073582831,
58.3917969713027));
#166300=CARTESIAN_POINT('Ctrl Pts',(64.1400625365877,-3.83694561066209,
58.3892941352866));
#166301=CARTESIAN_POINT('Ctrl Pts',(64.1812311848857,-3.93005322047514,
58.383182101967));
#166302=CARTESIAN_POINT('Ctrl Pts',(64.2057753422229,-3.9841917966498,58.3795340690249));
#166303=CARTESIAN_POINT('Ctrl Pts',(64.2883248672261,-4.16185120570181,
58.3672509236198));
#166304=CARTESIAN_POINT('Ctrl Pts',(64.3484618297949,-4.28433922271799,
58.3582815095215));
#166305=CARTESIAN_POINT('Ctrl Pts',(64.6905627408281,-4.94497349033314,
58.3071238990448));
#166306=CARTESIAN_POINT('Ctrl Pts',(65.0205461204864,-5.45606972650783,
58.2574253140063));
#166307=CARTESIAN_POINT('Ctrl Pts',(65.5092364819749,-6.07456577013193,
58.1817935662063));
#166308=CARTESIAN_POINT('Ctrl Pts',(65.6261553977769,-6.21410952578817,
58.1635654708648));
#166309=CARTESIAN_POINT('Ctrl Pts',(65.7956166646602,-6.4049591856445,58.1368857455231));
#166310=CARTESIAN_POINT('Ctrl Pts',(65.8449059334505,-6.45919241571806,
58.1290964935448));
#166311=CARTESIAN_POINT('Ctrl Pts',(65.9327277908391,-6.55360555782429,
58.115159915273));
#166312=CARTESIAN_POINT('Ctrl Pts',(65.9709997234127,-6.59403121683617,
58.1090676965539));
#166313=CARTESIAN_POINT('Ctrl Pts',(66.0293810769665,-6.65462197163174,
58.0997434517078));
#166314=CARTESIAN_POINT('Ctrl Pts',(66.0492338026511,-6.67504131205081,
58.0965674034375));
#166315=CARTESIAN_POINT('Ctrl Pts',(66.0855740390587,-6.71208378603744,
58.0907435687896));
#166316=CARTESIAN_POINT('Ctrl Pts',(66.1020321035148,-6.72873618763518,
58.0881022489186));
#166317=CARTESIAN_POINT('Ctrl Pts',(66.1396151271271,-6.76648257787124,
58.0820621457074));
#166318=CARTESIAN_POINT('Ctrl Pts',(66.160777570398,-6.78753731511597,58.0786550651021));
#166319=CARTESIAN_POINT('Ctrl Pts',(66.2266729591109,-6.852481059745,58.0680286443838));
#166320=CARTESIAN_POINT('Ctrl Pts',(66.2717359575052,-6.89602084411713,
58.0607369423431));
#166321=CARTESIAN_POINT('Ctrl Pts',(66.6586584089125,-7.26250928516937,
57.9979444446001));
#166322=CARTESIAN_POINT('Ctrl Pts',(67.0232922894948,-7.55960861704001,
57.937592563155));
#166323=CARTESIAN_POINT('Ctrl Pts',(67.7915681430084,-8.09507772881114,
57.8102654879827));
#166324=CARTESIAN_POINT('Ctrl Pts',(68.1939658545534,-8.33294420832425,
57.743505870903));
#166325=CARTESIAN_POINT('Ctrl Pts',(68.6846877278869,-8.57534972289602,
57.6626472369883));
#166326=CARTESIAN_POINT('Ctrl Pts',(68.7576310234073,-8.61020786993134,
57.6506403913566));
#166327=CARTESIAN_POINT('Ctrl Pts',(68.8736324174974,-8.66379787626326,
57.6315672530401));
#166328=CARTESIAN_POINT('Ctrl Pts',(68.9163993634356,-8.68316389436018,
57.624539950053));
#166329=CARTESIAN_POINT('Ctrl Pts',(68.9971501917322,-8.71899606356189,
57.611280019271));
#166330=CARTESIAN_POINT('Ctrl Pts',(69.0351015825265,-8.73553418863046,
57.6050516972604));
#166331=CARTESIAN_POINT('Ctrl Pts',(69.1209883407484,-8.77228086811203,
57.5909648021187));
#166332=CARTESIAN_POINT('Ctrl Pts',(69.1689843142457,-8.79234121316166,
57.5830984031688));
#166333=CARTESIAN_POINT('Ctrl Pts',(69.311680099136,-8.85058041724986,57.559728156058));
#166334=CARTESIAN_POINT('Ctrl Pts',(69.4068350908284,-8.88759967514904,
57.5441663208849));
#166335=CARTESIAN_POINT('Ctrl Pts',(70.0614171591809,-9.12991788946181,
57.4372626359304));
#166336=CARTESIAN_POINT('Ctrl Pts',(70.6385650868135,-9.28243004052871,
57.3438531483033));
#166337=CARTESIAN_POINT('Ctrl Pts',(71.513186721696,-9.42548798437507,57.2020976284825));
#166338=CARTESIAN_POINT('Ctrl Pts',(71.8023342095742,-9.45889916442988,
57.1551797555897));
#166339=CARTESIAN_POINT('Ctrl Pts',(72.2362399202519,-9.48842566885487,
57.0843579497743));
#166340=CARTESIAN_POINT('Ctrl Pts',(72.3801735704896,-9.4948495061206,57.0607963021624));
#166341=CARTESIAN_POINT('Ctrl Pts',(72.5629167595653,-9.49873403448535,
57.0307531726488));
#166342=CARTESIAN_POINT('Ctrl Pts',(72.6016575913313,-9.49931410024482,
57.0243768121353));
#166343=CARTESIAN_POINT('Ctrl Pts',(72.6639486647109,-9.49985540442961,
57.0141114504137));
#166344=CARTESIAN_POINT('Ctrl Pts',(72.6874979688409,-9.49997011154059,
57.0102276474667));
#166345=CARTESIAN_POINT('Ctrl Pts',(72.7328165285815,-9.50001778243422,
57.0027476311316));
#166346=CARTESIAN_POINT('Ctrl Pts',(72.754585577935,-9.49996382400027,56.9991518766479));
#166347=CARTESIAN_POINT('Ctrl Pts',(72.8027704012823,-9.49967426068319,
56.9911871488104));
#166348=CARTESIAN_POINT('Ctrl Pts',(72.829185631001,-9.49940232792237,56.9868170583928));
#166349=CARTESIAN_POINT('Ctrl Pts',(72.9232821546964,-9.4980303780061,56.971237255248));
#166350=CARTESIAN_POINT('Ctrl Pts',(72.9909492174259,-9.49630041718572,
56.9600101630647));
#166351=CARTESIAN_POINT('Ctrl Pts',(73.4346395656196,-9.48007980871439,
56.8862665531732));
#166352=CARTESIAN_POINT('Ctrl Pts',(73.8094364466946,-9.44338615530301,
56.8233824204234));
#166353=CARTESIAN_POINT('Ctrl Pts',(74.4985605949375,-9.33315350902319,
56.7077099752523));
#166354=CARTESIAN_POINT('Ctrl Pts',(74.813291182377,-9.26582733056012,56.6548604715169));
#166355=CARTESIAN_POINT('Ctrl Pts',(75.3348497331866,-9.12551582848721,
56.5676583618627));
#166356=CARTESIAN_POINT('Ctrl Pts',(75.5436750060612,-9.061352846041,56.5328465768688));
#166357=CARTESIAN_POINT('Ctrl Pts',(75.8904674353115,-8.94126287332556,
56.4752869999921));
#166358=CARTESIAN_POINT('Ctrl Pts',(76.0296620639175,-8.88929502592799,
56.4522534085077));
#166359=CARTESIAN_POINT('Ctrl Pts',(76.2226974185921,-8.81191216675489,
56.4204189653304));
#166360=CARTESIAN_POINT('Ctrl Pts',(76.2775947265289,-8.78929373745793,
56.4113780026013));
#166361=CARTESIAN_POINT('Ctrl Pts',(76.3713879423166,-8.74959689799275,
56.3959531082265));
#166362=CARTESIAN_POINT('Ctrl Pts',(76.4103869223857,-8.73277587998832,
56.3895459944723));
#166363=CARTESIAN_POINT('Ctrl Pts',(76.4893705324138,-8.69806675157806,
56.3765831823614));
#166364=CARTESIAN_POINT('Ctrl Pts',(76.5293470450378,-8.68016215303519,
56.3700292334103));
#166365=CARTESIAN_POINT('Ctrl Pts',(76.6293506996679,-8.6345244447365,56.3536517606071));
#166366=CARTESIAN_POINT('Ctrl Pts',(76.689216708219,-8.60643147073267,56.34386364101));
#166367=CARTESIAN_POINT('Ctrl Pts',(76.9145193677493,-8.49776941214144,
56.3070868172415));
#166368=CARTESIAN_POINT('Ctrl Pts',(77.0779188610577,-8.41292555410641,
56.2805395390404));
#166369=CARTESIAN_POINT('Ctrl Pts',(77.6726651150445,-8.08146368281936,
56.1843304610601));
#166370=CARTESIAN_POINT('Ctrl Pts',(78.0871146175184,-7.80522107436626,
56.1181699073794));
#166371=CARTESIAN_POINT('Ctrl Pts',(78.6988207004769,-7.32324201516067,
56.0208311704537));
#166372=CARTESIAN_POINT('Ctrl Pts',(78.9117571459242,-7.13942939984271,
55.9870018997138));
#166373=CARTESIAN_POINT('Ctrl Pts',(79.1634469617107,-6.90166717403784,
55.9468248047271));
#166374=CARTESIAN_POINT('Ctrl Pts',(79.210197274325,-6.85657959476065,55.939353261449));
#166375=CARTESIAN_POINT('Ctrl Pts',(79.2780592614554,-6.78976208851189,
55.9284903139532));
#166376=CARTESIAN_POINT('Ctrl Pts',(79.2995346761457,-6.76841223526,55.9250500527615));
#166377=CARTESIAN_POINT('Ctrl Pts',(79.3358720275714,-6.73193711867265,
55.9192240111268));
#166378=CARTESIAN_POINT('Ctrl Pts',(79.3507859627285,-6.7168651764674,55.9168313727608));
#166379=CARTESIAN_POINT('Ctrl Pts',(79.3846905380177,-6.68236914756725,
55.911388635546));
#166380=CARTESIAN_POINT('Ctrl Pts',(79.4036485269671,-6.66291279369679,
55.9083428631627));
#166381=CARTESIAN_POINT('Ctrl Pts',(79.4558868017254,-6.60883536891432,
55.8999442308619));
#166382=CARTESIAN_POINT('Ctrl Pts',(79.4889888457069,-6.57403956121119,
55.8946153406252));
#166383=CARTESIAN_POINT('Ctrl Pts',(79.6860798861485,-6.363668962265,55.8628530117063));
#166384=CARTESIAN_POINT('Ctrl Pts',(79.84364510948,-6.18206247020525,55.8373199245345));
#166385=CARTESIAN_POINT('Ctrl Pts',(80.2619401450234,-5.66114345369423,
55.7695474550765));
#166386=CARTESIAN_POINT('Ctrl Pts',(80.5070370553553,-5.30969996049169,
55.7298698045886));
#166387=CARTESIAN_POINT('Ctrl Pts',(80.8331744871437,-4.76773514606693,
55.6780517617711));
#166388=CARTESIAN_POINT('Ctrl Pts',(80.93284726701,-4.58941656460383,55.6623778404422));
#166389=CARTESIAN_POINT('Ctrl Pts',(81.0911828028448,-4.28358834369425,
55.6378365961909));
#166390=CARTESIAN_POINT('Ctrl Pts',(81.1528662611215,-4.15777070352312,
55.6283813833674));
#166391=CARTESIAN_POINT('Ctrl Pts',(81.2363110073525,-3.97770120371416,
55.6157574560281));
#166392=CARTESIAN_POINT('Ctrl Pts',(81.2603524732508,-3.92455804778409,
55.6121416723445));
#166393=CARTESIAN_POINT('Ctrl Pts',(81.3011100503674,-3.83223604861605,
55.6060500491535));
#166394=CARTESIAN_POINT('Ctrl Pts',(81.3180511706121,-3.79316137361405,
55.603530046097));
#166395=CARTESIAN_POINT('Ctrl Pts',(81.3522411992092,-3.71284466570169,
55.5984694394092));
#166396=CARTESIAN_POINT('Ctrl Pts',(81.3694634132779,-3.67159209235742,
55.5959340529241));
#166397=CARTESIAN_POINT('Ctrl Pts',(81.412545460645,-3.56634021987553,55.589627378788));
#166398=CARTESIAN_POINT('Ctrl Pts',(81.4380070523745,-3.50217610519317,
55.5859341451506));
#166399=CARTESIAN_POINT('Ctrl Pts',(81.53558783923,-3.24834062503304,55.571917602389));
#166400=CARTESIAN_POINT('Ctrl Pts',(81.6024139697956,-3.05663616059278,
55.5626303829469));
#166401=CARTESIAN_POINT('Ctrl Pts',(81.8449420280424,-2.28312757208262,
55.5302303672368));
#166402=CARTESIAN_POINT('Ctrl Pts',(81.9716589841839,-1.68708541232549,
55.5166271718393));
#166403=CARTESIAN_POINT('Ctrl Pts',(82.0709754922155,-0.826081109782583,
55.5109108782228));
#166404=CARTESIAN_POINT('Ctrl Pts',(82.0902503395178,-0.56804435403418,
55.5109257407692));
#166405=CARTESIAN_POINT('Ctrl Pts',(82.1011744800333,-0.248408270794094,
55.5128688402182));
#166406=CARTESIAN_POINT('Ctrl Pts',(82.1026797706731,-0.187244352105316,
55.5133274666071));
#166407=CARTESIAN_POINT('Ctrl Pts',(82.104026816949,-0.0976913123765372,
55.5141224750122));
#166408=CARTESIAN_POINT('Ctrl Pts',(82.104327760441,-0.0693100533167987,
55.5143925846016));
#166409=CARTESIAN_POINT('Ctrl Pts',(82.1045868046991,-0.0272854394580932,
55.5148190559226));
#166410=CARTESIAN_POINT('Ctrl Pts',(82.1046417876626,-0.0136427461076473,
55.514961641197));
#166411=CARTESIAN_POINT('Ctrl Pts',(82.1046676540618,-6.66937018010743E-11,
55.5151083368358));
#166412=CARTESIAN_POINT('',(81.9996908076899,9.81597696801075E-5,54.9197550594462));
#166413=CARTESIAN_POINT('Ctrl Pts',(82.1125619375607,6.64456069956318E-11,
55.5598790433222));
#166414=CARTESIAN_POINT('Ctrl Pts',(82.1125360255529,-0.0136668014906386,
55.5597320890229));
#166415=CARTESIAN_POINT('Ctrl Pts',(82.1124812457219,-0.0273335719858172,
55.5595912531169));
#166416=CARTESIAN_POINT('Ctrl Pts',(82.1122237839164,-0.0693960590722018,
55.5591765377402));
#166417=CARTESIAN_POINT('Ctrl Pts',(82.1119253322823,-0.0977911812342799,
55.5589228587031));
#166418=CARTESIAN_POINT('Ctrl Pts',(82.1105894637986,-0.187432230743492,
55.55820415569));
#166419=CARTESIAN_POINT('Ctrl Pts',(82.1090966125081,-0.248670552593953,
55.5578342368826));
#166420=CARTESIAN_POINT('Ctrl Pts',(82.0982476273081,-0.569031278259053,
55.5565189630936));
#166421=CARTESIAN_POINT('Ctrl Pts',(82.0790771428474,-0.827719230267891,
55.557577764286));
#166422=CARTESIAN_POINT('Ctrl Pts',(81.9800912821575,-1.69058319990238,
55.5676174054073));
#166423=CARTESIAN_POINT('Ctrl Pts',(81.8535609968872,-2.28776150893319,
55.5852456228765));
#166424=CARTESIAN_POINT('Ctrl Pts',(81.6111483540582,-3.06075393816077,
55.6204359434127));
#166425=CARTESIAN_POINT('Ctrl Pts',(81.5448674797552,-3.25091457336205,
55.6301497961054));
#166426=CARTESIAN_POINT('Ctrl Pts',(81.4479620218375,-3.50306690856643,
55.6444344463764));
#166427=CARTESIAN_POINT('Ctrl Pts',(81.4225731932735,-3.56705957764205,
55.6481837324348));
#166428=CARTESIAN_POINT('Ctrl Pts',(81.3795794719202,-3.67210458368161,
55.6545430240807));
#166429=CARTESIAN_POINT('Ctrl Pts',(81.3623722929424,-3.71332061847222,
55.6570907175287));
#166430=CARTESIAN_POINT('Ctrl Pts',(81.3281864041571,-3.79361902625666,
55.6621570676167));
#166431=CARTESIAN_POINT('Ctrl Pts',(81.3112338122779,-3.83271162603291,
55.6646716377605));
#166432=CARTESIAN_POINT('Ctrl Pts',(81.2704072612829,-3.92515976751463,
55.6707325374166));
#166433=CARTESIAN_POINT('Ctrl Pts',(81.2463050545487,-3.97841024212875,
55.6743146204079));
#166434=CARTESIAN_POINT('Ctrl Pts',(81.1624376258653,-4.15926951853397,
55.6867927392426));
#166435=CARTESIAN_POINT('Ctrl Pts',(81.1003491686526,-4.28575489135513,
55.6960530732046));
#166436=CARTESIAN_POINT('Ctrl Pts',(80.940697981556,-4.59358539212979,55.7199290102874));
#166437=CARTESIAN_POINT('Ctrl Pts',(80.8400382007869,-4.77320404669988,
55.7350353862728));
#166438=CARTESIAN_POINT('Ctrl Pts',(80.5138828051378,-5.31344372736145,
55.7842304526298));
#166439=CARTESIAN_POINT('Ctrl Pts',(80.2701319312162,-5.66213831350987,
55.8213027277249));
#166440=CARTESIAN_POINT('Ctrl Pts',(79.8531072124986,-6.1810730799033,55.885987986311));
#166441=CARTESIAN_POINT('Ctrl Pts',(79.6950258598222,-6.36314554350392,
55.9107520212205));
#166442=CARTESIAN_POINT('Ctrl Pts',(79.4974382461152,-6.57397003278031,
55.9421495739343));
#166443=CARTESIAN_POINT('Ctrl Pts',(79.4643119514582,-6.60878211357146,
55.9474277305992));
#166444=CARTESIAN_POINT('Ctrl Pts',(79.412046315553,-6.66287934452541,55.9557794450618));
#166445=CARTESIAN_POINT('Ctrl Pts',(79.3930829798991,-6.68233933675426,
55.9588145315035));
#166446=CARTESIAN_POINT('Ctrl Pts',(79.3591744100656,-6.71683842750533,
55.9642506286868));
#166447=CARTESIAN_POINT('Ctrl Pts',(79.3442613938861,-6.73190980792745,
55.9666445346258));
#166448=CARTESIAN_POINT('Ctrl Pts',(79.3079325587747,-6.76837915527102,
55.9724835941919));
#166449=CARTESIAN_POINT('Ctrl Pts',(79.286465547779,-6.7897238808116,55.9759400913013));
#166450=CARTESIAN_POINT('Ctrl Pts',(79.2186520693956,-6.85650833587099,
55.986877235347));
#166451=CARTESIAN_POINT('Ctrl Pts',(79.1719474145352,-6.90156874971383,
55.9944363750182));
#166452=CARTESIAN_POINT('Ctrl Pts',(78.9206856817879,-7.13904600760519,
56.0352257413341));
#166453=CARTESIAN_POINT('Ctrl Pts',(78.7082496555849,-7.32262844922743,
56.0701359412207));
#166454=CARTESIAN_POINT('Ctrl Pts',(78.0983332284704,-7.80382989095364,
56.1708456612503));
#166455=CARTESIAN_POINT('Ctrl Pts',(77.6852946023917,-8.0796274366257,56.2395330219509));
#166456=CARTESIAN_POINT('Ctrl Pts',(77.0909677876752,-8.41142496431611,
56.3378098325893));
#166457=CARTESIAN_POINT('Ctrl Pts',(76.9266534935861,-8.49684137376437,
56.3649325470597));
#166458=CARTESIAN_POINT('Ctrl Pts',(76.7002583345621,-8.60608562749063,
56.4022090418431));
#166459=CARTESIAN_POINT('Ctrl Pts',(76.6402700312127,-8.63424663202308,
56.4120776684254));
#166460=CARTESIAN_POINT('Ctrl Pts',(76.5401154361674,-8.67996449625796,
56.4285388695781));
#166461=CARTESIAN_POINT('Ctrl Pts',(76.5001136913954,-8.69788376026319,
56.435109507075));
#166462=CARTESIAN_POINT('Ctrl Pts',(76.4211226249072,-8.73260063254941,
56.4480764806771));
#166463=CARTESIAN_POINT('Ctrl Pts',(76.3821418118313,-8.74941538885511,
56.454471670396));
#166464=CARTESIAN_POINT('Ctrl Pts',(76.2884654744931,-8.78906510808121,
56.4698309722384));
#166465=CARTESIAN_POINT('Ctrl Pts',(76.2336659638703,-8.81164437711394,
56.478808480221));
#166466=CARTESIAN_POINT('Ctrl Pts',(76.0413915199108,-8.8887256656826,56.5102815162446));
#166467=CARTESIAN_POINT('Ctrl Pts',(75.9028543189174,-8.94046200180463,
56.5329114272489));
#166468=CARTESIAN_POINT('Ctrl Pts',(75.5580704757652,-9.05992314015649,
56.5891247484948));
#166469=CARTESIAN_POINT('Ctrl Pts',(75.3505939047013,-9.12375718500429,
56.6228579811986));
#166470=CARTESIAN_POINT('Ctrl Pts',(74.8283151887886,-9.26460489578375,
56.7076239639697));
#166471=CARTESIAN_POINT('Ctrl Pts',(74.5113952427779,-9.33249773916729,
56.7589218462161));
#166472=CARTESIAN_POINT('Ctrl Pts',(73.8196223814295,-9.44318442541645,
56.8710530418786));
#166473=CARTESIAN_POINT('Ctrl Pts',(73.4443952264645,-9.47995599251494,
56.9319713033499));
#166474=CARTESIAN_POINT('Ctrl Pts',(73.0016358359056,-9.49621096932413,
57.0045663251759));
#166475=CARTESIAN_POINT('Ctrl Pts',(72.9351438112067,-9.49793449432923,
57.0154876508926));
#166476=CARTESIAN_POINT('Ctrl Pts',(72.8416117494996,-9.49934995670988,
57.0308820384208));
#166477=CARTESIAN_POINT('Ctrl Pts',(72.8145794909049,-9.49964053625336,
57.0353349906176));
#166478=CARTESIAN_POINT('Ctrl Pts',(72.7656245590012,-9.49995215672126,
57.0434063699352));
#166479=CARTESIAN_POINT('Ctrl Pts',(72.7437020605574,-9.50001376539328,
57.0470234166934));
#166480=CARTESIAN_POINT('Ctrl Pts',(72.6985137107118,-9.49998009980099,
57.0544847574435));
#166481=CARTESIAN_POINT('Ctrl Pts',(72.6752481499632,-9.49987497562994,
57.0583293228877));
#166482=CARTESIAN_POINT('Ctrl Pts',(72.614525992139,-9.49937145596472,57.0683710000932));
#166483=CARTESIAN_POINT('Ctrl Pts',(72.5770716807192,-9.49883327277347,
57.0745723209678));
#166484=CARTESIAN_POINT('Ctrl Pts',(72.4095009643444,-9.49540689366203,
57.1023475659263));
#166485=CARTESIAN_POINT('Ctrl Pts',(72.2794613473683,-9.48999938018888,
57.1239841525583));
#166486=CARTESIAN_POINT('Ctrl Pts',(71.904030582383,-9.46643778442168,57.1866120961271));
#166487=CARTESIAN_POINT('Ctrl Pts',(71.6592032220148,-9.44122964631399,
57.227652043293));
#166488=CARTESIAN_POINT('Ctrl Pts',(70.8056812299706,-9.31876084621198,
57.3708751745608));
#166489=CARTESIAN_POINT('Ctrl Pts',(70.2057298384782,-9.17045251366239,
57.4717045855736));
#166490=CARTESIAN_POINT('Ctrl Pts',(69.504796880521,-8.92099197253348,57.5879182777093));
#166491=CARTESIAN_POINT('Ctrl Pts',(69.3861815633877,-8.87602377153626,
57.6075325211451));
#166492=CARTESIAN_POINT('Ctrl Pts',(69.220545102184,-8.80932702504476,57.6348424277852));
#166493=CARTESIAN_POINT('Ctrl Pts',(69.1727545382097,-8.78961938390927,
57.6427126237254));
#166494=CARTESIAN_POINT('Ctrl Pts',(69.0895856639037,-8.75451003261279,
57.6563921548573));
#166495=CARTESIAN_POINT('Ctrl Pts',(69.0541366177832,-8.73928541170523,
57.6622174047591));
#166496=CARTESIAN_POINT('Ctrl Pts',(68.9797990557655,-8.70681100364406,
57.6744217166096));
#166497=CARTESIAN_POINT('Ctrl Pts',(68.9409313836164,-8.68951399426703,
57.680796185491));
#166498=CARTESIAN_POINT('Ctrl Pts',(68.8477452670836,-8.64727796026977,
57.6960631916992));
#166499=CARTESIAN_POINT('Ctrl Pts',(68.7935420454523,-8.62208019548396,
57.7049303807334));
#166500=CARTESIAN_POINT('Ctrl Pts',(68.6025315004657,-8.53104282966057,
57.7361319102404));
#166501=CARTESIAN_POINT('Ctrl Pts',(68.4670537498172,-8.46237123217672,
57.7581772140976));
#166502=CARTESIAN_POINT('Ctrl Pts',(68.1305815346606,-8.28138267081173,
57.8127287105792));
#166503=CARTESIAN_POINT('Ctrl Pts',(67.9318871771172,-8.16486140122882,
57.8447561602995));
#166504=CARTESIAN_POINT('Ctrl Pts',(67.3358376680028,-7.7851260434429,57.9403992392503));
#166505=CARTESIAN_POINT('Ctrl Pts',(66.9537402845773,-7.49867085352006,
58.0010619802806));
#166506=CARTESIAN_POINT('Ctrl Pts',(66.4786535375545,-7.08249886625802,
58.0766784000258));
#166507=CARTESIAN_POINT('Ctrl Pts',(66.3650651565212,-6.97795131916147,
58.094777363123));
#166508=CARTESIAN_POINT('Ctrl Pts',(66.2230921323951,-6.84067619280946,
58.1174733905887));
#166509=CARTESIAN_POINT('Ctrl Pts',(66.1923175456572,-6.81050848079737,
58.1223977178687));
#166510=CARTESIAN_POINT('Ctrl Pts',(66.1434427289572,-6.76193501459169,
58.1302271998457));
#166511=CARTESIAN_POINT('Ctrl Pts',(66.1252105831228,-6.74366568990208,
58.1331498983603));
#166512=CARTESIAN_POINT('Ctrl Pts',(66.0901544777273,-6.70824804413174,
58.1387738157274));
#166513=CARTESIAN_POINT('Ctrl Pts',(66.0733207557135,-6.69111004895203,
58.1414763395027));
#166514=CARTESIAN_POINT('Ctrl Pts',(66.0323816262767,-6.649110770648,58.1480532305458));
#166515=CARTESIAN_POINT('Ctrl Pts',(66.008346610756,-6.62417983030463,58.1519182391814));
#166516=CARTESIAN_POINT('Ctrl Pts',(65.9213693332408,-6.5329596392893,58.1659168384311));
#166517=CARTESIAN_POINT('Ctrl Pts',(65.8592461385075,-6.46587934785723,
58.1759383743014));
#166518=CARTESIAN_POINT('Ctrl Pts',(65.7024131566258,-6.29151872738471,
58.2012757541372));
#166519=CARTESIAN_POINT('Ctrl Pts',(65.6091341018514,-6.18295275927967,
58.2163818292685));
#166520=CARTESIAN_POINT('Ctrl Pts',(65.117094794154,-5.58328562049482,58.2960957636188));
#166521=CARTESIAN_POINT('Ctrl Pts',(64.7653396514642,-5.05472175361954,
58.3530731883585));
#166522=CARTESIAN_POINT('Ctrl Pts',(64.392566943181,-4.35233090368823,58.4111254271624));
#166523=CARTESIAN_POINT('Ctrl Pts',(64.3206750710312,-4.2082197362665,58.4221876428815));
#166524=CARTESIAN_POINT('Ctrl Pts',(64.2256324991032,-4.00506479649708,
58.4365988594911));
#166525=CARTESIAN_POINT('Ctrl Pts',(64.1994064674166,-3.94753370053154,
58.440550718768));
#166526=CARTESIAN_POINT('Ctrl Pts',(64.1578585200484,-3.8539562227327,58.4467696347737));
#166527=CARTESIAN_POINT('Ctrl Pts',(64.1421875837915,-3.81807153525195,
58.4491051738658));
#166528=CARTESIAN_POINT('Ctrl Pts',(64.109862687214,-3.7428011143,58.4539011915989));
#166529=CARTESIAN_POINT('Ctrl Pts',(64.0932511274301,-3.7033976001956,58.4563533685969));
#166530=CARTESIAN_POINT('Ctrl Pts',(64.0542313617415,-3.60908922144042,
58.4620830489079));
#166531=CARTESIAN_POINT('Ctrl Pts',(64.0320658676684,-3.55408301751158,
58.4653129782517));
#166532=CARTESIAN_POINT('Ctrl Pts',(63.9571741375909,-3.36316065001344,
58.4761380288964));
#166533=CARTESIAN_POINT('Ctrl Pts',(63.9070175956668,-3.22623048014024,
58.4832299329698));
#166534=CARTESIAN_POINT('Ctrl Pts',(63.7915698364866,-2.88743425540025,
58.4991497296821));
#166535=CARTESIAN_POINT('Ctrl Pts',(63.729787306591,-2.6844248219704,58.5072971236605));
#166536=CARTESIAN_POINT('Ctrl Pts',(63.5875153708102,-2.15479781856576,
58.5250663127387));
#166537=CARTESIAN_POINT('Ctrl Pts',(63.5172992143608,-1.8256623217694,58.532747625524));
#166538=CARTESIAN_POINT('Ctrl Pts',(63.4038724050146,-1.11306713989593,
58.5427300164016));
#166539=CARTESIAN_POINT('Ctrl Pts',(63.3661688939888,-0.729313567826545,
58.5440775717329));
#166540=CARTESIAN_POINT('Ctrl Pts',(63.3490646836895,-0.2769138713198,58.5415717179955));
#166541=CARTESIAN_POINT('Ctrl Pts',(63.3472259471866,-0.209450397333085,
58.5410918560795));
#166542=CARTESIAN_POINT('Ctrl Pts',(63.3456413777209,-0.114566163059452,
58.5402722242381));
#166543=CARTESIAN_POINT('Ctrl Pts',(63.3453011231222,-0.0871565957880548,
58.5400184778408));
#166544=CARTESIAN_POINT('Ctrl Pts',(63.3448978017111,-0.0375252792831324,
58.5395286752416));
#166545=CARTESIAN_POINT('Ctrl Pts',(63.3447944526855,-0.0153039432741772,
58.5392983690199));
#166546=CARTESIAN_POINT('Ctrl Pts',(63.3447406639745,0.0304910167184051,
58.5388012857994));
#166547=CARTESIAN_POINT('Ctrl Pts',(63.3447999067499,0.0540644024239192,
58.5385331218232));
#166548=CARTESIAN_POINT('Ctrl Pts',(63.3451812460527,0.115572764262319,
58.5378009642449));
#166549=CARTESIAN_POINT('Ctrl Pts',(63.3456415014136,0.153506224787392,
58.5373172121439));
#166550=CARTESIAN_POINT('Ctrl Pts',(63.3487039550173,0.323032355641628,
58.5350084924542));
#166551=CARTESIAN_POINT('Ctrl Pts',(63.353788490623,0.454560662918221,58.532821676005));
#166552=CARTESIAN_POINT('Ctrl Pts',(63.3762701073733,0.833987689020082,
58.5252970938101));
#166553=CARTESIAN_POINT('Ctrl Pts',(63.4005828058213,1.08134506544725,58.5188868951615));
#166554=CARTESIAN_POINT('Ctrl Pts',(63.5190153250352,1.94246850127986,58.4907628123768));
#166555=CARTESIAN_POINT('Ctrl Pts',(63.6628423739426,2.54752174277458,58.4604747325846));
#166556=CARTESIAN_POINT('Ctrl Pts',(63.9061204508566,3.258103172746,58.4102197181101));
#166557=CARTESIAN_POINT('Ctrl Pts',(63.9511751225037,3.38139949019407,58.4009440319482));
#166558=CARTESIAN_POINT('Ctrl Pts',(64.0178203776762,3.55280161797357,58.387258329664));
#166559=CARTESIAN_POINT('Ctrl Pts',(64.0373136565667,3.60173922230622,58.3832592048031));
#166560=CARTESIAN_POINT('Ctrl Pts',(64.0719475837959,3.68664740079326,58.3761602129072));
#166561=CARTESIAN_POINT('Ctrl Pts',(64.086907741873,3.72269313639632,58.3730957448931));
#166562=CARTESIAN_POINT('Ctrl Pts',(64.1187174420369,3.79803514866314,58.3665837432107));
#166563=CARTESIAN_POINT('Ctrl Pts',(64.1356103907788,3.83731140773162,58.3631276964778));
#166564=CARTESIAN_POINT('Ctrl Pts',(64.176658854597,3.93101765144412,58.3547350478729));
#166565=CARTESIAN_POINT('Ctrl Pts',(64.2010584059769,3.98533442751659,58.3497505804098));
#166566=CARTESIAN_POINT('Ctrl Pts',(64.2880222327021,4.17419769256586,58.3319999033415));
#166567=CARTESIAN_POINT('Ctrl Pts',(64.3531869243333,4.30747443543313,58.3187240848827));
#166568=CARTESIAN_POINT('Ctrl Pts',(64.5233796491981,4.63596255462977,58.2841255659868));
#166569=CARTESIAN_POINT('Ctrl Pts',(64.6321198533269,4.82907307667321,58.2620821698103));
#166570=CARTESIAN_POINT('Ctrl Pts',(64.8918203435309,5.25482656633036,58.2096626561683));
#166571=CARTESIAN_POINT('Ctrl Pts',(65.046385783662,5.48494807235221,58.1786110215429));
#166572=CARTESIAN_POINT('Ctrl Pts',(65.4069336383958,5.9739581172662,58.1067839061018));
#166573=CARTESIAN_POINT('Ctrl Pts',(65.6168242144495,6.22941413096834,58.0653392555951));
#166574=CARTESIAN_POINT('Ctrl Pts',(65.8848283569779,6.52264476239926,58.0132415429448));
#166575=CARTESIAN_POINT('Ctrl Pts',(65.9306222360787,6.57168283794933,58.0043665121508));
#166576=CARTESIAN_POINT('Ctrl Pts',(65.9978512917886,6.64214349978431,57.9913806463445));
#166577=CARTESIAN_POINT('Ctrl Pts',(66.0188755589456,6.66396555056729,57.9873256618525));
#166578=CARTESIAN_POINT('Ctrl Pts',(66.056337391677,6.7024733384773,57.980111530446));
#166579=CARTESIAN_POINT('Ctrl Pts',(66.0727328444927,6.71920059729626,57.9769579914442));
#166580=CARTESIAN_POINT('Ctrl Pts',(66.1085864471861,6.7555063847317,57.9700701468326));
#166581=CARTESIAN_POINT('Ctrl Pts',(66.1280683066891,6.77506029231369,57.9663327045083));
#166582=CARTESIAN_POINT('Ctrl Pts',(66.1842390678595,6.83094258158476,57.9555709779972));
#166583=CARTESIAN_POINT('Ctrl Pts',(66.2211396009993,6.86705134104539,57.9485184505943));
#166584=CARTESIAN_POINT('Ctrl Pts',(66.3062464979302,6.94896565995924,57.9322879421562));
#166585=CARTESIAN_POINT('Ctrl Pts',(66.3546434840923,6.9945639287013,57.923083711614));
#166586=CARTESIAN_POINT('Ctrl Pts',(66.5188730674604,7.14602711647788,57.891923372572));
#166587=CARTESIAN_POINT('Ctrl Pts',(66.6368492177105,7.2494645539054,57.8696587999886));
#166588=CARTESIAN_POINT('Ctrl Pts',(66.9930432406784,7.5462632952188,57.8026602317816));
#166589=CARTESIAN_POINT('Ctrl Pts',(67.2381163367901,7.73081873352753,57.7568401022762));
#166590=CARTESIAN_POINT('Ctrl Pts',(67.8413484825217,8.14019029590115,57.6440814531632));
#166591=CARTESIAN_POINT('Ctrl Pts',(68.2064285287763,8.35322982114183,57.575842169));
#166592=CARTESIAN_POINT('Ctrl Pts',(68.6561574217945,8.57613378851909,57.4913254979524));
#166593=CARTESIAN_POINT('Ctrl Pts',(68.728452176626,8.61080570323646,57.4777269728817));
#166594=CARTESIAN_POINT('Ctrl Pts',(68.8435449427241,8.66417823082398,57.4560570162182));
#166595=CARTESIAN_POINT('Ctrl Pts',(68.8860598592975,8.6835047066625,57.4480476894804));
#166596=CARTESIAN_POINT('Ctrl Pts',(68.9626442390345,8.71762214702849,57.4336117200641));
#166597=CARTESIAN_POINT('Ctrl Pts',(68.9966618001168,8.73253195661687,57.4271965628337));
#166598=CARTESIAN_POINT('Ctrl Pts',(69.0766629336065,8.76702391116082,57.4121026809964));
#166599=CARTESIAN_POINT('Ctrl Pts',(69.1227147726885,8.78643804609169,57.4034086681932));
#166600=CARTESIAN_POINT('Ctrl Pts',(69.2575028925935,8.84197916381548,57.3779465626433));
#166601=CARTESIAN_POINT('Ctrl Pts',(69.3466314833654,8.87709579207641,57.3610898604267));
#166602=CARTESIAN_POINT('Ctrl Pts',(69.7487432582385,9.02834969343535,57.2849522709281));
#166603=CARTESIAN_POINT('Ctrl Pts',(70.0671274266133,9.12877731614799,57.2244223562583));
#166604=CARTESIAN_POINT('Ctrl Pts',(70.8373676477867,9.32647079816782,57.0776774276926));
#166605=CARTESIAN_POINT('Ctrl Pts',(71.2923517948619,9.40736026884724,56.9907323209208));
#166606=CARTESIAN_POINT('Ctrl Pts',(71.979129529797,9.47664608914504,56.8602012104029));
#166607=CARTESIAN_POINT('Ctrl Pts',(72.2076153269439,9.49108817887239,56.8168975996582));
#166608=CARTESIAN_POINT('Ctrl Pts',(72.4817890629712,9.49813588071572,56.7652345179813));
#166609=CARTESIAN_POINT('Ctrl Pts',(72.5271525457802,9.49896532260876,56.7566964591517));
#166610=CARTESIAN_POINT('Ctrl Pts',(72.5977324290803,9.49973223228133,56.7434293398238));
#166611=CARTESIAN_POINT('Ctrl Pts',(72.6229443210239,9.49990227262387,56.7386935620761));
#166612=CARTESIAN_POINT('Ctrl Pts',(72.6695933548331,9.50002465368916,56.7299376531561));
#166613=CARTESIAN_POINT('Ctrl Pts',(72.6910298853012,9.50000578912789,56.7259166835128));
#166614=CARTESIAN_POINT('Ctrl Pts',(72.7403648739039,9.49978953698635,56.7166685481759));
#166615=CARTESIAN_POINT('Ctrl Pts',(72.7682631253118,9.49954005495001,56.7114431646031));
#166616=CARTESIAN_POINT('Ctrl Pts',(72.8562956805742,9.49835144245543,56.6949672683449));
#166617=CARTESIAN_POINT('Ctrl Pts',(72.9164250452732,9.49694854588446,56.6837323873429));
#166618=CARTESIAN_POINT('Ctrl Pts',(73.2306780699394,9.48652655700116,56.6250996199903));
#166619=CARTESIAN_POINT('Ctrl Pts',(73.4844231668491,9.4675442330946,56.5780408243862));
#166620=CARTESIAN_POINT('Ctrl Pts',(74.3311218594117,9.36873109314952,56.4213444578738));
#166621=CARTESIAN_POINT('Ctrl Pts',(74.9172950855356,9.24157334392083,56.3133137460433));
#166622=CARTESIAN_POINT('Ctrl Pts',(75.6777403911334,8.99710230269761,56.1716771819452));
#166623=CARTESIAN_POINT('Ctrl Pts',(75.8661696468452,8.9296855204103,56.1364645986918));
#166624=CARTESIAN_POINT('Ctrl Pts',(76.1156397729411,8.83116327839062,56.089656179576));
#166625=CARTESIAN_POINT('Ctrl Pts',(76.1787018474511,8.80544810603254,56.0778074029109));
#166626=CARTESIAN_POINT('Ctrl Pts',(76.2821422055465,8.76192666057605,56.0583442041768));
#166627=CARTESIAN_POINT('Ctrl Pts',(76.3226842767657,8.74452601422051,56.0507087780499));
#166628=CARTESIAN_POINT('Ctrl Pts',(76.4016160559352,8.70997669597214,56.0358293137047));
#166629=CARTESIAN_POINT('Ctrl Pts',(76.4400162399858,8.69285519987277,56.0285839615913));
#166630=CARTESIAN_POINT('Ctrl Pts',(76.53074328329,8.65165805148271,56.0114500705618));
#166631=CARTESIAN_POINT('Ctrl Pts',(76.5829666966652,8.62735314649564,56.0015753129146));
#166632=CARTESIAN_POINT('Ctrl Pts',(76.7599196486291,8.54297779475444,55.9680741110235));
#166633=CARTESIAN_POINT('Ctrl Pts',(76.8835486393362,8.48058409024693,55.944596909408));
#166634=CARTESIAN_POINT('Ctrl Pts',(77.1840346612582,8.32037460543431,55.8873681083627));
#166635=CARTESIAN_POINT('Ctrl Pts',(77.3592148871461,8.21948126215258,55.8538578264081));
#166636=CARTESIAN_POINT('Ctrl Pts',(77.8916498018825,7.88921152618273,55.751640958093));
#166637=CARTESIAN_POINT('Ctrl Pts',(78.236837012401,7.64085749729854,55.6848186048476));
#166638=CARTESIAN_POINT('Ctrl Pts',(78.748450442419,7.21699554661016,55.5857238012496));
#166639=CARTESIAN_POINT('Ctrl Pts',(78.926805324731,7.05733574788239,55.5511727688975));
#166640=CARTESIAN_POINT('Ctrl Pts',(79.1333303485869,6.85775331938775,55.5113231900014));
#166641=CARTESIAN_POINT('Ctrl Pts',(79.1674042680018,6.82432039398413,55.5047540500755));
#166642=CARTESIAN_POINT('Ctrl Pts',(79.2203949721892,6.77153081844813,55.4945485127131));
#166643=CARTESIAN_POINT('Ctrl Pts',(79.2394812566104,6.75235267674756,55.4908748507105));
#166644=CARTESIAN_POINT('Ctrl Pts',(79.2750009730927,6.71635371881951,55.4840426575004));
#166645=CARTESIAN_POINT('Ctrl Pts',(79.2914539975338,6.69955363143591,55.4808798082087));
#166646=CARTESIAN_POINT('Ctrl Pts',(79.3299256628392,6.65997575177617,55.4734884202254));
#166647=CARTESIAN_POINT('Ctrl Pts',(79.351893796531,6.63714725129234,55.4692710175102));
#166648=CARTESIAN_POINT('Ctrl Pts',(79.4241345916666,6.56131716603358,55.4554118423714));
#166649=CARTESIAN_POINT('Ctrl Pts',(79.4739170211828,6.50783286035037,55.4458765512534));
#166650=CARTESIAN_POINT('Ctrl Pts',(79.5937847596349,6.37601841968089,55.422943767704));
#166651=CARTESIAN_POINT('Ctrl Pts',(79.6632059424909,6.29707372856666,55.4096850881321));
#166652=CARTESIAN_POINT('Ctrl Pts',(79.948226373592,5.96184219810876,55.3552920956997));
#166653=CARTESIAN_POINT('Ctrl Pts',(80.1516476416783,5.69513761824494,55.3165688469124));
#166654=CARTESIAN_POINT('Ctrl Pts',(80.5914765342703,5.05018728247726,55.2322601975524));
#166655=CARTESIAN_POINT('Ctrl Pts',(80.8163592090348,4.66479907830197,55.1886603967258));
#166656=CARTESIAN_POINT('Ctrl Pts',(81.0588454266084,4.17276775217562,55.1403700966464));
#166657=CARTESIAN_POINT('Ctrl Pts',(81.1026736434647,4.0800915849361,55.1315810831492));
#166658=CARTESIAN_POINT('Ctrl Pts',(81.1666034884089,3.93906378649308,55.1186620917445));
#166659=CARTESIAN_POINT('Ctrl Pts',(81.1878107359992,3.89123780940432,55.1143588799458));
#166660=CARTESIAN_POINT('Ctrl Pts',(81.2252206886373,3.80496221223433,55.106735246783));
#166661=CARTESIAN_POINT('Ctrl Pts',(81.2415660739167,3.76657793901731,55.1033925025104));
#166662=CARTESIAN_POINT('Ctrl Pts',(81.2759447923359,3.68435290878306,55.0963361039098));
#166663=CARTESIAN_POINT('Ctrl Pts',(81.2939046120829,3.64048166784317,55.0926339834636));
#166664=CARTESIAN_POINT('Ctrl Pts',(81.3419608038894,3.52055122724325,55.0826840494763));
#166665=CARTESIAN_POINT('Ctrl Pts',(81.3714103483635,3.44422892696746,55.076537671794));
#166666=CARTESIAN_POINT('Ctrl Pts',(81.5466344001559,2.97213799971209,55.0396565448256));
#166667=CARTESIAN_POINT('Ctrl Pts',(81.667136108596,2.5671907497471,55.012878823399));
#166668=CARTESIAN_POINT('Ctrl Pts',(81.8688883039445,1.67847989412539,54.9648233998089));
#166669=CARTESIAN_POINT('Ctrl Pts',(81.9406202039826,1.19370601529443,54.945150242408));
#166670=CARTESIAN_POINT('Ctrl Pts',(81.986895659199,0.542753960261524,54.9284747858057));
#166671=CARTESIAN_POINT('Ctrl Pts',(81.9943441450247,0.379830580717261,
54.9251101533736));
#166672=CARTESIAN_POINT('Ctrl Pts',(81.9984871251316,0.177303085997581,
54.9219848611074));
#166673=CARTESIAN_POINT('Ctrl Pts',(81.9990535529322,0.13781745766436,54.9214254268815));
#166674=CARTESIAN_POINT('Ctrl Pts',(81.99952399041,0.0807122232168575,54.9206894370387));
#166675=CARTESIAN_POINT('Ctrl Pts',(81.999621128999,0.0630951403504671,
54.920472439619));
#166676=CARTESIAN_POINT('Ctrl Pts',(81.9997125061064,0.0303480227767184,
54.9200878819032));
#166677=CARTESIAN_POINT('Ctrl Pts',(81.9997193407733,0.0152281085298869,
54.9199177788824));
#166678=CARTESIAN_POINT('Ctrl Pts',(81.9996908076899,9.81597684577923E-5,
54.9197550594462));
#166679=CARTESIAN_POINT('Ctrl Pts',(81.9996908076899,9.81597696801076E-5,
54.9197550594462));
#166680=CARTESIAN_POINT('Ctrl Pts',(81.9996907396986,6.21067117015059E-5,
54.9197546717031));
#166681=CARTESIAN_POINT('Ctrl Pts',(81.9996906904331,3.60530577702464E-5,
54.9197543915294));
#166682=CARTESIAN_POINT('Ctrl Pts',(81.9996906220771,-2.94123145262016E-14,
54.9197540038636));
#166683=CARTESIAN_POINT('Origin',(73.0915550886457,-4.33680868994202E-16,
59.1075264962884));
#166684=CARTESIAN_POINT('',(81.8789250230948,-3.34120657753585E-11,54.2348582579198));
#166685=CARTESIAN_POINT('',(81.8868193065938,3.36461090144049E-11,54.2796289644064));
#166686=CARTESIAN_POINT('',(82.4472287422617,-1.59709532818419E-15,57.4578688084528));
#166687=CARTESIAN_POINT('Ctrl Pts',(81.8789250230948,-6.6822534455389E-11,
54.2348582579198));
#166688=CARTESIAN_POINT('Ctrl Pts',(81.8789508660046,0.0136303569671984,
54.2350048203439));
#166689=CARTESIAN_POINT('Ctrl Pts',(81.8789476450494,0.0272606835137892,
54.2351554847755));
#166690=CARTESIAN_POINT('Ctrl Pts',(81.8788481666303,0.0692657480702391,
54.2356325265563));
#166691=CARTESIAN_POINT('Ctrl Pts',(81.8786550368243,0.0976398929770492,
54.2359726722447));
#166692=CARTESIAN_POINT('Ctrl Pts',(81.8776486538947,0.187147359440565,
54.237103006747));
#166693=CARTESIAN_POINT('Ctrl Pts',(81.8763768729974,0.248273117906502,
54.2379593079502));
#166694=CARTESIAN_POINT('Ctrl Pts',(81.8666825031072,0.567532233263183,
54.242886293918));
#166695=CARTESIAN_POINT('Ctrl Pts',(81.8484297613539,0.825235470181819,
54.2484186926386));
#166696=CARTESIAN_POINT('Ctrl Pts',(81.7510447555305,1.6993262079535,54.2731040882037));
#166697=CARTESIAN_POINT('Ctrl Pts',(81.6226518984717,2.30836761060028,54.3005120704126));
#166698=CARTESIAN_POINT('Ctrl Pts',(81.3791622878337,3.08371269393863,54.3510731391634));
#166699=CARTESIAN_POINT('Ctrl Pts',(81.3160752599985,3.26535601010979,54.3640906268238));
#166700=CARTESIAN_POINT('Ctrl Pts',(81.2234824320398,3.5081956727569,54.3831200279833));
#166701=CARTESIAN_POINT('Ctrl Pts',(81.1986887950296,3.57121042141983,54.3882089393183));
#166702=CARTESIAN_POINT('Ctrl Pts',(81.1565472718624,3.67507700839285,54.3968484931838));
#166703=CARTESIAN_POINT('Ctrl Pts',(81.139576772074,3.71608537315862,54.4003251244743));
#166704=CARTESIAN_POINT('Ctrl Pts',(81.1057333739227,3.79628661606075,54.4072535887144));
#166705=CARTESIAN_POINT('Ctrl Pts',(81.0888821125161,3.83548784540568,54.410701173171));
#166706=CARTESIAN_POINT('Ctrl Pts',(81.048079835128,3.928686896371,54.4190436538633));
#166707=CARTESIAN_POINT('Ctrl Pts',(81.0238917826987,3.98257480078041,54.4239850429927));
#166708=CARTESIAN_POINT('Ctrl Pts',(80.9385095351167,4.16818205768405,54.441413453742));
#166709=CARTESIAN_POINT('Ctrl Pts',(80.8748362528023,4.29869237429813,54.4543863134589));
#166710=CARTESIAN_POINT('Ctrl Pts',(80.7095866810805,4.61869838952139,54.4879840030721));
#166711=CARTESIAN_POINT('Ctrl Pts',(80.6045677206145,4.80625282979567,54.5092774247772));
#166712=CARTESIAN_POINT('Ctrl Pts',(80.3478371335481,5.23042888140658,54.5611186516719));
#166713=CARTESIAN_POINT('Ctrl Pts',(80.1918445821812,5.46412296194305,54.5924708543749));
#166714=CARTESIAN_POINT('Ctrl Pts',(79.826149960122,5.9624954624937,54.6653538029573));
#166715=CARTESIAN_POINT('Ctrl Pts',(79.612231374794,6.22349694401463,54.7076090363644));
#166716=CARTESIAN_POINT('Ctrl Pts',(79.3394896120106,6.52198523683414,54.7606295719624));
#166717=CARTESIAN_POINT('Ctrl Pts',(79.2935224220743,6.57121701320449,54.7695384145081));
#166718=CARTESIAN_POINT('Ctrl Pts',(79.2260847790901,6.64190204656182,54.7825647339134));
#166719=CARTESIAN_POINT('Ctrl Pts',(79.205028934959,6.66375832683685,54.7866258512179));
#166720=CARTESIAN_POINT('Ctrl Pts',(79.1675325214451,6.70230365103613,54.7938467012514));
#166721=CARTESIAN_POINT('Ctrl Pts',(79.1511343604701,6.71903451277881,54.7970007869954));
#166722=CARTESIAN_POINT('Ctrl Pts',(79.1153016756083,6.75532088816186,54.8038846663024));
#166723=CARTESIAN_POINT('Ctrl Pts',(79.0958436690304,6.77485201336231,54.807617566779));
#166724=CARTESIAN_POINT('Ctrl Pts',(79.0398099107747,6.83060189973919,54.818353156453));
#166725=CARTESIAN_POINT('Ctrl Pts',(79.0030241224877,6.86660271053121,54.825383874013));
#166726=CARTESIAN_POINT('Ctrl Pts',(78.6788861540233,7.17863476839374,54.8872007384371));
#166727=CARTESIAN_POINT('Ctrl Pts',(78.3747179465517,7.43614432683576,54.9443111089608));
#166728=CARTESIAN_POINT('Ctrl Pts',(77.6348460892549,7.98554888392823,55.0827817430526));
#166729=CARTESIAN_POINT('Ctrl Pts',(77.1893145608434,8.26150667456777,55.1658837232267));
#166730=CARTESIAN_POINT('Ctrl Pts',(76.644500425792,8.53846395991299,55.2681980457221));
#166731=CARTESIAN_POINT('Ctrl Pts',(76.5648424787215,8.57753079452375,55.2831719879763));
#166732=CARTESIAN_POINT('Ctrl Pts',(76.4365305345214,8.63819122410475,55.307317617881));
#166733=CARTESIAN_POINT('Ctrl Pts',(76.3882182924372,8.66052411349516,55.3164147294697));
#166734=CARTESIAN_POINT('Ctrl Pts',(76.3018910505516,8.69953078205289,55.3326806672048));
#166735=CARTESIAN_POINT('Ctrl Pts',(76.2639488028959,8.71636864761554,55.3398334464921));
#166736=CARTESIAN_POINT('Ctrl Pts',(76.1841860456536,8.75112546027824,55.3548778877595));
#166737=CARTESIAN_POINT('Ctrl Pts',(76.1423447996391,8.76899202374362,55.3627742065991));
#166738=CARTESIAN_POINT('Ctrl Pts',(76.0316160511195,8.81531180539807,55.3836828688425));
#166739=CARTESIAN_POINT('Ctrl Pts',(75.9625211060265,8.84323920870426,55.3967419332811));
#166740=CARTESIAN_POINT('Ctrl Pts',(75.6190326135437,8.97726592596113,55.4617208538378));
#166741=CARTESIAN_POINT('Ctrl Pts',(75.3401900846677,9.07099204479333,55.5146624714897));
#166742=CARTESIAN_POINT('Ctrl Pts',(74.7226909777175,9.24617518968099,55.6321860828827));
#166743=CARTESIAN_POINT('Ctrl Pts',(74.3829665550192,9.32204832449705,55.6970261548631));
#166744=CARTESIAN_POINT('Ctrl Pts',(73.6586800511553,9.44112818631614,55.8351096031619));
#166745=CARTESIAN_POINT('Ctrl Pts',(73.2740190077182,9.47965912719769,55.908354911667));
#166746=CARTESIAN_POINT('Ctrl Pts',(72.8206254254149,9.49629982567009,55.9939291275275));
#166747=CARTESIAN_POINT('Ctrl Pts',(72.7532121337388,9.49803009235094,56.0066327416));
#166748=CARTESIAN_POINT('Ctrl Pts',(72.6594695466927,9.49940224190416,56.0242651810636));
#166749=CARTESIAN_POINT('Ctrl Pts',(72.6331548481899,9.49967420555681,56.029211234575));
#166750=CARTESIAN_POINT('Ctrl Pts',(72.5851539572848,9.49996380503658,56.0382264425493));
#166751=CARTESIAN_POINT('Ctrl Pts',(72.563468330438,9.50001777653254,56.0422967064649));
#166752=CARTESIAN_POINT('Ctrl Pts',(72.5183241916775,9.49997012928969,56.0507643910986));
#166753=CARTESIAN_POINT('Ctrl Pts',(72.494865876502,9.4998554390896,56.0551613488345));
#166754=CARTESIAN_POINT('Ctrl Pts',(72.4328169921833,9.49931420144246,56.0667837963582));
#166755=CARTESIAN_POINT('Ctrl Pts',(72.3942272601592,9.49873421122485,56.074004089741));
#166756=CARTESIAN_POINT('Ctrl Pts',(72.212215595854,9.49485056124079,56.1080248922559));
#166757=CARTESIAN_POINT('Ctrl Pts',(72.0688606116671,9.48842873925612,56.1347198674065));
#166758=CARTESIAN_POINT('Ctrl Pts',(71.6367381851645,9.45891417901261,56.214991945299));
#166759=CARTESIAN_POINT('Ctrl Pts',(71.3487921177771,9.42552022242463,56.2682205815093));
#166760=CARTESIAN_POINT('Ctrl Pts',(70.477500788138,9.28248547054327,56.4292516546246));
#166761=CARTESIAN_POINT('Ctrl Pts',(69.9024915634766,9.12994561566432,56.5355711132637));
#166762=CARTESIAN_POINT('Ctrl Pts',(69.2504703161442,8.88758425827938,56.6576107863682));
#166763=CARTESIAN_POINT('Ctrl Pts',(69.1557154533756,8.85056859462303,56.6753811452198));
#166764=CARTESIAN_POINT('Ctrl Pts',(69.0136207885224,8.79233426904305,56.7020855992691));
#166765=CARTESIAN_POINT('Ctrl Pts',(68.9658254879533,8.77227470960467,56.7110776401391));
#166766=CARTESIAN_POINT('Ctrl Pts',(68.8802976518815,8.73552890277593,56.7271861877469));
#166767=CARTESIAN_POINT('Ctrl Pts',(68.8425044647696,8.71899080427367,56.7343105009408));
#166768=CARTESIAN_POINT('Ctrl Pts',(68.7620896460758,8.68315799340499,56.7494827299075));
#166769=CARTESIAN_POINT('Ctrl Pts',(68.7195005396518,8.66379129253889,56.7575263107204));
#166770=CARTESIAN_POINT('Ctrl Pts',(68.6039790183743,8.61019743373174,56.7793663172837));
#166771=CARTESIAN_POINT('Ctrl Pts',(68.5313380471226,8.57533606817214,56.7931236518591));
#166772=CARTESIAN_POINT('Ctrl Pts',(68.0422632332377,8.33270913423026,56.8859096946526));
#166773=CARTESIAN_POINT('Ctrl Pts',(67.6412496836092,8.09456302332125,56.9628307255044));
#166774=CARTESIAN_POINT('Ctrl Pts',(66.8761160733876,7.55861129633076,57.1105089703873));
#166775=CARTESIAN_POINT('Ctrl Pts',(66.5131986017449,7.26134116772372,57.181029454186));
#166776=CARTESIAN_POINT('Ctrl Pts',(66.1285695959665,6.89494726396894,57.2552998206332));
#166777=CARTESIAN_POINT('Ctrl Pts',(66.0840576129619,6.85169835870725,57.2638865848842));
#166778=CARTESIAN_POINT('Ctrl Pts',(66.018880305953,6.78710705952695,57.2764435905706));
#166779=CARTESIAN_POINT('Ctrl Pts',(65.9978903534727,6.76610846235605,57.2804849518767));
#166780=CARTESIAN_POINT('Ctrl Pts',(65.9605716806631,6.72842034416463,57.2876651197337));
#166781=CARTESIAN_POINT('Ctrl Pts',(65.9442060142965,6.71176956620389,57.2908120948118));
#166782=CARTESIAN_POINT('Ctrl Pts',(65.9080189807995,6.67467790672599,57.2977664908289));
#166783=CARTESIAN_POINT('Ctrl Pts',(65.8882275018205,6.65420727582768,57.3015673358906));
#166784=CARTESIAN_POINT('Ctrl Pts',(65.8298843045737,6.59331328404003,57.3127647233032));
#166785=CARTESIAN_POINT('Ctrl Pts',(65.7915930315932,6.55263170475197,57.3201044215832));
#166786=CARTESIAN_POINT('Ctrl Pts',(65.7036437432867,6.45751566453136,57.3369457177357));
#166787=CARTESIAN_POINT('Ctrl Pts',(65.6542518903138,6.40283016526812,57.3463909284866));
#166788=CARTESIAN_POINT('Ctrl Pts',(65.4839238826797,6.20975557944587,57.3789336382707));
#166789=CARTESIAN_POINT('Ctrl Pts',(65.3663295438945,6.06836020886151,57.4013491856481));
#166790=CARTESIAN_POINT('Ctrl Pts',(64.8772381868979,5.44413425101124,57.4946297629701));
#166791=CARTESIAN_POINT('Ctrl Pts',(64.5481196569545,4.92880109143663,57.5576414547113));
#166792=CARTESIAN_POINT('Ctrl Pts',(64.2107475951982,4.26792608278854,57.6244488516881));
#166793=CARTESIAN_POINT('Ctrl Pts',(64.1534999542628,4.14981654154612,57.635879660366));
#166794=CARTESIAN_POINT('Ctrl Pts',(64.0768142638135,3.98289882691513,57.6513384508323));
#166795=CARTESIAN_POINT('Ctrl Pts',(64.0553218750463,3.93508125841348,57.6556884524486));
#166796=CARTESIAN_POINT('Ctrl Pts',(64.018543749879,3.85141575252323,57.663163629565));
#166797=CARTESIAN_POINT('Ctrl Pts',(64.0030821473655,3.81564900553301,57.6663163365184));
#166798=CARTESIAN_POINT('Ctrl Pts',(63.9710912080004,3.74038218419297,57.6728611764342));
#166799=CARTESIAN_POINT('Ctrl Pts',(63.9546075388912,3.70086303365946,57.6762461411081));
#166800=CARTESIAN_POINT('Ctrl Pts',(63.9157119534642,3.60581571198785,57.6842644662583));
#166801=CARTESIAN_POINT('Ctrl Pts',(63.8935544206719,3.55018210214804,57.6888579456023));
#166802=CARTESIAN_POINT('Ctrl Pts',(63.8177631276299,3.35454759700674,57.7046625521922));
#166803=CARTESIAN_POINT('Ctrl Pts',(63.7668931790818,3.21346542895748,57.7154398678302));
#166804=CARTESIAN_POINT('Ctrl Pts',(63.6494138935544,2.86193791026962,57.7407665878182));
#166805=CARTESIAN_POINT('Ctrl Pts',(63.5867159741442,2.65023492558059,57.7546944865716));
#166806=CARTESIAN_POINT('Ctrl Pts',(63.4497907887842,2.12145917454508,57.7861633185172));
#166807=CARTESIAN_POINT('Ctrl Pts',(63.3842687511748,1.802339396006,57.802273113305));
#166808=CARTESIAN_POINT('Ctrl Pts',(63.2774695783862,1.10411678499286,57.8309157425616));
#166809=CARTESIAN_POINT('Ctrl Pts',(63.242246431142,0.724605983936422,57.8423618071329));
#166810=CARTESIAN_POINT('Ctrl Pts',(63.2271978994398,0.276578358908958,
57.8504831423012));
#166811=CARTESIAN_POINT('Ctrl Pts',(63.2256384359945,0.20921276297513,57.8515609702238));
#166812=CARTESIAN_POINT('Ctrl Pts',(63.2244325871052,0.114443402103744,
57.8528712535952));
#166813=CARTESIAN_POINT('Ctrl Pts',(63.2242001055327,0.0870507833191807,
57.8532257840577));
#166814=CARTESIAN_POINT('Ctrl Pts',(63.2239891749179,0.0374407803890094,
57.8538236394618));
#166815=CARTESIAN_POINT('Ctrl Pts',(63.2239710200176,0.0152238079495488,
57.8540753146484));
#166816=CARTESIAN_POINT('Ctrl Pts',(63.2240908527852,-0.0305740576833721,
57.8545607719944));
#166817=CARTESIAN_POINT('Ctrl Pts',(63.2242384963419,-0.0541547116533171,
57.8547925284985));
#166818=CARTESIAN_POINT('Ctrl Pts',(63.2248482682202,-0.115703330649285,
57.8553503408347));
#166819=CARTESIAN_POINT('Ctrl Pts',(63.2254473154192,-0.153669774989378,
57.8556476406131));
#166820=CARTESIAN_POINT('Ctrl Pts',(63.2291261640653,-0.323566157002608,
57.8567714442158));
#166821=CARTESIAN_POINT('Ctrl Pts',(63.2346757240404,-0.45543129779514,
57.8570862083068));
#166822=CARTESIAN_POINT('Ctrl Pts',(63.2585072584479,-0.836210276788409,
57.8564562225438));
#166823=CARTESIAN_POINT('Ctrl Pts',(63.2837192864116,-1.08457650910745,
57.854141361867));
#166824=CARTESIAN_POINT('Ctrl Pts',(63.4057142023206,-1.95065142595822,
57.8399114145395));
#166825=CARTESIAN_POINT('Ctrl Pts',(63.5528278126081,-2.5594944699328,57.8189341717185));
#166826=CARTESIAN_POINT('Ctrl Pts',(63.799933403572,-3.26994464349393,57.7827457278398));
#166827=CARTESIAN_POINT('Ctrl Pts',(63.8442901636461,-3.38970248143127,
57.7762206907059));
#166828=CARTESIAN_POINT('Ctrl Pts',(63.910102680954,-3.55703314062706,57.7665067173512));
#166829=CARTESIAN_POINT('Ctrl Pts',(63.9295784938296,-3.60538753336158,
57.7636283627451));
#166830=CARTESIAN_POINT('Ctrl Pts',(63.9642883780948,-3.68957338063784,
57.7584924442084));
#166831=CARTESIAN_POINT('Ctrl Pts',(63.9793484767071,-3.72547684665783,
57.7562621341555));
#166832=CARTESIAN_POINT('Ctrl Pts',(64.0114870623206,-3.80080308331473,
57.7514987007274));
#166833=CARTESIAN_POINT('Ctrl Pts',(64.0286126685412,-3.84020432716331,
57.7489581957445));
#166834=CARTESIAN_POINT('Ctrl Pts',(64.0704611014992,-3.9347382020334,57.7427449037923));
#166835=CARTESIAN_POINT('Ctrl Pts',(64.095441170743,-3.98975222340022,57.7390318203278));
#166836=CARTESIAN_POINT('Ctrl Pts',(64.1858828772381,-4.18401965148234,
57.7255731682155));
#166837=CARTESIAN_POINT('Ctrl Pts',(64.2541720748244,-4.32189891649985,
57.7153841908847));
#166838=CARTESIAN_POINT('Ctrl Pts',(64.4344032182216,-4.66471479959257,
57.6884125803448));
#166839=CARTESIAN_POINT('Ctrl Pts',(64.5505679328568,-4.86726166506303,
57.67095970094));
#166840=CARTESIAN_POINT('Ctrl Pts',(64.9143587859409,-5.45086637805468,
57.6159660764193));
#166841=CARTESIAN_POINT('Ctrl Pts',(65.1817916778534,-5.81847493084467,
57.5751548378277));
#166842=CARTESIAN_POINT('Ctrl Pts',(65.5860218602254,-6.2980178523416,57.512028204186));
#166843=CARTESIAN_POINT('Ctrl Pts',(65.7015127419095,-6.42764553183768,
57.4938487010207));
#166844=CARTESIAN_POINT('Ctrl Pts',(65.851135055557,-6.58659621003425,57.4700543735663));
#166845=CARTESIAN_POINT('Ctrl Pts',(65.8820636022155,-6.61899071049763,
57.4651233376893));
#166846=CARTESIAN_POINT('Ctrl Pts',(65.9314302114396,-6.66997022017942,
57.4572314643077));
#166847=CARTESIAN_POINT('Ctrl Pts',(65.9497204995777,-6.68870239658131,
57.4543029913016));
#166848=CARTESIAN_POINT('Ctrl Pts',(65.98482548799,-6.72435923515315,57.4486732803684));
#166849=CARTESIAN_POINT('Ctrl Pts',(66.0016270908808,-6.74129674603194,
57.4459748986392));
#166850=CARTESIAN_POINT('Ctrl Pts',(66.0423032481958,-6.7819937906323,57.4394330363391));
#166851=CARTESIAN_POINT('Ctrl Pts',(66.0662397327312,-6.80568880243069,
57.4355758544385));
#166852=CARTESIAN_POINT('Ctrl Pts',(66.1510767222687,-6.88877953741214,
57.4218802231341));
#166853=CARTESIAN_POINT('Ctrl Pts',(66.2126381165621,-6.94747069852206,
57.4118974564689));
#166854=CARTESIAN_POINT('Ctrl Pts',(66.3697235215974,-7.09324053084566,
57.3863315077649));
#166855=CARTESIAN_POINT('Ctrl Pts',(66.4662387860024,-7.17918813222846,
57.3705392866961));
#166856=CARTESIAN_POINT('Ctrl Pts',(66.8226848109313,-7.48371188821404,
57.3120017759671));
#166857=CARTESIAN_POINT('Ctrl Pts',(67.0924232362203,-7.69002369457173,
57.2673112570304));
#166858=CARTESIAN_POINT('Ctrl Pts',(67.7330514449455,-8.12706783224505,
57.1611200938878));
#166859=CARTESIAN_POINT('Ctrl Pts',(68.1099820083774,-8.3472931988225,57.0986200697327));
#166860=CARTESIAN_POINT('Ctrl Pts',(68.572937582603,-8.57588874047639,57.022337612544));
#166861=CARTESIAN_POINT('Ctrl Pts',(68.6456349821064,-8.61061877632187,
57.0103713625155));
#166862=CARTESIAN_POINT('Ctrl Pts',(68.761335089652,-8.66405918847396,56.991347881987));
#166863=CARTESIAN_POINT('Ctrl Pts',(68.8040493230036,-8.68339801219653,
56.9843292796573));
#166864=CARTESIAN_POINT('Ctrl Pts',(68.8809730484611,-8.71752688355916,
56.9716978500219));
#166865=CARTESIAN_POINT('Ctrl Pts',(68.9151296580056,-8.73243618537735,
56.9660920056517));
#166866=CARTESIAN_POINT('Ctrl Pts',(68.9954306651665,-8.76691437155132,
56.9529197992289));
#166867=CARTESIAN_POINT('Ctrl Pts',(69.0416442329359,-8.78631575851614,
56.945344481617));
#166868=CARTESIAN_POINT('Ctrl Pts',(69.1768076770679,-8.84177898334242,
56.9232042080925));
#166869=CARTESIAN_POINT('Ctrl Pts',(69.2661546972328,-8.8768351787469,56.9085885694714));
#166870=CARTESIAN_POINT('Ctrl Pts',(69.668656250943,-9.02760907878606,56.8428324364613));
#166871=CARTESIAN_POINT('Ctrl Pts',(69.9872709841347,-9.12774497602621,
56.7910234223515));
#166872=CARTESIAN_POINT('Ctrl Pts',(70.7583380200208,-9.3251187602244,56.6659505502013));
#166873=CARTESIAN_POINT('Ctrl Pts',(71.2139725588415,-9.40608131811315,
56.5923038522454));
#166874=CARTESIAN_POINT('Ctrl Pts',(71.905278372099,-9.47622086434692,56.4798698227964));
#166875=CARTESIAN_POINT('Ctrl Pts',(72.137765776598,-9.49097891025053,56.4419340118233));
#166876=CARTESIAN_POINT('Ctrl Pts',(72.4161768506161,-9.49812560012054,
56.3961994513083));
#166877=CARTESIAN_POINT('Ctrl Pts',(72.4618485953898,-9.49895958954531,
56.3886870813714));
#166878=CARTESIAN_POINT('Ctrl Pts',(72.5328611950074,-9.49973027753006,
56.3769894532961));
#166879=CARTESIAN_POINT('Ctrl Pts',(72.5582000897494,-9.49990115301473,
56.3728121031914));
#166880=CARTESIAN_POINT('Ctrl Pts',(72.6050549047792,-9.50002458677341,
56.3650810705607));
#166881=CARTESIAN_POINT('Ctrl Pts',(72.6265705365697,-9.50000619111442,
56.3615283937108));
#166882=CARTESIAN_POINT('Ctrl Pts',(72.6760506237442,-9.49979122403217,
56.353352328916));
#166883=CARTESIAN_POINT('Ctrl Pts',(72.7040142774998,-9.49954289160944,
56.3487273478871));
#166884=CARTESIAN_POINT('Ctrl Pts',(72.7921228119273,-9.49836072462214,
56.3341422164764));
#166885=CARTESIAN_POINT('Ctrl Pts',(72.8522578038061,-9.49696688788121,
56.3241691651579));
#166886=CARTESIAN_POINT('Ctrl Pts',(73.1655560201388,-9.48664529258244,
56.2721275853992));
#166887=CARTESIAN_POINT('Ctrl Pts',(73.418256203661,-9.46790243833621,56.2298721608435));
#166888=CARTESIAN_POINT('Ctrl Pts',(74.3217552675573,-9.36341829631492,
56.0784405319889));
#166889=CARTESIAN_POINT('Ctrl Pts',(74.9639264179844,-9.21882131945944,
55.9702888207293));
#166890=CARTESIAN_POINT('Ctrl Pts',(75.7365165269794,-8.95629819664322,
55.8419655296463));
#166891=CARTESIAN_POINT('Ctrl Pts',(75.885553953018,-8.90135911607756,55.8172890738096));
#166892=CARTESIAN_POINT('Ctrl Pts',(76.0913875267459,-8.81944087105524,
55.7833319445627));
#166893=CARTESIAN_POINT('Ctrl Pts',(76.149387730611,-8.79567689567379,55.7737772346591));
#166894=CARTESIAN_POINT('Ctrl Pts',(76.2428939701221,-8.75625881280899,
55.7583962853958));
#166895=CARTESIAN_POINT('Ctrl Pts',(76.2785451965742,-8.74096704708965,
55.7525374033601));
#166896=CARTESIAN_POINT('Ctrl Pts',(76.3529119105924,-8.70851815904882,
55.7403275109274));
#166897=CARTESIAN_POINT('Ctrl Pts',(76.3916086373921,-8.69131870456047,
55.7339806309303));
#166898=CARTESIAN_POINT('Ctrl Pts',(76.4836535109801,-8.64965481823642,
55.7188994579816));
#166899=CARTESIAN_POINT('Ctrl Pts',(76.5368937939655,-8.62494794706429,
55.7101888993659));
#166900=CARTESIAN_POINT('Ctrl Pts',(76.7205047765371,-8.5376267954686,55.6801921840591));
#166901=CARTESIAN_POINT('Ctrl Pts',(76.8496855113463,-8.47247084083345,
55.6591648638758));
#166902=CARTESIAN_POINT('Ctrl Pts',(77.1666748686668,-8.30324721147573,
55.6077474973792));
#166903=CARTESIAN_POINT('Ctrl Pts',(77.3525625007767,-8.19563834196867,
55.5777583106651));
#166904=CARTESIAN_POINT('Ctrl Pts',(77.773915924229,-7.93197952498977,55.5100781517785));
#166905=CARTESIAN_POINT('Ctrl Pts',(78.0064282629588,-7.77145640037084,
55.4729586453456));
#166906=CARTESIAN_POINT('Ctrl Pts',(78.4972544724062,-7.3988314658469,55.3947947015783));
#166907=CARTESIAN_POINT('Ctrl Pts',(78.7522817881167,-7.18291270359349,
55.3543111075302));
#166908=CARTESIAN_POINT('Ctrl Pts',(79.0444484044455,-6.90755413542126,
55.3076787877871));
#166909=CARTESIAN_POINT('Ctrl Pts',(79.0929805906219,-6.86082047728686,
55.2999233264019));
#166910=CARTESIAN_POINT('Ctrl Pts',(79.1626827439834,-6.79224426083568,
55.2887664892603));
#166911=CARTESIAN_POINT('Ctrl Pts',(79.1842508306468,-6.77081806001443,
55.2853115947057));
#166912=CARTESIAN_POINT('Ctrl Pts',(79.2222974921599,-6.73265380900773,
55.2792118733245));
#166913=CARTESIAN_POINT('Ctrl Pts',(79.2388174258855,-6.71595836491827,
55.2765615784987));
#166914=CARTESIAN_POINT('Ctrl Pts',(79.2746581365841,-6.67946481788585,
55.2708076326853));
#166915=CARTESIAN_POINT('Ctrl Pts',(79.2939546116864,-6.65964294332387,
55.2677072283126));
#166916=CARTESIAN_POINT('Ctrl Pts',(79.349064453543,-6.60253154610103,55.2588461209575));
#166917=CARTESIAN_POINT('Ctrl Pts',(79.3846608724563,-6.56502956540398,
55.2531146342129));
#166918=CARTESIAN_POINT('Ctrl Pts',(79.465389928753,-6.47856590752355,55.2401016001979));
#166919=CARTESIAN_POINT('Ctrl Pts',(79.5103183369713,-6.42941302455843,
55.2328487405332));
#166920=CARTESIAN_POINT('Ctrl Pts',(79.6594406695574,-6.2627632297597,55.2087507656911));
#166921=CARTESIAN_POINT('Ctrl Pts',(79.7612488871114,-6.14311641577636,
55.1922572283434));
#166922=CARTESIAN_POINT('Ctrl Pts',(80.0543689978334,-5.78074472302806,
55.144765871526));
#166923=CARTESIAN_POINT('Ctrl Pts',(80.2369286860602,-5.53102845992008,
55.1151872839117));
#166924=CARTESIAN_POINT('Ctrl Pts',(80.6416529865645,-4.91675761972446,
55.0502225694924));
#166925=CARTESIAN_POINT('Ctrl Pts',(80.8522504426097,-4.54517360435976,
55.0169562099889));
#166926=CARTESIAN_POINT('Ctrl Pts',(81.0727673905489,-4.08738135198437,
54.9832929442761));
#166927=CARTESIAN_POINT('Ctrl Pts',(81.1070600590357,-4.0138196860199,54.9780972737369));
#166928=CARTESIAN_POINT('Ctrl Pts',(81.1598593454323,-3.89670774517398,
54.9701633855689));
#166929=CARTESIAN_POINT('Ctrl Pts',(81.1789803206142,-3.85344709032269,
54.9673046508416));
#166930=CARTESIAN_POINT('Ctrl Pts',(81.212739221421,-3.77551870705794,54.9622841303363));
#166931=CARTESIAN_POINT('Ctrl Pts',(81.2274938012511,-3.74090409293813,
54.9600994412905));
#166932=CARTESIAN_POINT('Ctrl Pts',(81.2616301531713,-3.65949864970567,
54.9550677879093));
#166933=CARTESIAN_POINT('Ctrl Pts',(81.2808470409104,-3.61263794347518,
54.9522531477322));
#166934=CARTESIAN_POINT('Ctrl Pts',(81.3358316311714,-3.4754832274807,54.9442531137681));
#166935=CARTESIAN_POINT('Ctrl Pts',(81.370607811285,-3.38478754374128,54.9392619836735));
#166936=CARTESIAN_POINT('Ctrl Pts',(81.5204426026143,-2.97561239319266,
54.9180758590559));
#166937=CARTESIAN_POINT('Ctrl Pts',(81.620085289815,-2.65159856779745,54.9048957123404));
#166938=CARTESIAN_POINT('Ctrl Pts',(81.8166384341606,-1.86766018835391,
54.8811676500175));
#166939=CARTESIAN_POINT('Ctrl Pts',(81.89745242237,-1.40452788131614,54.873636527431));
#166940=CARTESIAN_POINT('Ctrl Pts',(81.9673237249124,-0.705470294435794,
54.8707509279738));
#166941=CARTESIAN_POINT('Ctrl Pts',(81.9820710223955,-0.472851133707171,
54.8711671834158));
#166942=CARTESIAN_POINT('Ctrl Pts',(81.9895821453053,-0.193782710685954,
54.8731626969154));
#166943=CARTESIAN_POINT('Ctrl Pts',(81.9904913381543,-0.14762222435378,
54.8735416781741));
#166944=CARTESIAN_POINT('Ctrl Pts',(81.9913872782568,-0.0758064403519598,
54.8742057332032));
#166945=CARTESIAN_POINT('Ctrl Pts',(81.9916043944257,-0.0501544171433835,
54.8744577003677));
#166946=CARTESIAN_POINT('Ctrl Pts',(81.9917549332481,-0.0163346478941346,
54.8748091295772));
#166947=CARTESIAN_POINT('Ctrl Pts',(81.9917808534907,-0.00816731848436852,
54.8748954770821));
#166948=CARTESIAN_POINT('Ctrl Pts',(81.9917963385783,-6.66906343255317E-11,
54.8749832973778));
#166949=CARTESIAN_POINT('Ctrl Pts',(81.9996906220771,-2.94123145262016E-14,
54.9197540038636));
#166950=CARTESIAN_POINT('Ctrl Pts',(81.9996543914623,-0.0191091568433552,
54.9195485298366));
#166951=CARTESIAN_POINT('Ctrl Pts',(81.9995617236469,-0.0382182903653823,
54.9193550169557));
#166952=CARTESIAN_POINT('Ctrl Pts',(81.9992250716837,-0.0813586940964622,
54.9189449652443));
#166953=CARTESIAN_POINT('Ctrl Pts',(81.998948257421,-0.105389644357322,
54.9187353385));
#166954=CARTESIAN_POINT('Ctrl Pts',(81.9976699366931,-0.189291046894798,
54.9180684917672));
#166955=CARTESIAN_POINT('Ctrl Pts',(81.9962033782377,-0.249153755475308,
54.9177083467591));
#166956=CARTESIAN_POINT('Ctrl Pts',(81.9765111417756,-0.832234119781761,
54.9153034916425));
#166957=CARTESIAN_POINT('Ctrl Pts',(81.916471825102,-1.35317638216592,54.9217658501432));
#166958=CARTESIAN_POINT('Ctrl Pts',(81.7467604813164,-2.20695625026125,
54.9444969621447));
#166959=CARTESIAN_POINT('Ctrl Pts',(81.6607438020665,-2.54341034204183,
54.9567229066047));
#166960=CARTESIAN_POINT('Ctrl Pts',(81.4957573764999,-3.06835540692492,
54.9806785851731));
#166961=CARTESIAN_POINT('Ctrl Pts',(81.4286432669879,-3.26032648788813,
54.990516751523));
#166962=CARTESIAN_POINT('Ctrl Pts',(81.3313881941951,-3.51244678510232,
55.0048560190491));
#166963=CARTESIAN_POINT('Ctrl Pts',(81.3066352655041,-3.57466324886592,
55.0085119394264));
#166964=CARTESIAN_POINT('Ctrl Pts',(81.2644378631296,-3.67756889565411,
55.0147540431852));
#166965=CARTESIAN_POINT('Ctrl Pts',(81.2473590268853,-3.71840882687804,
55.0172829427844));
#166966=CARTESIAN_POINT('Ctrl Pts',(81.213383603913,-3.79809440488792,55.0223184600511));
#166967=CARTESIAN_POINT('Ctrl Pts',(81.1965111046936,-3.83694943494383,
55.0248213091283));
#166968=CARTESIAN_POINT('Ctrl Pts',(81.1553419359743,-3.93005810722302,
55.0309334200571));
#166969=CARTESIAN_POINT('Ctrl Pts',(81.1307973304866,-3.98419758370011,
55.0345815198751));
#166970=CARTESIAN_POINT('Ctrl Pts',(81.048244816237,-4.16186306782704,55.0468651111836));
#166971=CARTESIAN_POINT('Ctrl Pts',(80.9881051081548,-4.28435615803449,
55.0558349363848));
#166972=CARTESIAN_POINT('Ctrl Pts',(80.6459579998245,-4.945075460852,55.1069994707986));
#166973=CARTESIAN_POINT('Ctrl Pts',(80.3159163833134,-5.45624295152242,
55.1567068571896));
#166974=CARTESIAN_POINT('Ctrl Pts',(79.8271913890805,-6.07474322030209,
55.23234459434));
#166975=CARTESIAN_POINT('Ctrl Pts',(79.7103117904494,-6.21423415781569,
55.2505666829455));
#166976=CARTESIAN_POINT('Ctrl Pts',(79.540903388712,-6.40502026328512,55.277238177257));
#166977=CARTESIAN_POINT('Ctrl Pts',(79.4916251198374,-6.45924054320261,
55.2850257121151));
#166978=CARTESIAN_POINT('Ctrl Pts',(79.4038210992298,-6.5536335452002,55.2989594850689));
#166979=CARTESIAN_POINT('Ctrl Pts',(79.3655558433369,-6.59405186600855,
55.3050506489884));
#166980=CARTESIAN_POINT('Ctrl Pts',(79.3071826448708,-6.65463391888389,
55.3143735982192));
#166981=CARTESIAN_POINT('Ctrl Pts',(79.2873312859905,-6.67505178618935,
55.31754942982));
#166982=CARTESIAN_POINT('Ctrl Pts',(79.2509923349751,-6.71209285138234,
55.323373061447));
#166983=CARTESIAN_POINT('Ctrl Pts',(79.2345341758204,-6.72874530394705,
55.3260143979054));
#166984=CARTESIAN_POINT('Ctrl Pts',(79.1969493636204,-6.76649338762336,
55.3320547916534));
#166985=CARTESIAN_POINT('Ctrl Pts',(79.175785211435,-6.78754975194111,55.335462149535));
#166986=CARTESIAN_POINT('Ctrl Pts',(79.1098791566091,-6.85250373441439,
55.3460902980748));
#166987=CARTESIAN_POINT('Ctrl Pts',(79.0648070478237,-6.89605196577429,
55.3533834840511));
#166988=CARTESIAN_POINT('Ctrl Pts',(78.677979981765,-7.2624456188471,55.4161606131424));
#166989=CARTESIAN_POINT('Ctrl Pts',(78.3134652438269,-7.55945831821165,
55.476492495436));
#166990=CARTESIAN_POINT('Ctrl Pts',(77.5452291460069,-8.09494620565633,
55.6038128585436));
#166991=CARTESIAN_POINT('Ctrl Pts',(77.1427291606947,-8.33288452715957,
55.6705895957359));
#166992=CARTESIAN_POINT('Ctrl Pts',(76.6518948370455,-8.57534623500454,
55.7514667654166));
#166993=CARTESIAN_POINT('Ctrl Pts',(76.5789499483404,-8.61020521221352,
55.7634738740725));
#166994=CARTESIAN_POINT('Ctrl Pts',(76.462946602241,-8.66379618776121,55.7825473341175));
#166995=CARTESIAN_POINT('Ctrl Pts',(76.4201793148645,-8.68316238197663,
55.7895746934616));
#166996=CARTESIAN_POINT('Ctrl Pts',(76.3394281967744,-8.71899471413204,
55.8028346722387));
#166997=CARTESIAN_POINT('Ctrl Pts',(76.3014768602568,-8.73553283198892,
55.8090629855396));
#166998=CARTESIAN_POINT('Ctrl Pts',(76.2155907037222,-8.77227929189866,
55.8231497824531));
#166999=CARTESIAN_POINT('Ctrl Pts',(76.1675952810867,-8.79233943306002,
55.8310160914402));
#167000=CARTESIAN_POINT('Ctrl Pts',(76.02490270769,-8.8505774199943,55.854385813728));
#167001=CARTESIAN_POINT('Ctrl Pts',(75.9297504065972,-8.88759574306452,
55.869947210255));
#167002=CARTESIAN_POINT('Ctrl Pts',(75.2751386841816,-9.12992603753234,
55.9768557513435));
#167003=CARTESIAN_POINT('Ctrl Pts',(74.6979562336475,-9.28244475646385,
56.0702707738278));
#167004=CARTESIAN_POINT('Ctrl Pts',(73.8233210946542,-9.4254961473837,56.2120285197604));
#167005=CARTESIAN_POINT('Ctrl Pts',(73.5341957873921,-9.45890297150018,
56.2589428223652));
#167006=CARTESIAN_POINT('Ctrl Pts',(73.1003189769933,-9.48842642732312,
56.3297599332903));
#167007=CARTESIAN_POINT('Ctrl Pts',(72.9563918679109,-9.49484976773475,
56.3533205160106));
#167008=CARTESIAN_POINT('Ctrl Pts',(72.7736558009451,-9.4987340790332,56.3833624766229));
#167009=CARTESIAN_POINT('Ctrl Pts',(72.734915541674,-9.49931412589773,56.3897387432393));
#167010=CARTESIAN_POINT('Ctrl Pts',(72.6726251672411,-9.4998554131959,56.4000039901323));
#167011=CARTESIAN_POINT('Ctrl Pts',(72.6490759894993,-9.49997011608609,
56.403887772357));
#167012=CARTESIAN_POINT('Ctrl Pts',(72.6037574946716,-9.50001778090229,
56.4113677781855));
#167013=CARTESIAN_POINT('Ctrl Pts',(72.5819883838354,-9.49996381921214,
56.4149635429323));
#167014=CARTESIAN_POINT('Ctrl Pts',(72.5338032426151,-9.49967424663347,
56.4229283235579));
#167015=CARTESIAN_POINT('Ctrl Pts',(72.5073877565322,-9.49940230610399,
56.4272984565549));
#167016=CARTESIAN_POINT('Ctrl Pts',(72.413289332745,-9.49803030629334,56.4428785749982));
#167017=CARTESIAN_POINT('Ctrl Pts',(72.3456206272278,-9.49630026944509,
56.4541059407717));
#167018=CARTESIAN_POINT('Ctrl Pts',(71.9000070444091,-9.48000900730683,
56.5281692111283));
#167019=CARTESIAN_POINT('Ctrl Pts',(71.5233031776256,-9.44300977489737,
56.5913762090154));
#167020=CARTESIAN_POINT('Ctrl Pts',(70.8271386592143,-9.33120543279843,
56.7082311688947));
#167021=CARTESIAN_POINT('Ctrl Pts',(70.5073361164754,-9.26229985036379,
56.761930867608));
#167022=CARTESIAN_POINT('Ctrl Pts',(69.9851626071795,-9.12051769081183,
56.8492191837797));
#167023=CARTESIAN_POINT('Ctrl Pts',(69.7805646262415,-9.05728830369756,
56.8833198619124));
#167024=CARTESIAN_POINT('Ctrl Pts',(69.4399526992648,-8.93898259000179,
56.9398470826378));
#167025=CARTESIAN_POINT('Ctrl Pts',(69.3027668991533,-8.88767220263716,
56.9625463825968));
#167026=CARTESIAN_POINT('Ctrl Pts',(69.1120095988285,-8.81114691545972,
56.9940040100372));
#167027=CARTESIAN_POINT('Ctrl Pts',(69.0574139907513,-8.78864005280026,
57.002995023854));
#167028=CARTESIAN_POINT('Ctrl Pts',(68.9639764294593,-8.74907747383411,
57.018361092331));
#167029=CARTESIAN_POINT('Ctrl Pts',(68.9250333609312,-8.73227418806761,
57.0247588878946));
#167030=CARTESIAN_POINT('Ctrl Pts',(68.850754637804,-8.69962119620557,57.0369492954803));
#167031=CARTESIAN_POINT('Ctrl Pts',(68.8154009484433,-8.68381623454716,
57.0427459629008));
#167032=CARTESIAN_POINT('Ctrl Pts',(68.732538644546,-8.64615160363277,57.0563193431114));
#167033=CARTESIAN_POINT('Ctrl Pts',(68.6851109532613,-8.62411069625395,
57.0640782656713));
#167034=CARTESIAN_POINT('Ctrl Pts',(68.5197760727363,-8.54557896337993,
57.0910912088325));
#167035=CARTESIAN_POINT('Ctrl Pts',(68.4028442360229,-8.48699813083125,
57.1101329793298));
#167036=CARTESIAN_POINT('Ctrl Pts',(67.7510073327286,-8.14314164054218,
57.2159440328911));
#167037=CARTESIAN_POINT('Ctrl Pts',(67.2428799584556,-7.80847175235973,
57.2970120852495));
#167038=CARTESIAN_POINT('Ctrl Pts',(66.627189069515,-7.31124077189001,57.3949564037384));
#167039=CARTESIAN_POINT('Ctrl Pts',(66.4876501584309,-7.19163359982041,
57.417142723216));
#167040=CARTESIAN_POINT('Ctrl Pts',(66.2971008723498,-7.01836649131229,
57.4475051916297));
#167041=CARTESIAN_POINT('Ctrl Pts',(66.2431203892434,-6.96811075817676,
57.4561143787328));
#167042=CARTESIAN_POINT('Ctrl Pts',(66.1492286410241,-6.87861501678154,
57.4711101711093));
#167043=CARTESIAN_POINT('Ctrl Pts',(66.1090689851143,-6.83964663452938,
57.4775312587777));
#167044=CARTESIAN_POINT('Ctrl Pts',(66.0489531754694,-6.78026439983104,
57.4871567023407));
#167045=CARTESIAN_POINT('Ctrl Pts',(66.0287412636062,-6.76011679026062,
57.4903952938556));
#167046=CARTESIAN_POINT('Ctrl Pts',(65.992116320494,-6.72327490259632,57.4962685598051));
#167047=CARTESIAN_POINT('Ctrl Pts',(65.9756738512513,-6.70661122162914,
57.4989071317947));
#167048=CARTESIAN_POINT('Ctrl Pts',(65.9384543237514,-6.66860858741753,
57.5048839392775));
#167049=CARTESIAN_POINT('Ctrl Pts',(65.9177157499812,-6.64723180845958,
57.5082170554009));
#167050=CARTESIAN_POINT('Ctrl Pts',(65.8539141451404,-6.58083989389841,
57.5184792056073));
#167051=CARTESIAN_POINT('Ctrl Pts',(65.8111922500503,-6.53549217524235,
57.525362048434));
#167052=CARTESIAN_POINT('Ctrl Pts',(65.4496562707306,-6.1440376390254,57.5836814772186));
#167053=CARTESIAN_POINT('Ctrl Pts',(65.1564237324558,-5.77466682140244,
57.6314437786339));
#167054=CARTESIAN_POINT('Ctrl Pts',(64.6271696504826,-4.99559301651045,
57.7166203379356));
#167055=CARTESIAN_POINT('Ctrl Pts',(64.3917609229367,-4.58707441697464,
57.7539296414042));
#167056=CARTESIAN_POINT('Ctrl Pts',(64.1517249399031,-4.08906171839117,
57.7905775941932));
#167057=CARTESIAN_POINT('Ctrl Pts',(64.1172450994925,-4.01513169422822,
57.7958021848038));
#167058=CARTESIAN_POINT('Ctrl Pts',(64.0642271782468,-3.89756843503945,
57.8037694993107));
#167059=CARTESIAN_POINT('Ctrl Pts',(64.0450664606938,-3.85422880773364,
57.8066343636464));
#167060=CARTESIAN_POINT('Ctrl Pts',(64.0096103182798,-3.77240039580295,
57.8119076001293));
#167061=CARTESIAN_POINT('Ctrl Pts',(63.9932442203614,-3.73394437312935,
57.8143298579128));
#167062=CARTESIAN_POINT('Ctrl Pts',(63.9568763421477,-3.64692001379552,
57.8196852868362));
#167063=CARTESIAN_POINT('Ctrl Pts',(63.9370199792312,-3.59829065424796,
57.822589957312));
#167064=CARTESIAN_POINT('Ctrl Pts',(63.8793667194219,-3.4537245527429,57.830965167705));
#167065=CARTESIAN_POINT('Ctrl Pts',(63.8427075241937,-3.35732966191139,
57.8362128357817));
#167066=CARTESIAN_POINT('Ctrl Pts',(63.6025406495692,-2.69394374354582,
57.8700416488785));
#167067=CARTESIAN_POINT('Ctrl Pts',(63.4508759665109,-2.10912859135389,
57.8884235627262));
#167068=CARTESIAN_POINT('Ctrl Pts',(63.3078994743928,-1.22309465822339,
57.9011693501972));
#167069=CARTESIAN_POINT('Ctrl Pts',(63.2743271865317,-0.930330914578197,
57.9030245152615));
#167070=CARTESIAN_POINT('Ctrl Pts',(63.2442955246402,-0.490899180369177,
57.902634895665));
#167071=CARTESIAN_POINT('Ctrl Pts',(63.2376615307871,-0.345101527986707,
57.9019874536953));
#167072=CARTESIAN_POINT('Ctrl Pts',(63.2334647197337,-0.159962073948043,
57.9005485740808));
#167073=CARTESIAN_POINT('Ctrl Pts',(63.2328158312106,-0.120706127649299,
57.9002083406172));
#167074=CARTESIAN_POINT('Ctrl Pts',(63.2321600363581,-0.0575831912739143,
57.8996057915336));
#167075=CARTESIAN_POINT('Ctrl Pts',(63.2320011701347,-0.0337180265013591,
57.8993652388043));
#167076=CARTESIAN_POINT('Ctrl Pts',(63.2318668976233,0.0122105293043752,
57.8988780519747));
#167077=CARTESIAN_POINT('Ctrl Pts',(63.2318785485024,0.034273637622909,
57.8986332777915));
#167078=CARTESIAN_POINT('Ctrl Pts',(63.2320728638578,0.0831114681549032,
57.8980674381057));
#167079=CARTESIAN_POINT('Ctrl Pts',(63.2322915224963,0.109885848235369,
57.8977412392575));
#167080=CARTESIAN_POINT('Ctrl Pts',(63.2334698568543,0.20527008881406,57.8965213928946));
#167081=CARTESIAN_POINT('Ctrl Pts',(63.2350535136951,0.273868947417529,
57.8955376158625));
#167082=CARTESIAN_POINT('Ctrl Pts',(63.2506255019945,0.73438064848014,57.8881935330277));
#167083=CARTESIAN_POINT('Ctrl Pts',(63.2878766102646,1.1250722932481,57.8783489777953));
#167084=CARTESIAN_POINT('Ctrl Pts',(63.4035972359396,1.86043661932604,57.8518033047862));
#167085=CARTESIAN_POINT('Ctrl Pts',(63.4774422076243,2.20520464142053,57.8359139645466));
#167086=CARTESIAN_POINT('Ctrl Pts',(63.6487563344907,2.83442980456629,57.7999334307641));
#167087=CARTESIAN_POINT('Ctrl Pts',(63.7410106299812,3.11990054383761,57.7808353102243));
#167088=CARTESIAN_POINT('Ctrl Pts',(63.8729625574057,3.47118158272536,57.7536996086356));
#167089=CARTESIAN_POINT('Ctrl Pts',(63.9003698276564,3.54160828277167,57.7480718247532));
#167090=CARTESIAN_POINT('Ctrl Pts',(63.9458134971997,3.6544228307231,57.7387527695002));
#167091=CARTESIAN_POINT('Ctrl Pts',(63.9633316139623,3.69702419853088,57.735163125661));
#167092=CARTESIAN_POINT('Ctrl Pts',(63.9973999085118,3.77820603078778,57.7281872559331));
#167093=CARTESIAN_POINT('Ctrl Pts',(64.0138982566356,3.81680792879478,57.7248112019246));
#167094=CARTESIAN_POINT('Ctrl Pts',(64.0521022480339,3.90459577177927,57.7169983783234));
#167095=CARTESIAN_POINT('Ctrl Pts',(64.0739682143242,3.95370754775727,57.7125301615332));
#167096=CARTESIAN_POINT('Ctrl Pts',(64.1333214779202,4.08405404421362,57.7004107319849));
#167097=CARTESIAN_POINT('Ctrl Pts',(64.171530506634,4.16494085057172,57.6926180815396));
#167098=CARTESIAN_POINT('Ctrl Pts',(64.4439995487114,4.72140993393359,57.6371173764298));
#167099=CARTESIAN_POINT('Ctrl Pts',(64.7159929997526,5.17671899593926,57.5819826842037));
#167100=CARTESIAN_POINT('Ctrl Pts',(65.2556278933211,5.92930167012332,57.4742239557703));
#167101=CARTESIAN_POINT('Ctrl Pts',(65.5070327918403,6.23699089422994,57.4245068846877));
#167102=CARTESIAN_POINT('Ctrl Pts',(65.8119182029589,6.56533159150481,57.3653750393213));
#167103=CARTESIAN_POINT('Ctrl Pts',(65.8472491391151,6.60275821621563,57.3585390883402));
#167104=CARTESIAN_POINT('Ctrl Pts',(65.9019726380357,6.65977974048592,57.3479782729481));
#167105=CARTESIAN_POINT('Ctrl Pts',(65.9211492056122,6.67958594173356,57.3442825375604));
#167106=CARTESIAN_POINT('Ctrl Pts',(65.9567826278662,6.71606578115462,57.3374249569922));
#167107=CARTESIAN_POINT('Ctrl Pts',(65.9732153167856,6.73276302986632,57.3342663509451));
#167108=CARTESIAN_POINT('Ctrl Pts',(66.011080373346,6.77095008647839,57.326996737532));
#167109=CARTESIAN_POINT('Ctrl Pts',(66.0325543152087,6.79239712079718,57.3228802417796));
#167110=CARTESIAN_POINT('Ctrl Pts',(66.1020262578688,6.8611108271439,57.3095815367732));
#167111=CARTESIAN_POINT('Ctrl Pts',(66.150424902648,6.9079589477878,57.3003455415892));
#167112=CARTESIAN_POINT('Ctrl Pts',(66.4452173369067,7.18721109030737,57.2442395016016));
#167113=CARTESIAN_POINT('Ctrl Pts',(66.7033999828718,7.40646837788407,57.1957148178854));
#167114=CARTESIAN_POINT('Ctrl Pts',(67.2016338024688,7.78507859305503,57.1024065185077));
#167115=CARTESIAN_POINT('Ctrl Pts',(67.4383506516803,7.94828523885839,57.058200187442));
#167116=CARTESIAN_POINT('Ctrl Pts',(67.8578043862365,8.2097551421779,56.9797654797525));
#167117=CARTESIAN_POINT('Ctrl Pts',(68.0370799036966,8.31336798873816,56.9462134805954));
#167118=CARTESIAN_POINT('Ctrl Pts',(68.34382173419,8.47724345363654,56.8886837590713));
#167119=CARTESIAN_POINT('Ctrl Pts',(68.4695267102784,8.54076784640929,56.8650750377454));
#167120=CARTESIAN_POINT('Ctrl Pts',(68.6489142397303,8.62635149445977,56.8313268052075));
#167121=CARTESIAN_POINT('Ctrl Pts',(68.7014701125895,8.65082272351403,56.8214326882021));
#167122=CARTESIAN_POINT('Ctrl Pts',(68.7925863317653,8.6922127478716,56.8042669976011));
#167123=CARTESIAN_POINT('Ctrl Pts',(68.8310423998376,8.70936626929446,56.7970184058439));
#167124=CARTESIAN_POINT('Ctrl Pts',(68.9099195534317,8.74390681295809,56.7821430558813));
#167125=CARTESIAN_POINT('Ctrl Pts',(68.9503499619508,8.76126896602064,56.7745141888425));
#167126=CARTESIAN_POINT('Ctrl Pts',(69.0531609805942,8.80455375859027,56.7551040152788));
#167127=CARTESIAN_POINT('Ctrl Pts',(69.1156987885475,8.83008036249795,56.7432873442472));
#167128=CARTESIAN_POINT('Ctrl Pts',(69.3601118387648,8.92673466386954,56.6970666396792));
#167129=CARTESIAN_POINT('Ctrl Pts',(69.5438719540856,8.99274928089602,56.6622327958355));
#167130=CARTESIAN_POINT('Ctrl Pts',(70.3045394493982,9.2390655768595,56.5177500921458));
#167131=CARTESIAN_POINT('Ctrl Pts',(70.8958147621585,9.36807306839831,56.4046620349361));
#167132=CARTESIAN_POINT('Ctrl Pts',(71.74764648053,9.46755482196796,56.2425827325765));
#167133=CARTESIAN_POINT('Ctrl Pts',(72.0011474928261,9.48653008343553,56.1944705996034));
#167134=CARTESIAN_POINT('Ctrl Pts',(72.3152302628538,9.49694909810163,56.135220467501));
#167135=CARTESIAN_POINT('Ctrl Pts',(72.3753375021582,9.4983517229637,56.1238979358385));
#167136=CARTESIAN_POINT('Ctrl Pts',(72.4633491342091,9.49954014093796,56.1073466339065));
#167137=CARTESIAN_POINT('Ctrl Pts',(72.4912432732057,9.49978958845323,56.1021049788767));
#167138=CARTESIAN_POINT('Ctrl Pts',(72.5405744468258,9.50000580127886,56.0928426752753));
#167139=CARTESIAN_POINT('Ctrl Pts',(72.5620106458844,9.50002465184133,56.0888204365761));
#167140=CARTESIAN_POINT('Ctrl Pts',(72.6086618487185,9.49990223857548,56.0800725951929));
#167141=CARTESIAN_POINT('Ctrl Pts',(72.6338765846449,9.49973217327249,56.0753479949009));
#167142=CARTESIAN_POINT('Ctrl Pts',(72.7044697574858,9.49896514963176,56.0621300369897));
#167143=CARTESIAN_POINT('Ctrl Pts',(72.7498464041002,9.49813557200794,56.053644536735));
#167144=CARTESIAN_POINT('Ctrl Pts',(73.0241877041815,9.49108494941575,56.0024010596379));
#167145=CARTESIAN_POINT('Ctrl Pts',(73.2529123496641,9.47663356441566,55.9599242027111));
#167146=CARTESIAN_POINT('Ctrl Pts',(73.9402989595516,9.40732134851028,55.832590466458));
#167147=CARTESIAN_POINT('Ctrl Pts',(74.3957579626969,9.3264294074589,55.7486248470616));
#167148=CARTESIAN_POINT('Ctrl Pts',(75.1665981452764,9.12874394520049,55.6057674057952));
#167149=CARTESIAN_POINT('Ctrl Pts',(75.4851651473643,9.02832480097397,55.5465053931756));
#167150=CARTESIAN_POINT('Ctrl Pts',(75.8873724343318,8.87708751583461,55.4711899113413));
#167151=CARTESIAN_POINT('Ctrl Pts',(75.9765188550052,8.84197274638609,55.4544654633048));
#167152=CARTESIAN_POINT('Ctrl Pts',(76.1113215854849,8.786434198187,55.4291254149382));
#167153=CARTESIAN_POINT('Ctrl Pts',(76.1573771759172,8.76702045639009,55.4204589323687));
#167154=CARTESIAN_POINT('Ctrl Pts',(76.2373811344034,8.73252895638724,55.4053882997191));
#167155=CARTESIAN_POINT('Ctrl Pts',(76.2713989404665,8.71761916185326,55.3989751798774));
#167156=CARTESIAN_POINT('Ctrl Pts',(76.3479817100524,8.68350134869854,55.3845261158146));
#167157=CARTESIAN_POINT('Ctrl Pts',(76.3904939261038,8.66417448904742,55.376497158438));
#167158=CARTESIAN_POINT('Ctrl Pts',(76.5055759959553,8.61079975804508,55.3547405493048));
#167159=CARTESIAN_POINT('Ctrl Pts',(76.577858328374,8.57612603714894,55.3410514585676));
#167160=CARTESIAN_POINT('Ctrl Pts',(77.0276679219405,8.35311292487585,55.2557174501453));
#167161=CARTESIAN_POINT('Ctrl Pts',(77.3926498052564,8.13994013275484,55.1857907711019));
#167162=CARTESIAN_POINT('Ctrl Pts',(77.9958719373521,7.73009805731332,55.0695013677019));
#167163=CARTESIAN_POINT('Ctrl Pts',(78.241058279384,7.54518352910079,55.0220138420851));
#167164=CARTESIAN_POINT('Ctrl Pts',(78.5968687876305,7.24827253993063,54.9530965697791));
#167165=CARTESIAN_POINT('Ctrl Pts',(78.7143576984184,7.14514031137337,54.9303407323003));
#167166=CARTESIAN_POINT('Ctrl Pts',(78.8780104389563,6.99408919902902,54.8986981688875));
#167167=CARTESIAN_POINT('Ctrl Pts',(78.9262795293674,6.94858191938103,54.8893723477172));
#167168=CARTESIAN_POINT('Ctrl Pts',(79.0111912884188,6.86681629702483,54.8729852347786));
#167169=CARTESIAN_POINT('Ctrl Pts',(79.0480209787864,6.83076416673249,54.8658837355163));
#167170=CARTESIAN_POINT('Ctrl Pts',(79.1041102809689,6.77495120781602,54.8550805941682));
#167171=CARTESIAN_POINT('Ctrl Pts',(79.1235774834283,6.75540924839076,54.8513333481908));
#167172=CARTESIAN_POINT('Ctrl Pts',(79.1594185899139,6.71911363903007,54.8444389105302));
#167173=CARTESIAN_POINT('Ctrl Pts',(79.1758157178529,6.70238450321822,54.8412865952095));
#167174=CARTESIAN_POINT('Ctrl Pts',(79.2132983974725,6.66385710712737,54.8340847475431));
#167175=CARTESIAN_POINT('Ctrl Pts',(79.2343423323037,6.64201714651654,54.8300443870573));
#167176=CARTESIAN_POINT('Ctrl Pts',(79.3016950774692,6.57143937040763,54.8171214459381));
#167177=CARTESIAN_POINT('Ctrl Pts',(79.3475969891558,6.52230001069604,54.8083273756248));
#167178=CARTESIAN_POINT('Ctrl Pts',(79.6180169411257,6.22654030109073,54.7565768455703));
#167179=CARTESIAN_POINT('Ctrl Pts',(79.8301018884544,5.96842381631564,54.7162228487968));
#167180=CARTESIAN_POINT('Ctrl Pts',(80.1960204684428,5.47168412008226,54.6463427308519));
#167181=CARTESIAN_POINT('Ctrl Pts',(80.353612814115,5.23640337575937,54.6161414988451));
#167182=CARTESIAN_POINT('Ctrl Pts',(80.612529467151,4.80972965763513,54.5660210859414));
#167183=CARTESIAN_POINT('Ctrl Pts',(80.7182460677757,4.62133224023602,54.5453806556852));
#167184=CARTESIAN_POINT('Ctrl Pts',(80.8844059838189,4.30003791327498,54.5125430232452));
#167185=CARTESIAN_POINT('Ctrl Pts',(80.9483537764292,4.16910516569654,54.4997911991359));
#167186=CARTESIAN_POINT('Ctrl Pts',(81.0340152048785,3.98300124835467,54.4825289181419));
#167187=CARTESIAN_POINT('Ctrl Pts',(81.0582434454874,3.92904737559927,54.4776243691093));
#167188=CARTESIAN_POINT('Ctrl Pts',(81.0990908996805,3.83577049978816,54.4693160546135));
#167189=CARTESIAN_POINT('Ctrl Pts',(81.1159498771867,3.79655782666367,54.4658747610282));
#167190=CARTESIAN_POINT('Ctrl Pts',(81.1477507323136,3.72120116370777,54.4593595772727));
#167191=CARTESIAN_POINT('Ctrl Pts',(81.162734497092,3.68507637194616,54.4562791438284));
#167192=CARTESIAN_POINT('Ctrl Pts',(81.2013504639087,3.59033391878792,54.4483119284538));
#167193=CARTESIAN_POINT('Ctrl Pts',(81.2246247789901,3.531567824447,54.4434812469245));
#167194=CARTESIAN_POINT('Ctrl Pts',(81.3048195903584,3.32305529302083,54.4267322493362));
#167195=CARTESIAN_POINT('Ctrl Pts',(81.3585664734141,3.1720780440009,54.4153122128391));
#167196=CARTESIAN_POINT('Ctrl Pts',(81.6153604679569,2.38895760027483,54.3597019091175));
#167197=CARTESIAN_POINT('Ctrl Pts',(81.7561565625459,1.73766512540865,54.3252901811299));
#167198=CARTESIAN_POINT('Ctrl Pts',(81.8569271514174,0.821510333654386,
54.2949775075885));
#167199=CARTESIAN_POINT('Ctrl Pts',(81.8748098085163,0.565284361092315,
54.288437205712));
#167200=CARTESIAN_POINT('Ctrl Pts',(81.8843188155679,0.247674584612399,
54.2829165930799));
#167201=CARTESIAN_POINT('Ctrl Pts',(81.8855682365754,0.186718236933947,
54.2819748184765));
#167202=CARTESIAN_POINT('Ctrl Pts',(81.8865564700108,0.0974115784321152,
54.2807709734858));
#167203=CARTESIAN_POINT('Ctrl Pts',(81.8867458609506,0.0690690495417933,
54.2804148714424));
#167204=CARTESIAN_POINT('Ctrl Pts',(81.8868423009076,0.0271505916043363,
54.279926941574));
#167205=CARTESIAN_POINT('Ctrl Pts',(81.8868450451571,0.0135753215422557,
54.2797749350526));
#167206=CARTESIAN_POINT('Ctrl Pts',(81.8868193065938,6.72938151241379E-11,
54.2796289644064));
#167207=CARTESIAN_POINT('Origin',(73.0915550886457,-4.33680868994202E-16,
59.1075264962884));
#167208=CARTESIAN_POINT('',(81.7660537076114,-5.44047451804188E-12,53.5947332184626));
#167209=CARTESIAN_POINT('',(81.7739479911102,2.25145191314116E-12,53.6395039249478));
#167210=CARTESIAN_POINT('',(82.4472287422617,-1.59709532818419E-15,57.4578688084528));
#167211=CARTESIAN_POINT('Ctrl Pts',(81.7660537076114,-1.08793519407556E-11,
53.5947332184626));
#167212=CARTESIAN_POINT('Ctrl Pts',(81.766089311675,0.0187786941596928,
53.594935139141));
#167213=CARTESIAN_POINT('Ctrl Pts',(81.7660697497931,0.0375572995376573,
53.5951448454953));
#167214=CARTESIAN_POINT('Ctrl Pts',(81.7658885063145,0.0831106075212402,
53.5956726299015));
#167215=CARTESIAN_POINT('Ctrl Pts',(81.7656698513442,0.109884855239771,
53.5959988267661));
#167216=CARTESIAN_POINT('Ctrl Pts',(81.7644915402974,0.205268114732128,
53.5972186589636));
#167217=CARTESIAN_POINT('Ctrl Pts',(81.7629079201996,0.273866125009716,
53.5982024213271));
#167218=CARTESIAN_POINT('Ctrl Pts',(81.747329218689,0.734581573566942,53.6055497270411));
#167219=CARTESIAN_POINT('Ctrl Pts',(81.7100462908909,1.12547632460795,53.6154012865544));
#167220=CARTESIAN_POINT('Ctrl Pts',(81.594204699406,1.8613059481231,53.6419721180145));
#167221=CARTESIAN_POINT('Ctrl Pts',(81.5202657075538,2.20633441514307,53.6578804072962));
#167222=CARTESIAN_POINT('Ctrl Pts',(81.3488968214419,2.83539203505383,53.6938704724558));
#167223=CARTESIAN_POINT('Ctrl Pts',(81.2567482905691,3.12045454484827,53.7129464508605));
#167224=CARTESIAN_POINT('Ctrl Pts',(81.1249480906405,3.47131279343958,53.7400508866665));
#167225=CARTESIAN_POINT('Ctrl Pts',(81.0975505357671,3.54171179529186,53.7456766669679));
#167226=CARTESIAN_POINT('Ctrl Pts',(81.0521192256183,3.65449288038163,53.7549931790221));
#167227=CARTESIAN_POINT('Ctrl Pts',(81.0346031953589,3.69708825898491,53.7585823925088));
#167228=CARTESIAN_POINT('Ctrl Pts',(81.0005361595372,3.77826559731044,53.7655579999387));
#167229=CARTESIAN_POINT('Ctrl Pts',(80.9840368793863,3.81686894571487,53.7689342424537));
#167230=CARTESIAN_POINT('Ctrl Pts',(80.945826599136,3.90466953481744,53.7767483469641));
#167231=CARTESIAN_POINT('Ctrl Pts',(80.9239551055655,3.95379252712304,53.7812176895887));
#167232=CARTESIAN_POINT('Ctrl Pts',(80.8645769792569,4.08418981395652,53.7933421840864));
#167233=CARTESIAN_POINT('Ctrl Pts',(80.8263476963176,4.16511574105258,53.8011389535829));
#167234=CARTESIAN_POINT('Ctrl Pts',(80.5541150543673,4.7210670533362,53.856591386042));
#167235=CARTESIAN_POINT('Ctrl Pts',(80.2824691179467,5.17586792222044,53.9116556106604));
#167236=CARTESIAN_POINT('Ctrl Pts',(79.7430125147178,5.92846932190368,54.0193818686345));
#167237=CARTESIAN_POINT('Ctrl Pts',(79.4913043740192,6.23658400322117,54.0691602503405));
#167238=CARTESIAN_POINT('Ctrl Pts',(79.1860624510275,6.56531110064247,54.1283613052804));
#167239=CARTESIAN_POINT('Ctrl Pts',(79.1507268808955,6.60274283164926,54.1351981583995));
#167240=CARTESIAN_POINT('Ctrl Pts',(79.0959976968593,6.65977045457835,54.1457600759643));
#167241=CARTESIAN_POINT('Ctrl Pts',(79.0768201504957,6.67957771830201,54.1494560015092));
#167242=CARTESIAN_POINT('Ctrl Pts',(79.0411858971306,6.71605848665225,54.1563137443743));
#167243=CARTESIAN_POINT('Ctrl Pts',(79.0247533660064,6.73275561183066,54.1594723212229));
#167244=CARTESIAN_POINT('Ctrl Pts',(78.9868899350406,6.7709411156073,54.1667416251171));
#167245=CARTESIAN_POINT('Ctrl Pts',(78.9654174739252,6.7923867337347,54.1708578388394));
#167246=CARTESIAN_POINT('Ctrl Pts',(78.8959552506888,6.86109107270506,54.1841546902176));
#167247=CARTESIAN_POINT('Ctrl Pts',(78.8475650007641,6.90793140714231,54.1933890926434));
#167248=CARTESIAN_POINT('Ctrl Pts',(78.5532008394214,7.18678090178326,54.2494136969507));
#167249=CARTESIAN_POINT('Ctrl Pts',(78.295479288909,7.40569001903707,54.2978527190256));
#167250=CARTESIAN_POINT('Ctrl Pts',(77.7981254176937,7.78378075038857,54.3909973997704));
#167251=CARTESIAN_POINT('Ctrl Pts',(77.5618137061987,7.94679912788598,54.4351283213659));
#167252=CARTESIAN_POINT('Ctrl Pts',(77.142293647711,8.20850395491835,54.5135747900315));
#167253=CARTESIAN_POINT('Ctrl Pts',(76.9625059866902,8.31246863880373,54.5472221954063));
#167254=CARTESIAN_POINT('Ctrl Pts',(76.6549779415856,8.47681683120888,54.6048989047051));
#167255=CARTESIAN_POINT('Ctrl Pts',(76.5290125853886,8.54048629379684,54.6285563795084));
#167256=CARTESIAN_POINT('Ctrl Pts',(76.3493178397523,8.62622472709793,54.6623623166521));
#167257=CARTESIAN_POINT('Ctrl Pts',(76.2967206130346,8.65071711526014,54.6722641967464));
#167258=CARTESIAN_POINT('Ctrl Pts',(76.2055557048802,8.69213170326657,54.6894390311634));
#167259=CARTESIAN_POINT('Ctrl Pts',(76.1670926140245,8.70928932300813,54.6966889350736));
#167260=CARTESIAN_POINT('Ctrl Pts',(76.0930125481498,8.74173094133538,54.710659586924));
#167261=CARTESIAN_POINT('Ctrl Pts',(76.0574133770316,8.75705506989795,54.7173763969815));
#167262=CARTESIAN_POINT('Ctrl Pts',(75.9636750452429,8.79671001447499,54.7350713680082));
#167263=CARTESIAN_POINT('Ctrl Pts',(75.9053871234054,8.8206689587982,54.7460829509784));
#167264=CARTESIAN_POINT('Ctrl Pts',(75.6963697012725,8.90409779949654,54.7856005397252));
#167265=CARTESIAN_POINT('Ctrl Pts',(75.544374851785,8.9601798693336,54.8143943173984));
#167266=CARTESIAN_POINT('Ctrl Pts',(74.7764584901133,9.2207778185887,54.9601245350163));
#167267=CARTESIAN_POINT('Ctrl Pts',(74.1423871569636,9.36365084070184,55.0814246755504));
#167268=CARTESIAN_POINT('Ctrl Pts',(73.2475224556367,9.46777148786138,55.2516873773412));
#167269=CARTESIAN_POINT('Ctrl Pts',(72.9951276850991,9.4866018652505,55.2995880089901));
#167270=CARTESIAN_POINT('Ctrl Pts',(72.6822831747417,9.49696017760314,55.3586040050923));
#167271=CARTESIAN_POINT('Ctrl Pts',(72.6223026888742,9.49835732872119,55.3699025822977));
#167272=CARTESIAN_POINT('Ctrl Pts',(72.534441515006,9.49954185362375,55.3864255298651));
#167273=CARTESIAN_POINT('Ctrl Pts',(72.5065710197733,9.49979060707295,55.3916627259293));
#167274=CARTESIAN_POINT('Ctrl Pts',(72.4572655253772,9.5000060442374,55.4009201855465));
#167275=CARTESIAN_POINT('Ctrl Pts',(72.4358313603421,9.50002461188377,55.4049420326747));
#167276=CARTESIAN_POINT('Ctrl Pts',(72.3891655357367,9.49990156374198,55.413692595416));
#167277=CARTESIAN_POINT('Ctrl Pts',(72.3639341443655,9.49973099490788,55.4184203034165));
#167278=CARTESIAN_POINT('Ctrl Pts',(72.2932499537031,9.49896169398094,55.4316552619596));
#167279=CARTESIAN_POINT('Ctrl Pts',(72.2477989566889,9.49812937607001,55.4401546226488));
#167280=CARTESIAN_POINT('Ctrl Pts',(71.9715978664719,9.49101920390794,55.4917451456631));
#167281=CARTESIAN_POINT('Ctrl Pts',(71.7410925927617,9.47637800073317,55.5345505785301));
#167282=CARTESIAN_POINT('Ctrl Pts',(71.0528728697567,9.40654687555473,55.662033176143));
#167283=CARTESIAN_POINT('Ctrl Pts',(70.5983499454807,9.32559737393371,55.7458276171454));
#167284=CARTESIAN_POINT('Ctrl Pts',(69.8292493820901,9.12808823030405,55.8883657059645));
#167285=CARTESIAN_POINT('Ctrl Pts',(69.5114867796251,9.02785437859029,55.947479454498));
#167286=CARTESIAN_POINT('Ctrl Pts',(69.1101656723436,8.87692203359165,56.0226295482308));
#167287=CARTESIAN_POINT('Ctrl Pts',(69.0211279174825,8.84184564459701,56.0393337001265));
#167288=CARTESIAN_POINT('Ctrl Pts',(68.8864545401026,8.78635656545091,56.0646495113161));
#167289=CARTESIAN_POINT('Ctrl Pts',(68.8404207899903,8.76695091906606,56.0733119070883));
#167290=CARTESIAN_POINT('Ctrl Pts',(68.7604407912212,8.73246816398617,56.0883780592396));
#167291=CARTESIAN_POINT('Ctrl Pts',(68.7264252370218,8.71755869347868,56.0947907683467));
#167292=CARTESIAN_POINT('Ctrl Pts',(68.6498294865343,8.68343362942294,56.1092423120975));
#167293=CARTESIAN_POINT('Ctrl Pts',(68.6073021534936,8.66409893527404,56.1172741445388));
#167294=CARTESIAN_POINT('Ctrl Pts',(68.4921337091477,8.61068113494746,56.1390471454897));
#167295=CARTESIAN_POINT('Ctrl Pts',(68.4197808882597,8.57597054021846,56.1527496490367));
#167296=CARTESIAN_POINT('Ctrl Pts',(67.9651233300583,8.35052706178557,56.2390039158279));
#167297=CARTESIAN_POINT('Ctrl Pts',(67.5957012389091,8.13430902447392,56.3097916254067));
#167298=CARTESIAN_POINT('Ctrl Pts',(66.9786628403738,7.71348127405852,56.4287629763096));
#167299=CARTESIAN_POINT('Ctrl Pts',(66.7243901780782,7.52022027008374,56.4780250396689));
#167300=CARTESIAN_POINT('Ctrl Pts',(66.3694688561866,7.22061335610846,56.5467679879914));
#167301=CARTESIAN_POINT('Ctrl Pts',(66.2608036355152,7.12447830648815,56.567810682016));
#167302=CARTESIAN_POINT('Ctrl Pts',(66.0867033385695,6.96311362972743,56.6014682042626));
#167303=CARTESIAN_POINT('Ctrl Pts',(66.0199535653995,6.8993958990753,56.6143581285272));
#167304=CARTESIAN_POINT('Ctrl Pts',(65.9293917436607,6.81036862447813,56.6318147587271));
#167305=CARTESIAN_POINT('Ctrl Pts',(65.9047843305848,6.78590964943391,56.6365547713395));
#167306=CARTESIAN_POINT('Ctrl Pts',(65.8633915620035,6.74431012431058,56.6445216818408));
#167307=CARTESIAN_POINT('Ctrl Pts',(65.8465370347348,6.72724175290705,56.6477638702909));
#167308=CARTESIAN_POINT('Ctrl Pts',(65.8117710044302,6.69176519442075,56.6544475018772));
#167309=CARTESIAN_POINT('Ctrl Pts',(65.7938690704714,6.67334768426026,56.6578868566572));
#167310=CARTESIAN_POINT('Ctrl Pts',(65.7463937169884,6.62410464340944,56.6670025242646));
#167311=CARTESIAN_POINT('Ctrl Pts',(65.7169512498564,6.59314839645086,56.6726501054801));
#167312=CARTESIAN_POINT('Ctrl Pts',(65.584423839207,6.45190047504579,56.6980497602557));
#167313=CARTESIAN_POINT('Ctrl Pts',(65.4837354091013,6.33929904271823,56.7172881251141));
#167314=CARTESIAN_POINT('Ctrl Pts',(65.0730914342873,5.85730632321677,56.7956588974026));
#167315=CARTESIAN_POINT('Ctrl Pts',(64.7885145284515,5.46645740968215,56.8497818266967));
#167316=CARTESIAN_POINT('Ctrl Pts',(64.4136755499147,4.85909413547504,56.9222177560214));
#167317=CARTESIAN_POINT('Ctrl Pts',(64.2997801843603,4.65857942921805,56.9444181941565));
#167318=CARTESIAN_POINT('Ctrl Pts',(64.1228253630042,4.31884181992413,56.9793513879912));
#167319=CARTESIAN_POINT('Ctrl Pts',(64.055650751179,4.18194362018412,56.9927359564357));
#167320=CARTESIAN_POINT('Ctrl Pts',(63.9665797219404,3.98882781585597,57.0106786875953));
#167321=CARTESIAN_POINT('Ctrl Pts',(63.9419006787588,3.93396074097829,57.0156729519043));
#167322=CARTESIAN_POINT('Ctrl Pts',(63.9005278980066,3.83960168641521,57.0240861126173));
#167323=CARTESIAN_POINT('Ctrl Pts',(63.8835793203608,3.80022707509067,57.0275448986472));
#167324=CARTESIAN_POINT('Ctrl Pts',(63.8517550363479,3.72489882762584,57.0340634388743));
#167325=CARTESIAN_POINT('Ctrl Pts',(63.8368329145727,3.68896638502454,57.0371304454779));
#167326=CARTESIAN_POINT('Ctrl Pts',(63.8024138836432,3.60463245713474,57.0442298263955));
#167327=CARTESIAN_POINT('Ctrl Pts',(63.7830925569564,3.55615838193804,57.0482346709695));
#167328=CARTESIAN_POINT('Ctrl Pts',(63.7176581611327,3.38799749356167,57.0618667765012));
#167329=CARTESIAN_POINT('Ctrl Pts',(63.6735517416903,3.26751974012838,57.0711790909016));
#167330=CARTESIAN_POINT('Ctrl Pts',(63.429555276041,2.55703805104296,57.1234470674421));
#167331=CARTESIAN_POINT('Ctrl Pts',(63.2851253917232,1.94897037145211,57.1577210353531));
#167332=CARTESIAN_POINT('Ctrl Pts',(63.1666622239508,1.08392075099097,57.1906794009407));
#167333=CARTESIAN_POINT('Ctrl Pts',(63.1424296648806,0.835760212641774,
57.1983452148013));
#167334=CARTESIAN_POINT('Ctrl Pts',(63.1200700971016,0.455255564289024,
57.2071683363034));
#167335=CARTESIAN_POINT('Ctrl Pts',(63.1150253214581,0.323459011811552,
57.2096890550143));
#167336=CARTESIAN_POINT('Ctrl Pts',(63.1119928394879,0.153636672107118,
57.2122182595312));
#167337=CARTESIAN_POINT('Ctrl Pts',(63.1115379645799,0.115676936922943,
57.21273737601));
#167338=CARTESIAN_POINT('Ctrl Pts',(63.1111617642863,0.054136416387556,
57.2135030922203));
#167339=CARTESIAN_POINT('Ctrl Pts',(63.1111035839216,0.0305572408797322,
57.2137784196053));
#167340=CARTESIAN_POINT('Ctrl Pts',(63.111157487027,-0.0152400383097263,
57.214277837288));
#167341=CARTESIAN_POINT('Ctrl Pts',(63.1112599297194,-0.0374578964485856,
57.214503944773));
#167342=CARTESIAN_POINT('Ctrl Pts',(63.1116591095197,-0.0870722029593554,
57.2149730047514));
#167343=CARTESIAN_POINT('Ctrl Pts',(63.1119955738653,-0.114468264310403,
57.2152075980197));
#167344=CARTESIAN_POINT('Ctrl Pts',(63.1135614728535,-0.209260586160049,
57.2159356541743));
#167345=CARTESIAN_POINT('Ctrl Pts',(63.115377369187,-0.27664605349559,57.2163068776385));
#167346=CARTESIAN_POINT('Ctrl Pts',(63.1321645750317,-0.725604601534028,
57.2178278532523));
#167347=CARTESIAN_POINT('Ctrl Pts',(63.1689751832739,-1.10602626318967,
57.214541776366));
#167348=CARTESIAN_POINT('Ctrl Pts',(63.2792496235438,-1.80799893656087,
57.2009627838911));
#167349=CARTESIAN_POINT('Ctrl Pts',(63.3468390394394,-2.12991371852061,
57.1917147605416));
#167350=CARTESIAN_POINT('Ctrl Pts',(63.4866173257163,-2.65909406999227,
57.1718431541107));
#167351=CARTESIAN_POINT('Ctrl Pts',(63.5496627790994,-2.8685318306424,57.1627182335516));
#167352=CARTESIAN_POINT('Ctrl Pts',(63.6676123373362,-3.21675006653548,
57.1454795911502));
#167353=CARTESIAN_POINT('Ctrl Pts',(63.7187068458715,-3.3567587597836,57.1379699564294));
#167354=CARTESIAN_POINT('Ctrl Pts',(63.7948446251956,-3.55117565991767,
57.1267346378981));
#167355=CARTESIAN_POINT('Ctrl Pts',(63.8171707819532,-3.60664853390628,
57.1234351441384));
#167356=CARTESIAN_POINT('Ctrl Pts',(63.8563852080932,-3.70150621018156,
57.1176319241774));
#167357=CARTESIAN_POINT('Ctrl Pts',(63.8730217131375,-3.74099549251064,
57.1151676336021));
#167358=CARTESIAN_POINT('Ctrl Pts',(63.9053281270779,-3.8162621156397,57.1103779572939));
#167359=CARTESIAN_POINT('Ctrl Pts',(63.9209531322106,-3.85205822088329,
57.10805960032));
#167360=CARTESIAN_POINT('Ctrl Pts',(63.9622185645461,-3.94503739716452,
57.1019321492266));
#167361=CARTESIAN_POINT('Ctrl Pts',(63.9882013443875,-4.0020628674108,57.0980694252641));
#167362=CARTESIAN_POINT('Ctrl Pts',(64.0813730043895,-4.20133348853111,
57.0842018467488));
#167363=CARTESIAN_POINT('Ctrl Pts',(64.1514990701253,-4.34214426541746,
57.073736295198));
#167364=CARTESIAN_POINT('Ctrl Pts',(64.5276242686246,-5.05284365776764,
57.0174305968665));
#167365=CARTESIAN_POINT('Ctrl Pts',(64.8872203712195,-5.59172393386763,
56.9631928403841));
#167366=CARTESIAN_POINT('Ctrl Pts',(65.3861799682201,-6.19628194310113,
56.8855119893723));
#167367=CARTESIAN_POINT('Ctrl Pts',(65.4767201862364,-6.30122230454004,
56.8713292366245));
#167368=CARTESIAN_POINT('Ctrl Pts',(65.6293416652474,-6.47049138706509,
56.8472395004043));
#167369=CARTESIAN_POINT('Ctrl Pts',(65.6901143975928,-6.53600984312842,
56.8376020928291));
#167370=CARTESIAN_POINT('Ctrl Pts',(65.7754878287027,-6.62548447115215,
56.8239915930124));
#167371=CARTESIAN_POINT('Ctrl Pts',(65.7993204352857,-6.65019225383117,
56.8201845630712));
#167372=CARTESIAN_POINT('Ctrl Pts',(65.8400185530687,-6.69192951249316,
56.8136699056959));
#167373=CARTESIAN_POINT('Ctrl Pts',(65.8568167251176,-6.70902655665234,
56.810977107473));
#167374=CARTESIAN_POINT('Ctrl Pts',(65.8919170522222,-6.7444817686687,56.8053421235555));
#167375=CARTESIAN_POINT('Ctrl Pts',(65.9102297572077,-6.76282865170696,
56.8023976128523));
#167376=CARTESIAN_POINT('Ctrl Pts',(65.9595498707783,-6.81183737592831,
56.7944556713425));
#167377=CARTESIAN_POINT('Ctrl Pts',(65.9906915295878,-6.84235840481285,
56.7894286498668));
#167378=CARTESIAN_POINT('Ctrl Pts',(66.1372954964266,-6.98407011312404,
56.7657105154106));
#167379=CARTESIAN_POINT('Ctrl Pts',(66.2553107171901,-7.09248843979961,
56.7464666034052));
#167380=CARTESIAN_POINT('Ctrl Pts',(66.6793857970444,-7.46262979858878,
56.6769599864269));
#167381=CARTESIAN_POINT('Ctrl Pts',(66.9991242809228,-7.70748361618338,
56.6239453297674));
#167382=CARTESIAN_POINT('Ctrl Pts',(67.6438958129781,-8.13844539967706,
56.5170596848018));
#167383=CARTESIAN_POINT('Ctrl Pts',(67.9663774915458,-8.32709835295906,
56.4636105473459));
#167384=CARTESIAN_POINT('Ctrl Pts',(68.3882118940512,-8.54100625152076,
56.3940461414255));
#167385=CARTESIAN_POINT('Ctrl Pts',(68.4780194289604,-8.58474515862727,
56.3792541317284));
#167386=CARTESIAN_POINT('Ctrl Pts',(68.6145962844914,-8.64856389684196,
56.3567896683141));
#167387=CARTESIAN_POINT('Ctrl Pts',(68.6608640935571,-8.66972315007258,
56.3491846781772));
#167388=CARTESIAN_POINT('Ctrl Pts',(68.7450108435647,-8.70737392981719,
56.3353634122024));
#167389=CARTESIAN_POINT('Ctrl Pts',(68.7828315981335,-8.7239950583187,56.3291548489606));
#167390=CARTESIAN_POINT('Ctrl Pts',(68.8646125220353,-8.75928728392246,
56.3157377244104));
#167391=CARTESIAN_POINT('Ctrl Pts',(68.9086077020988,-8.77787254010335,
56.3085246405678));
#167392=CARTESIAN_POINT('Ctrl Pts',(69.02884805874,-8.82757858244895,56.2888243443684));
#167393=CARTESIAN_POINT('Ctrl Pts',(69.1053617835307,-8.85802458593729,
56.2763027769185));
#167394=CARTESIAN_POINT('Ctrl Pts',(69.6280695734132,-9.05801385643573,
56.1908582245492));
#167395=CARTESIAN_POINT('Ctrl Pts',(70.0861417683028,-9.19389455685718,
56.1165060073459));
#167396=CARTESIAN_POINT('Ctrl Pts',(71.0323438312868,-9.39685184028539,
55.9631929772623));
#167397=CARTESIAN_POINT('Ctrl Pts',(71.519505702754,-9.46149162727628,55.8843905420308));
#167398=CARTESIAN_POINT('Ctrl Pts',(72.1119017796888,-9.49263414192549,
55.7874979223915));
#167399=CARTESIAN_POINT('Ctrl Pts',(72.2146127353695,-9.49631962096214,
55.7706580823399));
#167400=CARTESIAN_POINT('Ctrl Pts',(72.3529391211423,-9.49897699309798,
55.7479085197052));
#167401=CARTESIAN_POINT('Ctrl Pts',(72.3885266354459,-9.49945524949781,
55.7420494120179));
#167402=CARTESIAN_POINT('Ctrl Pts',(72.4447023201719,-9.49988596953694,
55.7327899514867));
#167403=CARTESIAN_POINT('Ctrl Pts',(72.4652898574265,-9.49997508678827,
55.7293942248832));
#167404=CARTESIAN_POINT('Ctrl Pts',(72.5079282331955,-9.50001729772026,
55.722356492773));
#167405=CARTESIAN_POINT('Ctrl Pts',(72.5299787883694,-9.49996026903604,
55.7187141574565));
#167406=CARTESIAN_POINT('Ctrl Pts',(72.5837046672675,-9.49962917292953,
55.7098332443231));
#167407=CARTESIAN_POINT('Ctrl Pts',(72.6153788156775,-9.49927122114843,
55.7045920701524));
#167408=CARTESIAN_POINT('Ctrl Pts',(72.7293895959455,-9.49739684630065,
55.6857084136771));
#167409=CARTESIAN_POINT('Ctrl Pts',(72.8117027750687,-9.49494330885159,
55.6720408700257));
#167410=CARTESIAN_POINT('Ctrl Pts',(73.333786850443,-9.47239647567461,55.5851795638939));
#167411=CARTESIAN_POINT('Ctrl Pts',(73.7716154456839,-9.42201164183068,
55.5115820349469));
#167412=CARTESIAN_POINT('Ctrl Pts',(74.7093058965669,-9.24561783447955,
55.354199663201));
#167413=CARTESIAN_POINT('Ctrl Pts',(75.2057357664216,-9.10869101437909,
55.2710584822521));
#167414=CARTESIAN_POINT('Ctrl Pts',(75.790445398465,-8.89384269090942,55.174243065176));
#167415=CARTESIAN_POINT('Ctrl Pts',(75.8915036496523,-8.85469288439399,
55.1575490123797));
#167416=CARTESIAN_POINT('Ctrl Pts',(76.0405337587023,-8.79394617656608,
55.1329921667997));
#167417=CARTESIAN_POINT('Ctrl Pts',(76.0890265413662,-8.77369980296775,
55.1250114572114));
#167418=CARTESIAN_POINT('Ctrl Pts',(76.1754596780747,-8.73675133555327,
55.110804562409));
#167419=CARTESIAN_POINT('Ctrl Pts',(76.2134628074514,-8.720205154257,55.1045642693147));
#167420=CARTESIAN_POINT('Ctrl Pts',(76.2939657059386,-8.68451466408779,
55.0913586319232));
#167421=CARTESIAN_POINT('Ctrl Pts',(76.3364357378043,-8.66530366954231,
55.0843998278683));
#167422=CARTESIAN_POINT('Ctrl Pts',(76.4507376762134,-8.612564761637,55.065692697827));
#167423=CARTESIAN_POINT('Ctrl Pts',(76.5222973009616,-8.57843498161289,
55.0540040559273));
#167424=CARTESIAN_POINT('Ctrl Pts',(76.9512176901878,-8.36711934902414,
54.9840809592697));
#167425=CARTESIAN_POINT('Ctrl Pts',(77.2976708617606,-8.16795873159066,
54.9282045165333));
#167426=CARTESIAN_POINT('Ctrl Pts',(77.9522518577298,-7.73382098625736,
54.8233966356192));
#167427=CARTESIAN_POINT('Ctrl Pts',(78.2606662805836,-7.50070914316503,
54.7743879784506));
#167428=CARTESIAN_POINT('Ctrl Pts',(78.6929658769925,-7.12999257225669,
54.7056076110398));
#167429=CARTESIAN_POINT('Ctrl Pts',(78.8284054257806,-7.00681721704554,
54.6840418389898));
#167430=CARTESIAN_POINT('Ctrl Pts',(78.9929135639126,-6.84819501800568,
54.6577482718694));
#167431=CARTESIAN_POINT('Ctrl Pts',(79.025393562022,-6.81642032567887,54.6525518781379));
#167432=CARTESIAN_POINT('Ctrl Pts',(79.0763263072911,-6.76586688962991,
54.6443935996856));
#167433=CARTESIAN_POINT('Ctrl Pts',(79.0949308817272,-6.74724537563443,
54.6414114951433));
#167434=CARTESIAN_POINT('Ctrl Pts',(79.1302104800646,-6.71163626877166,
54.6357522266302));
#167435=CARTESIAN_POINT('Ctrl Pts',(79.1468993974597,-6.69466324849478,
54.6330732100695));
#167436=CARTESIAN_POINT('Ctrl Pts',(79.1868167471057,-6.65375736669634,
54.6266610932853));
#167437=CARTESIAN_POINT('Ctrl Pts',(79.2099834345467,-6.62976338517252,
54.6229361964881));
#167438=CARTESIAN_POINT('Ctrl Pts',(79.2903049313384,-6.54568500892601,
54.6100107638819));
#167439=CARTESIAN_POINT('Ctrl Pts',(79.3468007618755,-6.48496263549507,
54.6009001541037));
#167440=CARTESIAN_POINT('Ctrl Pts',(79.7275711237563,-6.06473432874413,
54.5394083290304));
#167441=CARTESIAN_POINT('Ctrl Pts',(80.0248644545611,-5.68118573127458,
54.4909881299508));
#167442=CARTESIAN_POINT('Ctrl Pts',(80.5273632882508,-4.91925352939866,
54.4103218509623));
#167443=CARTESIAN_POINT('Ctrl Pts',(80.7387225627891,-4.54652323968196,
54.376931620969));
#167444=CARTESIAN_POINT('Ctrl Pts',(80.959850812974,-4.08747785067972,54.3431747723531));
#167445=CARTESIAN_POINT('Ctrl Pts',(80.9941542065315,-4.01389507305992,
54.33797744475));
#167446=CARTESIAN_POINT('Ctrl Pts',(81.0469660238515,-3.89675726489382,
54.3300416407751));
#167447=CARTESIAN_POINT('Ctrl Pts',(81.0660892781304,-3.85349208227253,
54.3271825545163));
#167448=CARTESIAN_POINT('Ctrl Pts',(81.099850286557,-3.77555981267128,54.3221617037155));
#167449=CARTESIAN_POINT('Ctrl Pts',(81.1146047699058,-3.74094587430185,
54.3199770211922));
#167450=CARTESIAN_POINT('Ctrl Pts',(81.1487385677232,-3.65954761405594,
54.3149457253764));
#167451=CARTESIAN_POINT('Ctrl Pts',(81.1679530919834,-3.6126934543398,54.3121314177833));
#167452=CARTESIAN_POINT('Ctrl Pts',(81.2229232410845,-3.47557751962789,
54.3041334370407));
#167453=CARTESIAN_POINT('Ctrl Pts',(81.2576882098913,-3.38491441259102,
54.2991438579255));
#167454=CARTESIAN_POINT('Ctrl Pts',(81.4074338600818,-2.97600506029438,
54.2779699511291));
#167455=CARTESIAN_POINT('Ctrl Pts',(81.5070221635251,-2.65223242719468,
54.2647958639422));
#167456=CARTESIAN_POINT('Ctrl Pts',(81.7035348461263,-1.86876789217715,
54.2410678371496));
#167457=CARTESIAN_POINT('Ctrl Pts',(81.7843698754555,-1.40586692489733,
54.2335295287399));
#167458=CARTESIAN_POINT('Ctrl Pts',(81.8543822587684,-0.706555442065941,
54.2306241735281));
#167459=CARTESIAN_POINT('Ctrl Pts',(81.8691810274887,-0.473448102637126,
54.2310382586001));
#167460=CARTESIAN_POINT('Ctrl Pts',(81.876709007879,-0.193869574515561,
54.2330369605984));
#167461=CARTESIAN_POINT('Ctrl Pts',(81.8776189721871,-0.147688661319497,
54.2334160562138));
#167462=CARTESIAN_POINT('Ctrl Pts',(81.8785155688848,-0.0758478686663873,
54.234080293023));
#167463=CARTESIAN_POINT('Ctrl Pts',(81.8787328285037,-0.0501912685364171,
54.2343322902245));
#167464=CARTESIAN_POINT('Ctrl Pts',(81.8788835494623,-0.0163561638718441,
54.2346838626483));
#167465=CARTESIAN_POINT('Ctrl Pts',(81.8789095176102,-0.00817807648179977,
54.2347703219472));
#167466=CARTESIAN_POINT('Ctrl Pts',(81.8789250230948,-6.6822534455389E-11,
54.2348582579198));
#167467=CARTESIAN_POINT('Ctrl Pts',(81.8868193065938,6.72938151241379E-11,
54.2796289644064));
#167468=CARTESIAN_POINT('Ctrl Pts',(81.8868037018699,-0.00823041824879308,
54.2795404656197));
#167469=CARTESIAN_POINT('Ctrl Pts',(81.8867776276105,-0.0164608554629298,
54.279454185466));
#167470=CARTESIAN_POINT('Ctrl Pts',(81.8866270604485,-0.0503705596085221,
54.2791078230115));
#167471=CARTESIAN_POINT('Ctrl Pts',(81.8864111104939,-0.0760494735295417,
54.278867068142));
#167472=CARTESIAN_POINT('Ctrl Pts',(81.885520170495,-0.148012085361578,
54.2782521807275));
#167473=CARTESIAN_POINT('Ctrl Pts',(81.8846158847755,-0.19429262809756,
54.2779260690182));
#167474=CARTESIAN_POINT('Ctrl Pts',(81.8770833769293,-0.476365369618101,
54.2763542287265));
#167475=CARTESIAN_POINT('Ctrl Pts',(81.8621834322366,-0.711863574058764,
54.2768118075317));
#167476=CARTESIAN_POINT('Ctrl Pts',(81.7920732767064,-1.41217311362647,
54.2830428280544));
#167477=CARTESIAN_POINT('Ctrl Pts',(81.7117187716005,-1.87369743422597,
54.2935659156048));
#167478=CARTESIAN_POINT('Ctrl Pts',(81.5161550782977,-2.65481791695313,
54.3211319109903));
#167479=CARTESIAN_POINT('Ctrl Pts',(81.417008554657,-2.97760906953024,54.3355337051005));
#167480=CARTESIAN_POINT('Ctrl Pts',(81.2677700727074,-3.38543212348313,
54.3574666876688));
#167481=CARTESIAN_POINT('Ctrl Pts',(81.2330738320505,-3.47596250547474,
54.3625807460449));
#167482=CARTESIAN_POINT('Ctrl Pts',(81.1781839095376,-3.61292005473898,
54.3706907744574));
#167483=CARTESIAN_POINT('Ctrl Pts',(81.1589838217342,-3.65974753090069,
54.3735309824325));
#167484=CARTESIAN_POINT('Ctrl Pts',(81.1248644977962,-3.74111646184618,
54.3785837473697));
#167485=CARTESIAN_POINT('Ctrl Pts',(81.1101107507902,-3.77572765707751,
54.3807703886754));
#167486=CARTESIAN_POINT('Ctrl Pts',(81.076338802895,-3.85367587452407,54.3857795520443));
#167487=CARTESIAN_POINT('Ctrl Pts',(81.0572027854896,-3.89695956210476,
54.3886205267855));
#167488=CARTESIAN_POINT('Ctrl Pts',(81.0043244696569,-4.01420333350509,
54.3964781202221));
#167489=CARTESIAN_POINT('Ctrl Pts',(80.9699613206163,-4.08787240278888,
54.4015920273012));
#167490=CARTESIAN_POINT('Ctrl Pts',(80.7443601195198,-4.55584599192918,
54.4352164696084));
#167491=CARTESIAN_POINT('Ctrl Pts',(80.527237583365,-4.93678840350033,54.4677687397645));
#167492=CARTESIAN_POINT('Ctrl Pts',(80.1017226532291,-5.57665300903674,
54.5324213539537));
#167493=CARTESIAN_POINT('Ctrl Pts',(79.9044194825698,-5.84223042498021,
54.5626589915195));
#167494=CARTESIAN_POINT('Ctrl Pts',(79.6067873758376,-6.20210705450477,
54.6090097342164));
#167495=CARTESIAN_POINT('Ctrl Pts',(79.5174760262113,-6.30547627230742,
54.6230032598172));
#167496=CARTESIAN_POINT('Ctrl Pts',(79.3667349052224,-6.47252939326779,
54.6467993287517));
#167497=CARTESIAN_POINT('Ctrl Pts',(79.3065681871575,-6.53736276963142,
54.6563414959228));
#167498=CARTESIAN_POINT('Ctrl Pts',(79.2219102082595,-6.6260698475448,54.6698384333121));
#167499=CARTESIAN_POINT('Ctrl Pts',(79.1981696492827,-6.65067833943088,
54.6736308719257));
#167500=CARTESIAN_POINT('Ctrl Pts',(79.1575802967885,-6.69229930409101,
54.6801282601002));
#167501=CARTESIAN_POINT('Ctrl Pts',(79.1407979339267,-6.70937843699708,
54.6828185798356));
#167502=CARTESIAN_POINT('Ctrl Pts',(79.1056760786384,-6.74485188006904,
54.688457126974));
#167503=CARTESIAN_POINT('Ctrl Pts',(79.0873256160593,-6.76323446730563,
54.691407772179));
#167504=CARTESIAN_POINT('Ctrl Pts',(79.0377971948921,-6.81244368777388,
54.6993834460056));
#167505=CARTESIAN_POINT('Ctrl Pts',(79.0064830248739,-6.84312743315383,
54.7044384949753));
#167506=CARTESIAN_POINT('Ctrl Pts',(78.8577788876661,-6.98682863128549,
54.7284974879095));
#167507=CARTESIAN_POINT('Ctrl Pts',(78.7377467747131,-7.09697545809167,
54.7480734480863));
#167508=CARTESIAN_POINT('Ctrl Pts',(78.2604321110614,-7.51275769315889,
54.8263212499131));
#167509=CARTESIAN_POINT('Ctrl Pts',(77.8837213471018,-7.79429326005309,
54.888888481178));
#167510=CARTESIAN_POINT('Ctrl Pts',(77.2952406566751,-8.16870785841258,
54.9864244522242));
#167511=CARTESIAN_POINT('Ctrl Pts',(77.0983037136312,-8.28410059184347,
55.0190409214751));
#167512=CARTESIAN_POINT('Ctrl Pts',(76.7644442175929,-8.46361131233401,
55.0741923601068));
#167513=CARTESIAN_POINT('Ctrl Pts',(76.629795718281,-8.53184688523183,55.0963993378599));
#167514=CARTESIAN_POINT('Ctrl Pts',(76.4397396027214,-8.62242491716268,
55.1276800750773));
#167515=CARTESIAN_POINT('Ctrl Pts',(76.3856613623745,-8.64756302150875,
55.1365735844978));
#167516=CARTESIAN_POINT('Ctrl Pts',(76.2926220992222,-8.68972937077951,
55.1518617802551));
#167517=CARTESIAN_POINT('Ctrl Pts',(76.2537770158542,-8.70701440027458,
55.1582410472903));
#167518=CARTESIAN_POINT('Ctrl Pts',(76.1794369346593,-8.7394850814779,55.1704421048029));
#167519=CARTESIAN_POINT('Ctrl Pts',(76.1439628269152,-8.75471737731974,
55.1762611373328));
#167520=CARTESIAN_POINT('Ctrl Pts',(76.060667530918,-8.78987106701651,55.1899171068255));
#167521=CARTESIAN_POINT('Ctrl Pts',(76.0127739782824,-8.80961403696841,
55.197763359345));
#167522=CARTESIAN_POINT('Ctrl Pts',(75.8464368736243,-8.87656163033207,
55.2249939961966));
#167523=CARTESIAN_POINT('Ctrl Pts',(75.7272031616995,-8.92172316593278,
55.2444785944213));
#167524=CARTESIAN_POINT('Ctrl Pts',(75.0259232068373,-9.17096521075283,
55.3588867249881));
#167525=CARTESIAN_POINT('Ctrl Pts',(74.4259354239074,-9.31900165167197,
55.4558785913282));
#167526=CARTESIAN_POINT('Ctrl Pts',(73.5724183466109,-9.44128635155178,
55.5943132607097));
#167527=CARTESIAN_POINT('Ctrl Pts',(73.3275401402027,-9.46646571011397,
55.634100334039));
#167528=CARTESIAN_POINT('Ctrl Pts',(72.9521054300962,-9.49000543493065,
55.6954207829239));
#167529=CARTESIAN_POINT('Ctrl Pts',(72.8220630485322,-9.49540910087137,
55.7167199876299));
#167530=CARTESIAN_POINT('Ctrl Pts',(72.6545134984376,-9.49883368609103,
55.7442694109516));
#167531=CARTESIAN_POINT('Ctrl Pts',(72.6170584157632,-9.49937169626509,
55.7504348799275));
#167532=CARTESIAN_POINT('Ctrl Pts',(72.5563369146072,-9.49987505736842,
55.7604423812777));
#167533=CARTESIAN_POINT('Ctrl Pts',(72.533071295167,-9.49998014100829,55.7642796773405));
#167534=CARTESIAN_POINT('Ctrl Pts',(72.4878830151827,-9.50001374574615,
55.7717386722315));
#167535=CARTESIAN_POINT('Ctrl Pts',(72.4659605421489,-9.49995210358764,
55.7753600209924));
#167536=CARTESIAN_POINT('Ctrl Pts',(72.4170057908746,-9.49964038424899,
55.7834525983054));
#167537=CARTESIAN_POINT('Ctrl Pts',(72.3899741255588,-9.49934972106651,
55.7879250733794));
#167538=CARTESIAN_POINT('Ctrl Pts',(72.2964396983423,-9.49793374924685,
55.8034134415145));
#167539=CARTESIAN_POINT('Ctrl Pts',(72.229950790923,-9.49620948254141,55.8144457275155));
#167540=CARTESIAN_POINT('Ctrl Pts',(71.7866313366997,-9.47992427102733,
55.8881297435857));
#167541=CARTESIAN_POINT('Ctrl Pts',(71.4110379251485,-9.44303607424208,
55.9511495569013));
#167542=CARTESIAN_POINT('Ctrl Pts',(70.7172642198884,-9.33174774183496,
56.0676029860616));
#167543=CARTESIAN_POINT('Ctrl Pts',(70.3987366952597,-9.26325038407453,
56.1210890401528));
#167544=CARTESIAN_POINT('Ctrl Pts',(69.8766655397566,-9.12184068168485,
56.2083646637515));
#167545=CARTESIAN_POINT('Ctrl Pts',(69.6709542908296,-9.05836433057767,
56.242652596755));
#167546=CARTESIAN_POINT('Ctrl Pts',(69.3287125709147,-8.93958729744622,
56.299452035826));
#167547=CARTESIAN_POINT('Ctrl Pts',(69.1909957221431,-8.8881029202051,56.322239704473));
#167548=CARTESIAN_POINT('Ctrl Pts',(68.9996358021361,-8.81135074198667,
56.3537970112849));
#167549=CARTESIAN_POINT('Ctrl Pts',(68.9449600838455,-8.78881425229208,
56.3628012879568));
#167550=CARTESIAN_POINT('Ctrl Pts',(68.8514281424868,-8.74921605380204,
56.3781829672609));
#167551=CARTESIAN_POINT('Ctrl Pts',(68.812470285213,-8.73240809088499,56.3845832277817));
#167552=CARTESIAN_POINT('Ctrl Pts',(68.7381919134569,-8.6997583007703,56.3967736410281));
#167553=CARTESIAN_POINT('Ctrl Pts',(68.702853200618,-8.68396160806406,56.4025678856032));
#167554=CARTESIAN_POINT('Ctrl Pts',(68.6200689469886,-8.64633643453006,
56.4161285633606));
#167555=CARTESIAN_POINT('Ctrl Pts',(68.5727039291519,-8.624327598275,56.423877293998));
#167556=CARTESIAN_POINT('Ctrl Pts',(68.4078159950103,-8.54602077316438,
56.4508174735786));
#167557=CARTESIAN_POINT('Ctrl Pts',(68.2912611519676,-8.48764796319075,
56.4697982471763));
#167558=CARTESIAN_POINT('Ctrl Pts',(67.5793662104695,-8.1122919378659,56.5853619099856));
#167559=CARTESIAN_POINT('Ctrl Pts',(67.0176567205434,-7.73366920555861,
56.6747601265172));
#167560=CARTESIAN_POINT('Ctrl Pts',(66.3936889914479,-7.20712609555206,
56.7740190118674));
#167561=CARTESIAN_POINT('Ctrl Pts',(66.2885975073678,-7.1143472560409,56.7907420525393));
#167562=CARTESIAN_POINT('Ctrl Pts',(66.1193907420373,-6.9581012129157,56.8177211283103));
#167563=CARTESIAN_POINT('Ctrl Pts',(66.0540595389005,-6.89601330030935,
56.8281516063107));
#167564=CARTESIAN_POINT('Ctrl Pts',(65.9649996469558,-6.80890678809975,
56.8424005375566));
#167565=CARTESIAN_POINT('Ctrl Pts',(65.9405099979431,-6.78469000345276,
56.8463219235067));
#167566=CARTESIAN_POINT('Ctrl Pts',(65.899188550292,-6.74337810233011,56.852944743338));
#167567=CARTESIAN_POINT('Ctrl Pts',(65.8822888792217,-6.72635272886875,
56.855655153581));
#167568=CARTESIAN_POINT('Ctrl Pts',(65.8472931773515,-6.69082622875994,
56.8612718896173));
#167569=CARTESIAN_POINT('Ctrl Pts',(65.8292079467307,-6.67231469713399,
56.8641767589549));
#167570=CARTESIAN_POINT('Ctrl Pts',(65.7809920204501,-6.62255371399367,
56.8719266870697));
#167571=CARTESIAN_POINT('Ctrl Pts',(65.7509991775424,-6.59116869957959,
56.8767532827162));
#167572=CARTESIAN_POINT('Ctrl Pts',(65.6128974275168,-6.44464405239583,
56.898999590071));
#167573=CARTESIAN_POINT('Ctrl Pts',(65.507447205033,-6.32697784859078,56.9160499571423));
#167574=CARTESIAN_POINT('Ctrl Pts',(65.1420317544909,-5.8980725068684,56.975210507752));
#167575=CARTESIAN_POINT('Ctrl Pts',(64.8990033414979,-5.57263290037703,
57.0146840597765));
#167576=CARTESIAN_POINT('Ctrl Pts',(64.4717379677446,-4.91695987548984,
57.083195157016));
#167577=CARTESIAN_POINT('Ctrl Pts',(64.2848892206694,-4.5893974135785,57.1127221172638));
#167578=CARTESIAN_POINT('Ctrl Pts',(64.0729657225697,-4.16105504507071,
57.1452644213271));
#167579=CARTESIAN_POINT('Ctrl Pts',(64.0296653390984,-4.06995170992162,
57.1518549610581));
#167580=CARTESIAN_POINT('Ctrl Pts',(63.966485534597,-3.93143776181582,57.1613762839153));
#167581=CARTESIAN_POINT('Ctrl Pts',(63.9455440509895,-3.884534038266,57.1645153554872));
#167582=CARTESIAN_POINT('Ctrl Pts',(63.908281739838,-3.7992463703181,57.1700694168243));
#167583=CARTESIAN_POINT('Ctrl Pts',(63.8918334329776,-3.76092119762157,
57.1725094374628));
#167584=CARTESIAN_POINT('Ctrl Pts',(63.85691038023,-3.67806662401944,57.1776644374106));
#167585=CARTESIAN_POINT('Ctrl Pts',(63.8385196576617,-3.63350205716523,
57.1803629549147));
#167586=CARTESIAN_POINT('Ctrl Pts',(63.789341906914,-3.5117477624044,57.1875340169673));
#167587=CARTESIAN_POINT('Ctrl Pts',(63.7592157228958,-3.43428818390488,
57.1918770682651));
#167588=CARTESIAN_POINT('Ctrl Pts',(63.5651731218812,-2.91559575363422,
57.2195078839532));
#167589=CARTESIAN_POINT('Ctrl Pts',(63.4326760499285,-2.46298503603752,
57.2366247678939));
#167590=CARTESIAN_POINT('Ctrl Pts',(63.2624592385337,-1.67037294422955,
57.2554586820962));
#167591=CARTESIAN_POINT('Ctrl Pts',(63.2087284589601,-1.33479508682692,
57.260140361922));
#167592=CARTESIAN_POINT('Ctrl Pts',(63.1459354028104,-0.743838779650244,
57.2631843828959));
#167593=CARTESIAN_POINT('Ctrl Pts',(63.1290859331298,-0.489639754540127,
57.2628367014751));
#167594=CARTESIAN_POINT('Ctrl Pts',(63.1211546198795,-0.189312912893192,
57.2606668808862));
#167595=CARTESIAN_POINT('Ctrl Pts',(63.1202733895077,-0.143535259063808,
57.2602880834199));
#167596=CARTESIAN_POINT('Ctrl Pts',(63.1194141866416,-0.0724641262934447,
57.2596269751481));
#167597=CARTESIAN_POINT('Ctrl Pts',(63.1192084689173,-0.0471737837894489,
57.2593773729443));
#167598=CARTESIAN_POINT('Ctrl Pts',(63.1190114576078,-2.04737978380578E-5,
57.2588855669708));
#167599=CARTESIAN_POINT('Ctrl Pts',(63.1189948859015,0.0218420668010453,
57.258646985011));
#167600=CARTESIAN_POINT('Ctrl Pts',(63.1191287671181,0.0721426862078172,
57.2580736336732));
#167601=CARTESIAN_POINT('Ctrl Pts',(63.1193309530555,0.100580271569169,
57.2577314917698));
#167602=CARTESIAN_POINT('Ctrl Pts',(63.1203626406985,0.189851770932978,
57.2566001002843));
#167603=CARTESIAN_POINT('Ctrl Pts',(63.1216443936129,0.250678078777477,
57.2557456106451));
#167604=CARTESIAN_POINT('Ctrl Pts',(63.1398670833702,0.846485663990278,
57.2465312803745));
#167605=CARTESIAN_POINT('Ctrl Pts',(63.2009344777738,1.37905493293315,57.2315717722661));
#167606=CARTESIAN_POINT('Ctrl Pts',(63.3721367094694,2.23521474306536,57.19415244763));
#167607=CARTESIAN_POINT('Ctrl Pts',(63.4558681992518,2.56305616835908,57.1765078746579));
#167608=CARTESIAN_POINT('Ctrl Pts',(63.6162260837168,3.07654082556368,57.1431967522594));
#167609=CARTESIAN_POINT('Ctrl Pts',(63.6817628196879,3.26547650233007,57.1296733286947));
#167610=CARTESIAN_POINT('Ctrl Pts',(63.7768620419819,3.51428634893736,57.1101308051765));
#167611=CARTESIAN_POINT('Ctrl Pts',(63.8012512260684,3.57616085275525,57.1051252604647));
#167612=CARTESIAN_POINT('Ctrl Pts',(63.8428872728525,3.67865519099926,57.0965897280603));
#167613=CARTESIAN_POINT('Ctrl Pts',(63.8597769870129,3.71942331897871,57.0931297844375));
#167614=CARTESIAN_POINT('Ctrl Pts',(63.8934234783828,3.799079935851,57.0862418687314));
#167615=CARTESIAN_POINT('Ctrl Pts',(63.9101578701817,3.83797713646599,57.0828182919277));
#167616=CARTESIAN_POINT('Ctrl Pts',(63.9510740761863,3.93137309794328,57.0744527097932));
#167617=CARTESIAN_POINT('Ctrl Pts',(63.9755061514997,3.98575581396697,57.0694616178568));
#167618=CARTESIAN_POINT('Ctrl Pts',(64.0581023064795,4.16510719833506,57.0526025334797));
#167619=CARTESIAN_POINT('Ctrl Pts',(64.1184410654669,4.2890143959922,57.0403084101541));
#167620=CARTESIAN_POINT('Ctrl Pts',(64.2755507193237,4.59467902619919,57.0083602819718));
#167621=CARTESIAN_POINT('Ctrl Pts',(64.375532197232,4.77463967360553,56.9880824776893));
#167622=CARTESIAN_POINT('Ctrl Pts',(64.6954363090397,5.30892404169094,56.9234490492815));
#167623=CARTESIAN_POINT('Ctrl Pts',(64.9327033558509,5.65186047291621,56.8758116710857));
#167624=CARTESIAN_POINT('Ctrl Pts',(65.344671843749,6.17046539751304,56.7943294858255));
#167625=CARTESIAN_POINT('Ctrl Pts',(65.505200084583,6.35705412738364,56.7628333922726));
#167626=CARTESIAN_POINT('Ctrl Pts',(65.7057654761593,6.5724566231778,56.7239498664319));
#167627=CARTESIAN_POINT('Ctrl Pts',(65.7390233081084,6.60762506407441,56.7175167827929));
#167628=CARTESIAN_POINT('Ctrl Pts',(65.7913953224537,6.66215368229698,56.7074109980558));
#167629=CARTESIAN_POINT('Ctrl Pts',(65.8103263047558,6.68169321299162,56.7037629774392));
#167630=CARTESIAN_POINT('Ctrl Pts',(65.8441090356111,6.71625937858891,56.6972621319641));
#167631=CARTESIAN_POINT('Ctrl Pts',(65.8589273230657,6.73131904240498,56.694413750271));
#167632=CARTESIAN_POINT('Ctrl Pts',(65.8949340311389,6.7676654769623,56.6874999179495));
#167633=CARTESIAN_POINT('Ctrl Pts',(65.9161734442222,6.78890001361772,56.683427749291));
#167634=CARTESIAN_POINT('Ctrl Pts',(65.9829086578959,6.85498119570882,56.6706508300068));
#167635=CARTESIAN_POINT('Ctrl Pts',(66.0287568461807,6.89946017657578,56.6618988260408));
#167636=CARTESIAN_POINT('Ctrl Pts',(66.2723156567597,7.13095611329834,56.6155245836703));
#167637=CARTESIAN_POINT('Ctrl Pts',(66.4775491862603,7.30965534968785,56.5768509225591));
#167638=CARTESIAN_POINT('Ctrl Pts',(67.0611866175379,7.77472479341755,56.467343245114));
#167639=CARTESIAN_POINT('Ctrl Pts',(67.4537952850087,8.04139391636132,56.3941515890003));
#167640=CARTESIAN_POINT('Ctrl Pts',(68.0457325045604,8.38067072794395,56.283313414584));
#167641=CARTESIAN_POINT('Ctrl Pts',(68.2303616987859,8.47837889630691,56.2486860473544));
#167642=CARTESIAN_POINT('Ctrl Pts',(68.4798890797847,8.59984288548275,56.2017691035976));
#167643=CARTESIAN_POINT('Ctrl Pts',(68.542071822468,8.62926063095005,56.1900680069379));
#167644=CARTESIAN_POINT('Ctrl Pts',(68.6447844275995,8.67646059939143,56.1707240003661));
#167645=CARTESIAN_POINT('Ctrl Pts',(68.6851307638111,8.69465212420425,56.163121438763));
#167646=CARTESIAN_POINT('Ctrl Pts',(68.7639912199249,8.7295311722847,56.1482534071613));
#167647=CARTESIAN_POINT('Ctrl Pts',(68.8024919634255,8.74624753131575,56.1409908776346));
#167648=CARTESIAN_POINT('Ctrl Pts',(68.8937018660945,8.78511422443546,56.123776641423));
#167649=CARTESIAN_POINT('Ctrl Pts',(68.9465019527323,8.80703767293152,56.1138045186464));
#167650=CARTESIAN_POINT('Ctrl Pts',(69.1249833024015,8.87921367193621,56.080071700581));
#167651=CARTESIAN_POINT('Ctrl Pts',(69.2515314724431,8.92718294011467,56.0561144137714));
#167652=CARTESIAN_POINT('Ctrl Pts',(69.80064677166,9.12164225637417,55.95199917272));
#167653=CARTESIAN_POINT('Ctrl Pts',(70.2321408548675,9.23996980639693,55.8697468278977));
#167654=CARTESIAN_POINT('Ctrl Pts',(71.1508633070926,9.4212387163456,55.6945325578907));
#167655=CARTESIAN_POINT('Ctrl Pts',(71.638024782268,9.47742375588013,55.6015764133996));
#167656=CARTESIAN_POINT('Ctrl Pts',(72.1908326194499,9.49665741169594,55.4972673125214));
#167657=CARTESIAN_POINT('Ctrl Pts',(72.2542511321458,9.49820558948042,55.4853189269724));
#167658=CARTESIAN_POINT('Ctrl Pts',(72.3458787538574,9.49949179646944,55.4680860472043));
#167659=CARTESIAN_POINT('Ctrl Pts',(72.3740758937811,9.49975762128033,55.4627870035779));
#167660=CARTESIAN_POINT('Ctrl Pts',(72.4237917534768,9.49999715168168,55.4534517388633));
#167661=CARTESIAN_POINT('Ctrl Pts',(72.4453096387934,9.5000251487393,55.4494138531572));
#167662=CARTESIAN_POINT('Ctrl Pts',(72.491531012897,9.49992273774942,55.4407459632756));
#167663=CARTESIAN_POINT('Ctrl Pts',(72.5162342458354,9.49976827473747,55.4361167980933));
#167664=CARTESIAN_POINT('Ctrl Pts',(72.5852147286712,9.49905847464713,55.4231995156892));
#167665=CARTESIAN_POINT('Ctrl Pts',(72.62949042129,9.49828248070331,55.4149188553773));
#167666=CARTESIAN_POINT('Ctrl Pts',(72.9067772803576,9.49141566200921,55.3631176637781));
#167667=CARTESIAN_POINT('Ctrl Pts',(73.1395460441066,9.47677302352543,55.3198897289655));
#167668=CARTESIAN_POINT('Ctrl Pts',(73.714024217922,9.41862243577074,55.2134743335685));
#167669=CARTESIAN_POINT('Ctrl Pts',(74.0543921880827,9.36473494312402,55.1506582099894));
#167670=CARTESIAN_POINT('Ctrl Pts',(74.8522560221838,9.19204550163891,55.003079553422));
#167671=CARTESIAN_POINT('Ctrl Pts',(75.3053294102451,9.05685050371174,54.9189857956076));
#167672=CARTESIAN_POINT('Ctrl Pts',(75.8228749248785,8.85802325338984,54.8219893753125));
#167673=CARTESIAN_POINT('Ctrl Pts',(75.8990736192657,8.82757748403866,54.8076851870293));
#167674=CARTESIAN_POINT('Ctrl Pts',(76.0188162574668,8.7778718603371,54.7851684786556));
#167675=CARTESIAN_POINT('Ctrl Pts',(76.0626289979602,8.75928665798209,54.7769216225474));
#167676=CARTESIAN_POINT('Ctrl Pts',(76.1440697956621,8.72399449429642,54.7615765659813));
#167677=CARTESIAN_POINT('Ctrl Pts',(76.1817328979715,8.70737335412838,54.7544738619917));
#167678=CARTESIAN_POINT('Ctrl Pts',(76.2655280858635,8.66972244998581,54.7386573540621));
#167679=CARTESIAN_POINT('Ctrl Pts',(76.3116019393107,8.64856309857459,54.729951296251));
#167680=CARTESIAN_POINT('Ctrl Pts',(76.4476050615252,8.58474361194902,54.7042241205318));
#167681=CARTESIAN_POINT('Ctrl Pts',(76.5370324288022,8.54100418656501,54.6872706193047));
#167682=CARTESIAN_POINT('Ctrl Pts',(76.9570752956643,8.32708935194492,54.6074694624332));
#167683=CARTESIAN_POINT('Ctrl Pts',(77.2781409908186,8.13843080712285,54.5459502410746));
#167684=CARTESIAN_POINT('Ctrl Pts',(77.9199689617395,7.70745538556204,54.4222790011362));
#167685=CARTESIAN_POINT('Ctrl Pts',(78.2381877487167,7.46258772423397,54.3605624114115));
#167686=CARTESIAN_POINT('Ctrl Pts',(78.6601071376136,7.09244599352062,54.2788758867884));
#167687=CARTESIAN_POINT('Ctrl Pts',(78.7774915188021,6.98404469276734,54.2561691872502));
#167688=CARTESIAN_POINT('Ctrl Pts',(78.9232985676954,6.84235126356615,54.2280441028623));
#167689=CARTESIAN_POINT('Ctrl Pts',(78.9542723123117,6.81183177091451,54.2220742713647));
#167690=CARTESIAN_POINT('Ctrl Pts',(79.0033254038192,6.7628248574842,54.212628962011));
#167691=CARTESIAN_POINT('Ctrl Pts',(79.0215389084019,6.74447831159453,54.2091239331579));
#167692=CARTESIAN_POINT('Ctrl Pts',(79.056448810804,6.70902326234618,54.20241013013));
#167693=CARTESIAN_POINT('Ctrl Pts',(79.0731557501983,6.69192604687947,54.1991990400479));
#167694=CARTESIAN_POINT('Ctrl Pts',(79.1136326149226,6.65018771908824,54.1914237735947));
#167695=CARTESIAN_POINT('Ctrl Pts',(79.1373352345226,6.62547899080174,54.1868744302463));
#167696=CARTESIAN_POINT('Ctrl Pts',(79.2222437045098,6.53599742631999,54.170589365341));
#167697=CARTESIAN_POINT('Ctrl Pts',(79.2826817300576,6.47047242462857,54.1590198552344));
#167698=CARTESIAN_POINT('Ctrl Pts',(79.4344526743067,6.3011824070846,54.1300031374128));
#167699=CARTESIAN_POINT('Ctrl Pts',(79.5244771109269,6.19622697916207,54.1128263089429));
#167700=CARTESIAN_POINT('Ctrl Pts',(80.0206649713991,5.59140006542065,54.018190898994));
#167701=CARTESIAN_POINT('Ctrl Pts',(80.3779607811106,5.05223054293846,53.9500616685561));
#167702=CARTESIAN_POINT('Ctrl Pts',(80.750991426542,4.34143940072097,53.8765038719716));
#167703=CARTESIAN_POINT('Ctrl Pts',(80.8203985614988,4.20085520762842,53.8626887079181));
#167704=CARTESIAN_POINT('Ctrl Pts',(80.9126072188179,4.00185272323795,53.8441292860633));
#167705=CARTESIAN_POINT('Ctrl Pts',(80.9383356633627,3.94486238842252,53.8389262188333));
#167706=CARTESIAN_POINT('Ctrl Pts',(80.9791963853384,3.85192488606166,53.8306215137677));
#167707=CARTESIAN_POINT('Ctrl Pts',(80.9946704502021,3.81613489613762,53.8274663613728));
#167708=CARTESIAN_POINT('Ctrl Pts',(81.0266659859806,3.74086827871907,53.8209207703901));
#167709=CARTESIAN_POINT('Ctrl Pts',(81.0431423895596,3.70137283544941,53.8175374060662));
#167710=CARTESIAN_POINT('Ctrl Pts',(81.0819831308973,3.60647589560421,53.8095306694711));
#167711=CARTESIAN_POINT('Ctrl Pts',(81.1040951324315,3.550969796042,53.8049468573553));
#167712=CARTESIAN_POINT('Ctrl Pts',(81.1795353537772,3.35630096280034,53.7892164874625));
#167713=CARTESIAN_POINT('Ctrl Pts',(81.2301365437784,3.21607092444481,53.7784979647761));
#167714=CARTESIAN_POINT('Ctrl Pts',(81.3468862685882,2.86717061425798,53.7533360673316));
#167715=CARTESIAN_POINT('Ctrl Pts',(81.4092041237738,2.65726679501057,53.7395013044267));
#167716=CARTESIAN_POINT('Ctrl Pts',(81.5467546317825,2.12815756493666,53.707921581553));
#167717=CARTESIAN_POINT('Ctrl Pts',(81.6129330712187,1.8068051040015,53.6916640158221));
#167718=CARTESIAN_POINT('Ctrl Pts',(81.7203516780883,1.1056104425334,53.6628695973415));
#167719=CARTESIAN_POINT('Ctrl Pts',(81.7556859612981,0.725389215569644,
53.6513930117048));
#167720=CARTESIAN_POINT('Ctrl Pts',(81.770762177904,0.276630689451335,53.6432577887107));
#167721=CARTESIAN_POINT('Ctrl Pts',(81.7723223054978,0.209249832552093,
53.6421796521692));
#167722=CARTESIAN_POINT('Ctrl Pts',(81.7735285954149,0.114462559547364,
53.6408690767072));
#167723=CARTESIAN_POINT('Ctrl Pts',(81.7737611497979,0.0870672968790157,
53.6405145014626));
#167724=CARTESIAN_POINT('Ctrl Pts',(81.7739622678791,0.0397810590504774,
53.6399446357702));
#167725=CARTESIAN_POINT('Ctrl Pts',(81.7739857033185,0.0198905954865054,
53.639717801509));
#167726=CARTESIAN_POINT('Ctrl Pts',(81.7739479911102,4.5045009216105E-12,
53.6395039249478));
#167727=CARTESIAN_POINT('Origin',(73.0915550886457,-4.33680868994202E-16,
59.1075264962884));
#167728=CARTESIAN_POINT('',(81.653182392128,-6.03303474316641E-13,52.9546081790047));
#167729=CARTESIAN_POINT('',(81.6610766756267,2.23549780027555E-12,52.9993788854899));
#167730=CARTESIAN_POINT('',(82.4472287422617,-1.59709532818419E-15,57.4578688084528));
#167731=CARTESIAN_POINT('Ctrl Pts',(81.653182392128,-1.2050098533051E-12,
52.9546081790047));
#167732=CARTESIAN_POINT('Ctrl Pts',(81.6531851088897,0.00143290493713799,
52.9546235865264));
#167733=CARTESIAN_POINT('Ctrl Pts',(81.6531875044535,0.00286581046897979,
52.9546390393913));
#167734=CARTESIAN_POINT('Ctrl Pts',(81.6532233539634,0.0276294538124026,
52.954906881751));
#167735=CARTESIAN_POINT('Ctrl Pts',(81.6531719782427,0.0509601047422428,
52.9551712533422));
#167736=CARTESIAN_POINT('Ctrl Pts',(81.6528199849092,0.111121506211944,
52.9558843734276));
#167737=CARTESIAN_POINT('Ctrl Pts',(81.6523923386346,0.147950905939667,
52.9563512783029));
#167738=CARTESIAN_POINT('Ctrl Pts',(81.6498429068614,0.294719037309852,
52.9583351952227));
#167739=CARTESIAN_POINT('Ctrl Pts',(81.6460434811885,0.404616702112234,
52.9600964744945));
#167740=CARTESIAN_POINT('Ctrl Pts',(81.6098997609032,1.1027383561785,52.973133326473));
#167741=CARTESIAN_POINT('Ctrl Pts',(81.5254093008345,1.68682274318137,52.9924731025717));
#167742=CARTESIAN_POINT('Ctrl Pts',(81.2976027997886,2.63757270516619,53.0409794735188));
#167743=CARTESIAN_POINT('Ctrl Pts',(81.1841234582634,3.00995384298833,53.0645334646489));
#167744=CARTESIAN_POINT('Ctrl Pts',(81.0204259219582,3.44964165566448,53.098210734284));
#167745=CARTESIAN_POINT('Ctrl Pts',(80.9913830923766,3.52474759383711,53.1041758701733));
#167746=CARTESIAN_POINT('Ctrl Pts',(80.9438527680212,3.64321128628823,53.113924298331));
#167747=CARTESIAN_POINT('Ctrl Pts',(80.9259811660577,3.68682177005464,53.1175868337448));
#167748=CARTESIAN_POINT('Ctrl Pts',(80.891670631995,3.76881967294016,53.1246130337504));
#167749=CARTESIAN_POINT('Ctrl Pts',(80.8753004837309,3.80723579936609,53.1279632004791));
#167750=CARTESIAN_POINT('Ctrl Pts',(80.8376866807841,3.8939302308394,53.1356561269352));
#167751=CARTESIAN_POINT('Ctrl Pts',(80.8162954086813,3.94214038937022,53.1400278423351));
#167752=CARTESIAN_POINT('Ctrl Pts',(80.7598177594276,4.06664304053919,53.151561553844));
#167753=CARTESIAN_POINT('Ctrl Pts',(80.7241284528481,4.14264589344325,53.1588417186191));
#167754=CARTESIAN_POINT('Ctrl Pts',(80.4294920360104,4.74922187462374,53.2188741527783));
#167755=CARTESIAN_POINT('Ctrl Pts',(80.1233338937517,5.25448783642775,53.2809444792974));
#167756=CARTESIAN_POINT('Ctrl Pts',(79.7237134958812,5.79358726663658,53.3605176287432));
#167757=CARTESIAN_POINT('Ctrl Pts',(79.6737511995805,5.85917659460431,53.3704424175489));
#167758=CARTESIAN_POINT('Ctrl Pts',(79.5097164749224,6.06876597478054,53.4029364910156));
#167759=CARTESIAN_POINT('Ctrl Pts',(79.3923383649786,6.21003971940025,53.4260516114764));
#167760=CARTESIAN_POINT('Ctrl Pts',(79.2222549390406,6.4029690782621,53.4592784642033));
#167761=CARTESIAN_POINT('Ctrl Pts',(79.1729177195201,6.45762496457932,53.4688869845655));
#167762=CARTESIAN_POINT('Ctrl Pts',(79.085047662333,6.55269508357314,53.4859407161347));
#167763=CARTESIAN_POINT('Ctrl Pts',(79.0467839236783,6.59335992723495,53.4933477937378));
#167764=CARTESIAN_POINT('Ctrl Pts',(78.9884701807746,6.65423423061991,53.5046046812826));
#167765=CARTESIAN_POINT('Ctrl Pts',(78.968684236537,6.67470151227817,53.5084187919373));
#167766=CARTESIAN_POINT('Ctrl Pts',(78.9325019982952,6.71178997853067,53.5153833973951));
#167767=CARTESIAN_POINT('Ctrl Pts',(78.9161360582504,6.72844083122991,53.5185298331574));
#167768=CARTESIAN_POINT('Ctrl Pts',(78.8788110506641,6.76613270619697,53.525697237507));
#167769=CARTESIAN_POINT('Ctrl Pts',(78.8578144476744,6.78713494028236,53.5297231581496));
#167770=CARTESIAN_POINT('Ctrl Pts',(78.7926005123424,6.85174885958812,53.5422099226398));
#167771=CARTESIAN_POINT('Ctrl Pts',(78.7480532683087,6.89501657676172,53.5507149788459));
#167772=CARTESIAN_POINT('Ctrl Pts',(78.3634704344591,7.26119087314628,53.6239564857326));
#167773=CARTESIAN_POINT('Ctrl Pts',(78.000380645464,7.55826585105626,53.6919215589871));
#167774=CARTESIAN_POINT('Ctrl Pts',(77.234534061211,8.0942693626051,53.835106201599));
#167775=CARTESIAN_POINT('Ctrl Pts',(76.8329440448213,8.33257751035838,53.9101169267169));
#167776=CARTESIAN_POINT('Ctrl Pts',(76.343472575379,8.57532840246176,54.0021007685567));
#167777=CARTESIAN_POINT('Ctrl Pts',(76.2708120141278,8.6101916243388,54.0157679207733));
#167778=CARTESIAN_POINT('Ctrl Pts',(76.155271077027,8.66378755544133,54.0375220799395));
#167779=CARTESIAN_POINT('Ctrl Pts',(76.1126777352058,8.68315465012804,54.0455461222872));
#167780=CARTESIAN_POINT('Ctrl Pts',(76.032259849134,8.71898781551311,54.0607046032667));
#167781=CARTESIAN_POINT('Ctrl Pts',(75.9944673254759,8.73552589656495,54.0678319717392));
#167782=CARTESIAN_POINT('Ctrl Pts',(75.9089458313919,8.77227123416493,54.0839689281252));
#167783=CARTESIAN_POINT('Ctrl Pts',(75.8611572540474,8.79233033312754,54.0929918860099));
#167784=CARTESIAN_POINT('Ctrl Pts',(75.7190935229166,8.85056209863549,54.1198321712684));
#167785=CARTESIAN_POINT('Ctrl Pts',(75.624370986828,8.88757564336336,54.137750648613));
#167786=CARTESIAN_POINT('Ctrl Pts',(74.9725214106413,9.12996767661181,54.2612083882653));
#167787=CARTESIAN_POINT('Ctrl Pts',(74.3980220324031,9.28251995801431,54.3708687689541));
#167788=CARTESIAN_POINT('Ctrl Pts',(73.5275810894262,9.42553785836264,54.5368158118696));
#167789=CARTESIAN_POINT('Ctrl Pts',(73.2399592872618,9.45892242627501,54.5915958444191));
#167790=CARTESIAN_POINT('Ctrl Pts',(72.8081745632571,9.48843030376819,54.6734161688691));
#167791=CARTESIAN_POINT('Ctrl Pts',(72.664902405294,9.49485110491601,54.7004961134848));
#167792=CARTESIAN_POINT('Ctrl Pts',(72.482947966746,9.49873430675822,54.7347584843411));
#167793=CARTESIAN_POINT('Ctrl Pts',(72.4443661336139,9.49931425703466,54.7420161527846));
#167794=CARTESIAN_POINT('Ctrl Pts',(72.3823249654886,9.49985545800877,54.7536738683831));
#167795=CARTESIAN_POINT('Ctrl Pts',(72.3588682885446,9.49997013932155,54.7580784785989));
#167796=CARTESIAN_POINT('Ctrl Pts',(72.313724850805,9.50001777306765,54.7665493474078));
#167797=CARTESIAN_POINT('Ctrl Pts',(72.2920384406394,9.49996379472975,54.7706159664307));
#167798=CARTESIAN_POINT('Ctrl Pts',(72.2440334840176,9.49967417479822,54.7796121120073));
#167799=CARTESIAN_POINT('Ctrl Pts',(72.217715066986,9.49940219454825,54.7845404023461));
#167800=CARTESIAN_POINT('Ctrl Pts',(72.1239530773142,9.49802993961756,54.8020852443306));
#167801=CARTESIAN_POINT('Ctrl Pts',(72.0565169371262,9.49629951400901,54.814680590286));
#167802=CARTESIAN_POINT('Ctrl Pts',(71.6037718665759,9.47968824177278,54.8991102449892));
#167803=CARTESIAN_POINT('Ctrl Pts',(71.2195600721447,9.44129098303147,54.9701334413135));
#167804=CARTESIAN_POINT('Ctrl Pts',(70.4963812153249,9.32270896029754,55.1037906958956));
#167805=CARTESIAN_POINT('Ctrl Pts',(70.1573210241772,9.24721904033253,55.1664448247529));
#167806=CARTESIAN_POINT('Ctrl Pts',(69.5386556079521,9.07225515070606,55.2813054512462));
#167807=CARTESIAN_POINT('Ctrl Pts',(69.2580380363048,8.97809467536674,55.3336168206133));
#167808=CARTESIAN_POINT('Ctrl Pts',(68.9127885771729,8.84344769595115,55.3983622716093));
#167809=CARTESIAN_POINT('Ctrl Pts',(68.8435699668383,8.81548034045728,55.4113624996697));
#167810=CARTESIAN_POINT('Ctrl Pts',(68.7326953078154,8.76910983180753,55.4322187747066));
#167811=CARTESIAN_POINT('Ctrl Pts',(68.6908272496663,8.75123468941025,55.4401019652083));
#167812=CARTESIAN_POINT('Ctrl Pts',(68.6110447637958,8.71647272437077,55.4551384770455));
#167813=CARTESIAN_POINT('Ctrl Pts',(68.573109055057,8.69963870183839,55.4622945180514));
#167814=CARTESIAN_POINT('Ctrl Pts',(68.4868379884985,8.66065792082803,55.4785828776011));
#167815=CARTESIAN_POINT('Ctrl Pts',(68.43857622262,8.63834780040543,55.4877053980935));
#167816=CARTESIAN_POINT('Ctrl Pts',(68.3104888284529,8.57778970720131,55.5119445636487));
#167817=CARTESIAN_POINT('Ctrl Pts',(68.2310082889168,8.53880633272851,55.5270145386497));
#167818=CARTESIAN_POINT('Ctrl Pts',(67.6843088897289,8.26085827462049,55.6308689310983));
#167819=CARTESIAN_POINT('Ctrl Pts',(67.2371836347527,7.98345115343855,55.7168833548564));
#167820=CARTESIAN_POINT('Ctrl Pts',(66.4981887656814,7.43331683276955,55.8597945435958));
#167821=CARTESIAN_POINT('Ctrl Pts',(66.1960621862242,7.177073485896,55.9184558384286));
#167822=CARTESIAN_POINT('Ctrl Pts',(65.8735982952597,6.86652298197054,55.9806877483495));
#167823=CARTESIAN_POINT('Ctrl Pts',(65.8368435243893,6.83054137601503,55.9877747665752));
#167824=CARTESIAN_POINT('Ctrl Pts',(65.7808436989398,6.77481492282599,55.9985606407082));
#167825=CARTESIAN_POINT('Ctrl Pts',(65.7613920790619,6.75528785333911,56.0023048766362));
#167826=CARTESIAN_POINT('Ctrl Pts',(65.7255646139728,6.71900490908967,56.0091966734451));
#167827=CARTESIAN_POINT('Ctrl Pts',(65.7091656909039,6.70227339623416,56.0123493255522));
#167828=CARTESIAN_POINT('Ctrl Pts',(65.6716603088655,6.66372137156733,56.0195555168211));
#167829=CARTESIAN_POINT('Ctrl Pts',(65.6505956575853,6.6418589651321,56.0235998419343));
#167830=CARTESIAN_POINT('Ctrl Pts',(65.5831059764369,6.57113394912269,56.0365490096215));
#167831=CARTESIAN_POINT('Ctrl Pts',(65.537090243409,6.52186745495794,56.0453648242135));
#167832=CARTESIAN_POINT('Ctrl Pts',(65.262819257121,6.2218473032735,56.0978518841695));
#167833=CARTESIAN_POINT('Ctrl Pts',(65.0474346617468,5.95920004815421,56.1388297521726));
#167834=CARTESIAN_POINT('Ctrl Pts',(64.6753177678137,5.45208819192811,56.2099029650843));
#167835=CARTESIAN_POINT('Ctrl Pts',(64.5148227683445,5.21098492136576,56.2406723360261));
#167836=CARTESIAN_POINT('Ctrl Pts',(64.2580418784646,4.78410875016397,56.2904254571182));
#167837=CARTESIAN_POINT('Ctrl Pts',(64.1564379179796,4.60188570289519,56.3102803457906));
#167838=CARTESIAN_POINT('Ctrl Pts',(63.9957790516098,4.29005225111126,56.3420492100451));
#167839=CARTESIAN_POINT('Ctrl Pts',(63.933509024626,4.16223635293633,56.3544717913713));
#167840=CARTESIAN_POINT('Ctrl Pts',(63.8496329315514,3.97980697350209,56.3713777272633));
#167841=CARTESIAN_POINT('Ctrl Pts',(63.8256469086816,3.9263440003003,56.3762340682647));
#167842=CARTESIAN_POINT('Ctrl Pts',(63.7850808955849,3.83364602727304,56.3844862270183));
#167843=CARTESIAN_POINT('Ctrl Pts',(63.7682691639683,3.79451761693966,56.3879183162862));
#167844=CARTESIAN_POINT('Ctrl Pts',(63.7364764881869,3.71913351153391,56.3944326297103));
#167845=CARTESIAN_POINT('Ctrl Pts',(63.7214561696865,3.68289590952451,56.3975210036219));
#167846=CARTESIAN_POINT('Ctrl Pts',(63.6825726451172,3.58742611533613,56.4055446456523));
#167847=CARTESIAN_POINT('Ctrl Pts',(63.6590781258552,3.52804111868332,56.4104221198305));
#167848=CARTESIAN_POINT('Ctrl Pts',(63.5771757609427,3.31479246837527,56.427532869769));
#167849=CARTESIAN_POINT('Ctrl Pts',(63.5221382824121,3.15962410510045,56.4392369569967));
#167850=CARTESIAN_POINT('Ctrl Pts',(63.2674918484385,2.37820455941616,56.4944640878441));
#167851=CARTESIAN_POINT('Ctrl Pts',(63.1286276081184,1.73338423843806,56.5284354258869));
#167852=CARTESIAN_POINT('Ctrl Pts',(63.0282874495021,0.823225331996955,
56.5585928568498));
#167853=CARTESIAN_POINT('Ctrl Pts',(63.0103206638125,0.56632020372454,56.565157902973));
#167854=CARTESIAN_POINT('Ctrl Pts',(63.0007772661167,0.247950331523532,
56.5706941076219));
#167855=CARTESIAN_POINT('Ctrl Pts',(62.9995247559059,0.186916016119687,
56.5716373966359));
#167856=CARTESIAN_POINT('Ctrl Pts',(62.9985343941073,0.0975168026113216,
56.5728427199189));
#167857=CARTESIAN_POINT('Ctrl Pts',(62.9983446195951,0.0691597164579145,
56.5731990650259));
#167858=CARTESIAN_POINT('Ctrl Pts',(62.9982288146377,0.0189951161409549,
56.5737830627965));
#167859=CARTESIAN_POINT('Ctrl Pts',(62.998251979729,-0.00281185154086295,
56.5740214044755));
#167860=CARTESIAN_POINT('Ctrl Pts',(62.9984624304569,-0.0502878787672504,
56.5745064116745));
#167861=CARTESIAN_POINT('Ctrl Pts',(62.9986780614881,-0.0759564992473333,
56.5747471189385));
#167862=CARTESIAN_POINT('Ctrl Pts',(62.9995675392294,-0.147862838647288,
56.5753616857521));
#167863=CARTESIAN_POINT('Ctrl Pts',(63.0004701053835,-0.194097413028669,
56.5756876445601));
#167864=CARTESIAN_POINT('Ctrl Pts',(63.0079647818126,-0.475015389661,56.5772544889009));
#167865=CARTESIAN_POINT('Ctrl Pts',(63.022748548414,-0.709408209651014,
56.576808494219));
#167866=CARTESIAN_POINT('Ctrl Pts',(63.0925551452664,-1.40929162176869,
56.570630574318));
#167867=CARTESIAN_POINT('Ctrl Pts',(63.1728982913727,-1.8714855318355,56.5601138616527));
#167868=CARTESIAN_POINT('Ctrl Pts',(63.3685960529682,-2.65369613980434,
56.5325322891673));
#167869=CARTESIAN_POINT('Ctrl Pts',(63.4678384230203,-2.97691385881897,
56.5181169486992));
#167870=CARTESIAN_POINT('Ctrl Pts',(63.6172343928597,-3.38520712801605,
56.496160960067));
#167871=CARTESIAN_POINT('Ctrl Pts',(63.6519504746455,-3.47579523215722,
56.4910439961187));
#167872=CARTESIAN_POINT('Ctrl Pts',(63.706865966957,-3.61282150503926,56.4829302051978));
#167873=CARTESIAN_POINT('Ctrl Pts',(63.7260702405749,-3.6596605882726,56.4800893823114));
#167874=CARTESIAN_POINT('Ctrl Pts',(63.7601940837421,-3.74104224742202,
56.47503595405));
#167875=CARTESIAN_POINT('Ctrl Pts',(63.7749479961465,-3.7756546334831,56.4728492906534));
#167876=CARTESIAN_POINT('Ctrl Pts',(63.8087161835238,-3.85359592043542,
56.4678406903297));
#167877=CARTESIAN_POINT('Ctrl Pts',(63.8278481407165,-3.89687154779444,
56.465000321757));
#167878=CARTESIAN_POINT('Ctrl Pts',(63.8807041312365,-4.01406926395532,
56.45714605628));
#167879=CARTESIAN_POINT('Ctrl Pts',(63.9150481660042,-4.08770074481185,
56.4520350041243));
#167880=CARTESIAN_POINT('Ctrl Pts',(64.1380401797386,-4.5502906750407,56.4187995378315));
#167881=CARTESIAN_POINT('Ctrl Pts',(64.3518546959585,-4.92626548755453,
56.3867447015043));
#167882=CARTESIAN_POINT('Ctrl Pts',(64.7679436043986,-5.55452725632516,
56.323546326405));
#167883=CARTESIAN_POINT('Ctrl Pts',(64.9590468267763,-5.81354188317332,
56.2942773865799));
#167884=CARTESIAN_POINT('Ctrl Pts',(65.2552181614526,-6.17510824662347,
56.2482168567204));
#167885=CARTESIAN_POINT('Ctrl Pts',(65.3502536701254,-6.28582711028667,
56.2333424992836));
#167886=CARTESIAN_POINT('Ctrl Pts',(65.5097323844737,-6.46319745322292,
56.2081822474878));
#167887=CARTESIAN_POINT('Ctrl Pts',(65.5726924888361,-6.53119281418251,
56.1982011833488));
#167888=CARTESIAN_POINT('Ctrl Pts',(65.6606438943671,-6.6234339050194,56.1841815056031));
#167889=CARTESIAN_POINT('Ctrl Pts',(65.6848026362384,-6.64849355766373,
56.1803227786715));
#167890=CARTESIAN_POINT('Ctrl Pts',(65.7258877429669,-6.69064443696378,
56.1737466721988));
#167891=CARTESIAN_POINT('Ctrl Pts',(65.7427435270944,-6.70780646726806,
56.1710448328442));
#167892=CARTESIAN_POINT('Ctrl Pts',(65.777775226757,-6.7432044849496,56.1654212360849));
#167893=CARTESIAN_POINT('Ctrl Pts',(65.7959602430942,-6.76143069855299,
56.162497473426));
#167894=CARTESIAN_POINT('Ctrl Pts',(65.8445767290485,-6.80976217323059,
56.1546694742757));
#167895=CARTESIAN_POINT('Ctrl Pts',(65.8751359114217,-6.83973353817258,
56.1497370796754));
#167896=CARTESIAN_POINT('Ctrl Pts',(66.014527895092,-6.97460362589823,56.1271892000794));
#167897=CARTESIAN_POINT('Ctrl Pts',(66.1256174938266,-7.07705554811865,
56.1090847317394));
#167898=CARTESIAN_POINT('Ctrl Pts',(66.6011782138914,-7.49497911654568,
56.0311925169791));
#167899=CARTESIAN_POINT('Ctrl Pts',(66.9866843808187,-7.78459586609376,
55.9671611342368));
#167900=CARTESIAN_POINT('Ctrl Pts',(67.5859016687395,-8.16636221186927,
55.867844530841));
#167901=CARTESIAN_POINT('Ctrl Pts',(67.7838182941223,-8.28244277363937,
55.8350649478133));
#167902=CARTESIAN_POINT('Ctrl Pts',(68.1191630341652,-8.4628544801865,55.7796672818617));
#167903=CARTESIAN_POINT('Ctrl Pts',(68.2542864395813,-8.53135611121289,
55.75738170233));
#167904=CARTESIAN_POINT('Ctrl Pts',(68.4448998313424,-8.62221424464514,
55.7260090837402));
#167905=CARTESIAN_POINT('Ctrl Pts',(68.4990495165836,-8.6473887957525,55.717103787401));
#167906=CARTESIAN_POINT('Ctrl Pts',(68.5921736776358,-8.68959768876844,
55.7018015936054));
#167907=CARTESIAN_POINT('Ctrl Pts',(68.6310316564608,-8.70689003262623,
55.6954201900798));
#167908=CARTESIAN_POINT('Ctrl Pts',(68.7053705143828,-8.73936296670161,
55.683219299872));
#167909=CARTESIAN_POINT('Ctrl Pts',(68.7408303490545,-8.75459055774761,
55.6774025913991));
#167910=CARTESIAN_POINT('Ctrl Pts',(68.8240529088259,-8.78971711156529,
55.6637585034054));
#167911=CARTESIAN_POINT('Ctrl Pts',(68.8718876798237,-8.80943844854408,
55.6559218490915));
#167912=CARTESIAN_POINT('Ctrl Pts',(69.0387102451521,-8.87659239012893,
55.6286116045841));
#167913=CARTESIAN_POINT('Ctrl Pts',(69.1584974517625,-8.92195827496836,
55.6090366256135));
#167914=CARTESIAN_POINT('Ctrl Pts',(69.860076405798,-9.1712007918962,55.4945809437024));
#167915=CARTESIAN_POINT('Ctrl Pts',(70.4597761055783,-9.31911243207795,
55.3976358060226));
#167916=CARTESIAN_POINT('Ctrl Pts',(71.312916881783,-9.44131278489087,55.2592619483569));
#167917=CARTESIAN_POINT('Ctrl Pts',(71.5577185115048,-9.46647872083246,
55.219487219222));
#167918=CARTESIAN_POINT('Ctrl Pts',(71.9330506369443,-9.49000828287909,
55.1581834452261));
#167919=CARTESIAN_POINT('Ctrl Pts',(72.063067470748,-9.49541013754424,55.1368884032225));
#167920=CARTESIAN_POINT('Ctrl Pts',(72.2305889448303,-9.49883387908354,
55.1093435881339));
#167921=CARTESIAN_POINT('Ctrl Pts',(72.2680415273798,-9.4993718082175,55.1031785292554));
#167922=CARTESIAN_POINT('Ctrl Pts',(72.3287599772102,-9.49987509549167,
55.0931715291942));
#167923=CARTESIAN_POINT('Ctrl Pts',(72.3520250457068,-9.49998016012502,
55.089334323441));
#167924=CARTESIAN_POINT('Ctrl Pts',(72.3972131050212,-9.500013736652,55.0818753640039));
#167925=CARTESIAN_POINT('Ctrl Pts',(72.4191359083683,-9.49995207878265,
55.0782539601697));
#167926=CARTESIAN_POINT('Ctrl Pts',(72.4680922735697,-9.49964031353047,
55.0701611148772));
#167927=CARTESIAN_POINT('Ctrl Pts',(72.4951252223416,-9.49934961123635,
55.0656884266296));
#167928=CARTESIAN_POINT('Ctrl Pts',(72.5886683472263,-9.4979334006619,55.0501986149061));
#167929=CARTESIAN_POINT('Ctrl Pts',(72.6551646646249,-9.49620878556374,
55.0391650947126));
#167930=CARTESIAN_POINT('Ctrl Pts',(73.0988234815666,-9.47990952994969,
54.9654246318891));
#167931=CARTESIAN_POINT('Ctrl Pts',(73.4747462493226,-9.4429671901786,54.9023490404419));
#167932=CARTESIAN_POINT('Ctrl Pts',(74.169641037568,-9.33141974889466,54.7857072993243));
#167933=CARTESIAN_POINT('Ctrl Pts',(74.4889513305227,-9.26267281084391,
54.7320900751759));
#167934=CARTESIAN_POINT('Ctrl Pts',(75.0110902310015,-9.12103469033791,
54.6448058161543));
#167935=CARTESIAN_POINT('Ctrl Pts',(75.216122770848,-9.05770880816632,54.6106320454121));
#167936=CARTESIAN_POINT('Ctrl Pts',(75.5573710626558,-8.93921899473136,
54.5539985361194));
#167937=CARTESIAN_POINT('Ctrl Pts',(75.6947643274422,-8.88784061888727,
54.5312647135036));
#167938=CARTESIAN_POINT('Ctrl Pts',(75.8857570873621,-8.81122667628798,
54.4997681387308));
#167939=CARTESIAN_POINT('Ctrl Pts',(75.9403840224649,-8.78870822776538,
54.4907719384913));
#167940=CARTESIAN_POINT('Ctrl Pts',(76.0338584860343,-8.74913172249382,
54.4753997662184));
#167941=CARTESIAN_POINT('Ctrl Pts',(76.0728073326654,-8.73232661046519,
54.4690010075488));
#167942=CARTESIAN_POINT('Ctrl Pts',(76.1470858955967,-8.69967488212756,
54.4568106014597));
#167943=CARTESIAN_POINT('Ctrl Pts',(76.1824337107016,-8.683873162942,54.4510148843723));
#167944=CARTESIAN_POINT('Ctrl Pts',(76.2652654183662,-8.64622399895604,
54.4374464836224));
#167945=CARTESIAN_POINT('Ctrl Pts',(76.3126685446303,-8.6241956621182,54.4296915558093));
#167946=CARTESIAN_POINT('Ctrl Pts',(76.4778281290465,-8.54575214227553,
54.4027071510864));
#167947=CARTESIAN_POINT('Ctrl Pts',(76.5946120932545,-8.48725291539084,
54.3836893058772));
#167948=CARTESIAN_POINT('Ctrl Pts',(77.2464981544172,-8.14343592709517,
54.277869002374));
#167949=CARTESIAN_POINT('Ctrl Pts',(77.7548048635759,-7.80868240634213,
54.1967720053534));
#167950=CARTESIAN_POINT('Ctrl Pts',(78.3706817865983,-7.3113176967463,54.0987980666803));
#167951=CARTESIAN_POINT('Ctrl Pts',(78.5102477533446,-7.19168995334135,
54.0766074567405));
#167952=CARTESIAN_POINT('Ctrl Pts',(78.7008295324219,-7.01839518237206,
54.0462398234681));
#167953=CARTESIAN_POINT('Ctrl Pts',(78.7548166020132,-6.96813372240287,
54.0376295895671));
#167954=CARTESIAN_POINT('Ctrl Pts',(78.8487185825342,-6.87862869911172,
54.0226321677738));
#167955=CARTESIAN_POINT('Ctrl Pts',(78.8888819606826,-6.83965684693043,
54.016210486688));
#167956=CARTESIAN_POINT('Ctrl Pts',(78.9490021813989,-6.78027037483051,
54.0065843383982));
#167957=CARTESIAN_POINT('Ctrl Pts',(78.9692148381762,-6.76012205677604,
54.0033456279937));
#167958=CARTESIAN_POINT('Ctrl Pts',(79.0058404977669,-6.72327949860582,
53.9974722478685));
#167959=CARTESIAN_POINT('Ctrl Pts',(79.0222829454009,-6.70661586250353,
53.9948336796945));
#167960=CARTESIAN_POINT('Ctrl Pts',(79.0595016347727,-6.66861413698908,
53.9888570075512));
#167961=CARTESIAN_POINT('Ctrl Pts',(79.0802393997811,-6.64723822955063,
53.9855240219263));
#167962=CARTESIAN_POINT('Ctrl Pts',(79.1440359318979,-6.58085173641304,
53.9752626894438));
#167963=CARTESIAN_POINT('Ctrl Pts',(79.186753643857,-6.53550864566605,53.968380522767));
#167964=CARTESIAN_POINT('Ctrl Pts',(79.5483377831547,-6.14400436424126,
53.9100533480883));
#167965=CARTESIAN_POINT('Ctrl Pts',(79.8416142209471,-5.77457148759858,
53.8622838239147));
#167966=CARTESIAN_POINT('Ctrl Pts',(80.3708586533091,-4.99547711129451,
53.7771091168074));
#167967=CARTESIAN_POINT('Ctrl Pts',(80.6062308265866,-4.58701194791107,
53.7398057883377));
#167968=CARTESIAN_POINT('Ctrl Pts',(80.8462381816745,-4.08905797442266,
53.7031622174816));
#167969=CARTESIAN_POINT('Ctrl Pts',(80.8807176040813,-4.0151287727142,53.6979376914601));
#167970=CARTESIAN_POINT('Ctrl Pts',(80.9337350371828,-3.89756652116829,
53.6899704515841));
#167971=CARTESIAN_POINT('Ctrl Pts',(80.9528956660566,-3.85422707012049,
53.687105600925));
#167972=CARTESIAN_POINT('Ctrl Pts',(80.9883517264494,-3.77239880783103,
53.6818323773236));
#167973=CARTESIAN_POINT('Ctrl Pts',(81.0047178280493,-3.73394275719147,
53.679410119329));
#167974=CARTESIAN_POINT('Ctrl Pts',(81.0410858170288,-3.646918087512,53.6740546748789));
#167975=CARTESIAN_POINT('Ctrl Pts',(81.0609422827981,-3.5982884438105,53.6711499899173));
#167976=CARTESIAN_POINT('Ctrl Pts',(81.1185961564571,-3.45372068577784,
53.6627746923882));
#167977=CARTESIAN_POINT('Ctrl Pts',(81.1552558234924,-3.35732440722175,
53.6575269593339));
#167978=CARTESIAN_POINT('Ctrl Pts',(81.3954166105477,-2.69395378083437,
53.6236990299759));
#167979=CARTESIAN_POINT('Ctrl Pts',(81.5470779541456,-2.1091564217122,53.6053174237616));
#167980=CARTESIAN_POINT('Ctrl Pts',(81.6900577174245,-1.22312945548832,
53.5925709806086));
#167981=CARTESIAN_POINT('Ctrl Pts',(81.7236322173041,-0.930354280515686,
53.5907155989023));
#167982=CARTESIAN_POINT('Ctrl Pts',(81.7536654417887,-0.490907646989111,
53.5911051470487));
#167983=CARTESIAN_POINT('Ctrl Pts',(81.7602996923846,-0.345106621283968,
53.5917525887928));
#167984=CARTESIAN_POINT('Ctrl Pts',(81.7644966198225,-0.159963493406468,
53.5931914921324));
#167985=CARTESIAN_POINT('Ctrl Pts',(81.7651455184341,-0.120707251723698,
53.5935317274066));
#167986=CARTESIAN_POINT('Ctrl Pts',(81.7658013224872,-0.0575839547028548,
53.5941342791524));
#167987=CARTESIAN_POINT('Ctrl Pts',(81.7659601909634,-0.0337187247201237,
53.5943748322806));
#167988=CARTESIAN_POINT('Ctrl Pts',(81.7660395656254,-0.00656885437556106,
53.5946628240841));
#167989=CARTESIAN_POINT('Ctrl Pts',(81.7660474803996,-0.00328442583511579,
53.5946979021895));
#167990=CARTESIAN_POINT('Ctrl Pts',(81.7660537076114,-1.08793519407556E-11,
53.5947332184626));
#167991=CARTESIAN_POINT('Ctrl Pts',(81.7739479911102,4.5045009216105E-12,
53.6395039249478));
#167992=CARTESIAN_POINT('Ctrl Pts',(81.7739435788723,-0.0023271519310627,
53.6394789019034));
#167993=CARTESIAN_POINT('Ctrl Pts',(81.7739383296181,-0.00465430567239209,
53.6394540562307));
#167994=CARTESIAN_POINT('Ctrl Pts',(81.7738705745845,-0.0305610931805376,
53.6391794376136));
#167995=CARTESIAN_POINT('Ctrl Pts',(81.7737229710217,-0.0541406115829586,
53.6389476853336));
#167996=CARTESIAN_POINT('Ctrl Pts',(81.7731133581065,-0.115682941145436,
53.6383899097105));
#167997=CARTESIAN_POINT('Ctrl Pts',(81.7725144821153,-0.153644232417719,
53.6380926315016));
#167998=CARTESIAN_POINT('Ctrl Pts',(81.7688374252251,-0.323482709412806,
53.6369690995888));
#167999=CARTESIAN_POINT('Ctrl Pts',(81.7632915785597,-0.455295166218249,
53.6366541539024));
#168000=CARTESIAN_POINT('Ctrl Pts',(81.7394807488555,-0.835862496200755,
53.6372823187662));
#168001=CARTESIAN_POINT('Ctrl Pts',(81.7142958664717,-1.08407074726912,
53.6395935649047));
#168002=CARTESIAN_POINT('Ctrl Pts',(81.5924716314608,-1.94936756526757,
53.6537996749283));
#168003=CARTESIAN_POINT('Ctrl Pts',(81.4456102316304,-2.55761463047674,
53.6747380167085));
#168004=CARTESIAN_POINT('Ctrl Pts',(81.1986495746275,-3.26826109240764,
53.7109029249683));
#168005=CARTESIAN_POINT('Ctrl Pts',(81.1540428298269,-3.38874829255497,
53.7174645646486));
#168006=CARTESIAN_POINT('Ctrl Pts',(81.087941795081,-3.55682559483755,53.7272210815887));
#168007=CARTESIAN_POINT('Ctrl Pts',(81.0684557847543,-3.60520834751748,
53.7301009338568));
#168008=CARTESIAN_POINT('Ctrl Pts',(81.0337331261786,-3.6894292577611,53.7352387300448));
#168009=CARTESIAN_POINT('Ctrl Pts',(81.0186708254145,-3.72533957941291,
53.7374693613516));
#168010=CARTESIAN_POINT('Ctrl Pts',(80.9865333797313,-3.8006662385055,53.7422326164722));
#168011=CARTESIAN_POINT('Ctrl Pts',(80.9694112848591,-3.84006112394793,
53.7447725953886));
#168012=CARTESIAN_POINT('Ctrl Pts',(80.9275832170625,-3.93455336022793,
53.7509828505172));
#168013=CARTESIAN_POINT('Ctrl Pts',(80.902620584541,-3.98953237409775,53.7546933318891));
#168014=CARTESIAN_POINT('Ctrl Pts',(80.8123136977879,-4.18352510474944,
53.7681318751447));
#168015=CARTESIAN_POINT('Ctrl Pts',(80.7441527510494,-4.32117009628719,
53.7783016409775));
#168016=CARTESIAN_POINT('Ctrl Pts',(80.5643579982684,-4.66324994061301,
53.8052075804389));
#168017=CARTESIAN_POINT('Ctrl Pts',(80.4485274313295,-4.8653104872372,53.8226098499921));
#168018=CARTESIAN_POINT('Ctrl Pts',(80.0798593958943,-5.4571323354101,53.8783380774478));
#168019=CARTESIAN_POINT('Ctrl Pts',(79.8059598832282,-5.83260429851963,
53.9201398194718));
#168020=CARTESIAN_POINT('Ctrl Pts',(79.3990001339462,-6.31256365636161,
53.9837484290553));
#168021=CARTESIAN_POINT('Ctrl Pts',(79.2886415813603,-6.43602604468151,
54.0011305791617));
#168022=CARTESIAN_POINT('Ctrl Pts',(79.1448752567326,-6.58864459546846,
54.0239966366722));
#168023=CARTESIAN_POINT('Ctrl Pts',(79.1143654252176,-6.62058356424803,
54.0288613989999));
#168024=CARTESIAN_POINT('Ctrl Pts',(79.0655146741229,-6.67101344014595,
54.0366712996995));
#168025=CARTESIAN_POINT('Ctrl Pts',(79.0473161370937,-6.68964619426383,
54.0395852455076));
#168026=CARTESIAN_POINT('Ctrl Pts',(79.0122623193101,-6.72524215981955,
54.0452070213877));
#168027=CARTESIAN_POINT('Ctrl Pts',(78.9954190497796,-6.74221713054289,
54.0479122341511));
#168028=CARTESIAN_POINT('Ctrl Pts',(78.954464104476,-6.78318141256307,54.0544992800625));
#168029=CARTESIAN_POINT('Ctrl Pts',(78.9302883451521,-6.80710395385358,
54.0583952896698));
#168030=CARTESIAN_POINT('Ctrl Pts',(78.8436411808546,-6.89192562861749,
54.0723843141305));
#168031=CARTESIAN_POINT('Ctrl Pts',(78.7804709522617,-6.95207928737868,
54.082629881807));
#168032=CARTESIAN_POINT('Ctrl Pts',(78.618253936078,-7.10232838853546,54.1090375827375));
#168033=CARTESIAN_POINT('Ctrl Pts',(78.5181286810934,-7.19119057019406,
54.1254268511999));
#168034=CARTESIAN_POINT('Ctrl Pts',(78.1629462060085,-7.49315467367921,
54.1837812503194));
#168035=CARTESIAN_POINT('Ctrl Pts',(77.8987140240129,-7.69472446669826,
54.2275599272912));
#168036=CARTESIAN_POINT('Ctrl Pts',(77.264300242671,-8.12742409278371,54.3327211296841));
#168037=CARTESIAN_POINT('Ctrl Pts',(76.8876626359836,-8.34744965195274,
54.3951721960963));
#168038=CARTESIAN_POINT('Ctrl Pts',(76.4250228660552,-8.5758891808143,54.4714026165396));
#168039=CARTESIAN_POINT('Ctrl Pts',(76.3523256671751,-8.61061911215167,
54.4833688334468));
#168040=CARTESIAN_POINT('Ctrl Pts',(76.2366258054512,-8.6640594022498,54.5023922734591));
#168041=CARTESIAN_POINT('Ctrl Pts',(76.1939116151177,-8.68339820377563,
54.5094108686884));
#168042=CARTESIAN_POINT('Ctrl Pts',(76.116987926664,-8.71752705457139,54.5220422921981));
#168043=CARTESIAN_POINT('Ctrl Pts',(76.0828313107758,-8.73243635728515,
54.5276481375869));
#168044=CARTESIAN_POINT('Ctrl Pts',(76.002530235741,-8.76691456812469,54.5408203550892));
#168045=CARTESIAN_POINT('Ctrl Pts',(75.9563166060691,-8.78631597794009,
54.5483956828099));
#168046=CARTESIAN_POINT('Ctrl Pts',(75.8211527954778,-8.84177934234442,
54.5705360162297));
#168047=CARTESIAN_POINT('Ctrl Pts',(75.7318054675107,-8.87683564604249,
54.5851517050483));
#168048=CARTESIAN_POINT('Ctrl Pts',(75.3293014073264,-9.0276104052791,54.650908246581));
#168049=CARTESIAN_POINT('Ctrl Pts',(75.0106843999781,-9.12774682512769,
54.7027176279918));
#168050=CARTESIAN_POINT('Ctrl Pts',(74.2396112397559,-9.3251214178566,54.8277914888407));
#168051=CARTESIAN_POINT('Ctrl Pts',(73.783972807736,-9.40608394327155,54.901438813675));
#168052=CARTESIAN_POINT('Ctrl Pts',(73.092669241097,-9.47622175434809,55.0138724992235));
#168053=CARTESIAN_POINT('Ctrl Pts',(72.8601880300136,-9.49097913818975,
55.0518073070235));
#168054=CARTESIAN_POINT('Ctrl Pts',(72.5817834234466,-9.49812562146044,
55.0975408063158));
#168055=CARTESIAN_POINT('Ctrl Pts',(72.5361119356159,-9.49895960144131,
55.1050531341384));
#168056=CARTESIAN_POINT('Ctrl Pts',(72.4650996505089,-9.49973028158489,
55.116750710549));
#168057=CARTESIAN_POINT('Ctrl Pts',(72.4397608132908,-9.49990115533811,
55.1209280512153));
#168058=CARTESIAN_POINT('Ctrl Pts',(72.3929060488989,-9.5000245869161,55.1286590755608));
#168059=CARTESIAN_POINT('Ctrl Pts',(72.3713904102209,-9.500006190287,55.1322117535819));
#168060=CARTESIAN_POINT('Ctrl Pts',(72.3219102349707,-9.49979122054929,
55.1403878330069));
#168061=CARTESIAN_POINT('Ctrl Pts',(72.2939465000311,-9.49954288575259,
55.1450128275175));
#168062=CARTESIAN_POINT('Ctrl Pts',(72.2058374496105,-9.49836070547216,
55.1595980445449));
#168063=CARTESIAN_POINT('Ctrl Pts',(72.145702023126,-9.49696685006281,55.1695711682019));
#168064=CARTESIAN_POINT('Ctrl Pts',(71.8323995737194,-9.48664504836688,
55.221613452924));
#168065=CARTESIAN_POINT('Ctrl Pts',(71.5796956094659,-9.46790170270744,
55.263869514766));
#168066=CARTESIAN_POINT('Ctrl Pts',(70.6761818374809,-9.36341453496009,
55.4153036215634));
#168067=CARTESIAN_POINT('Ctrl Pts',(70.0340001689457,-9.21881299824602,
55.523457096834));
#168068=CARTESIAN_POINT('Ctrl Pts',(69.2614117502248,-8.95628610894851,
55.651780029097));
#168069=CARTESIAN_POINT('Ctrl Pts',(69.1123853901585,-8.90135057236214,
55.6764546418972));
#168070=CARTESIAN_POINT('Ctrl Pts',(68.9065643467413,-8.81943700671664,
55.7104096977477));
#168071=CARTESIAN_POINT('Ctrl Pts',(68.8485657978985,-8.7956736413379,55.719964133609));
#168072=CARTESIAN_POINT('Ctrl Pts',(68.7550615019874,-8.75625629838545,
55.735344761527));
#168073=CARTESIAN_POINT('Ctrl Pts',(68.719410575645,-8.74096463309731,55.7412035936562));
#168074=CARTESIAN_POINT('Ctrl Pts',(68.6450439249085,-8.7085157178352,55.7534134745602));
#168075=CARTESIAN_POINT('Ctrl Pts',(68.6063469642528,-8.69131612870886,
55.7597603922748));
#168076=CARTESIAN_POINT('Ctrl Pts',(68.5143005003488,-8.64965144430281,
55.7748418241645));
#168077=CARTESIAN_POINT('Ctrl Pts',(68.4610588711095,-8.62494388705857,
55.7835526017649));
#168078=CARTESIAN_POINT('Ctrl Pts',(68.2774377262581,-8.53761763459406,
55.8135509717747));
#168079=CARTESIAN_POINT('Ctrl Pts',(68.1482483613159,-8.47245687800116,
55.8345796874533));
#168080=CARTESIAN_POINT('Ctrl Pts',(67.8312326484309,-8.303217406328,55.8860012949317));
#168081=CARTESIAN_POINT('Ctrl Pts',(67.6453277735364,-8.19559664811225,
55.9159932278355));
#168082=CARTESIAN_POINT('Ctrl Pts',(67.2239787149258,-7.9319341052037,55.9836725900661));
#168083=CARTESIAN_POINT('Ctrl Pts',(66.9914862156297,-7.77142214123729,
56.0207889067569));
#168084=CARTESIAN_POINT('Ctrl Pts',(66.5006882927859,-7.39881576768811,
56.0989483301185));
#168085=CARTESIAN_POINT('Ctrl Pts',(66.2456699050642,-7.18290369070718,
56.1394305134399));
#168086=CARTESIAN_POINT('Ctrl Pts',(65.9535117858883,-6.90755300798338,
56.1860614781161));
#168087=CARTESIAN_POINT('Ctrl Pts',(65.9049799446759,-6.8608196681872,56.1938168845393));
#168088=CARTESIAN_POINT('Ctrl Pts',(65.8352781908649,-6.7922438347912,56.204973657854));
#168089=CARTESIAN_POINT('Ctrl Pts',(65.8137101651539,-6.77081769195838,
56.2084285426796));
#168090=CARTESIAN_POINT('Ctrl Pts',(65.7756635704857,-6.73265350446117,
56.2145282533942));
#168091=CARTESIAN_POINT('Ctrl Pts',(65.7591436431825,-6.71595806535549,
56.2171785472124));
#168092=CARTESIAN_POINT('Ctrl Pts',(65.7233028979491,-6.67946447995962,
56.2229324986162));
#168093=CARTESIAN_POINT('Ctrl Pts',(65.7040063823056,-6.65964256163827,
56.2260329095319));
#168094=CARTESIAN_POINT('Ctrl Pts',(65.6488963048328,-6.60253091306488,
56.2348940548648));
#168095=CARTESIAN_POINT('Ctrl Pts',(65.6132996938343,-6.56502872188158,
56.2406255726365));
#168096=CARTESIAN_POINT('Ctrl Pts',(65.5325701330007,-6.47856449704637,
56.2536386882547));
#168097=CARTESIAN_POINT('Ctrl Pts',(65.4876414162638,-6.42941125399487,
56.2608915979324));
#168098=CARTESIAN_POINT('Ctrl Pts',(65.3385176849451,-6.26275979422972,
56.2849897995331));
#168099=CARTESIAN_POINT('Ctrl Pts',(65.2367084334307,-6.14311162624957,
56.3014835051011));
#168100=CARTESIAN_POINT('Ctrl Pts',(64.9435887003916,-5.78073977715671,
56.3489748009083));
#168101=CARTESIAN_POINT('Ctrl Pts',(64.7610302256386,-5.5310248850314,56.3785531895552));
#168102=CARTESIAN_POINT('Ctrl Pts',(64.3563075352983,-4.91675613630517,
56.4435176420691));
#168103=CARTESIAN_POINT('Ctrl Pts',(64.145710531136,-4.54517280094908,56.4767839281));
#168104=CARTESIAN_POINT('Ctrl Pts',(63.925193946218,-4.08738129239885,56.5104471382329));
#168105=CARTESIAN_POINT('Ctrl Pts',(63.8909012843529,-4.01381963946874,
56.515642807749));
#168106=CARTESIAN_POINT('Ctrl Pts',(63.8381020056929,-3.89670771459341,
56.5235766947342));
#168107=CARTESIAN_POINT('Ctrl Pts',(63.8189810319182,-3.85344706253765,
56.5264354292444));
#168108=CARTESIAN_POINT('Ctrl Pts',(63.7852221324119,-3.77551868167044,
56.5314559495459));
#168109=CARTESIAN_POINT('Ctrl Pts',(63.7704675525215,-3.74090406713161,
56.5336406385959));
#168110=CARTESIAN_POINT('Ctrl Pts',(63.7363311990189,-3.65949861945083,
56.5386722921987));
#168111=CARTESIAN_POINT('Ctrl Pts',(63.7171143098185,-3.61263790917291,
56.5414869325814));
#168112=CARTESIAN_POINT('Ctrl Pts',(63.6621297106346,-3.4754831692157,56.5494869678141));
#168113=CARTESIAN_POINT('Ctrl Pts',(63.6273535235925,-3.38478746534386,
56.5544780988672));
#168114=CARTESIAN_POINT('Ctrl Pts',(63.477518677162,-2.97561215049119,56.5756642310369));
#168115=CARTESIAN_POINT('Ctrl Pts',(63.3778759563504,-2.65159817599759,
56.5888443814968));
#168116=CARTESIAN_POINT('Ctrl Pts',(63.1813227904579,-1.86765951736082,
56.612572443422));
#168117=CARTESIAN_POINT('Ctrl Pts',(63.1005088166986,-1.40452708149557,
56.620103561528));
#168118=CARTESIAN_POINT('Ctrl Pts',(63.0306375983541,-0.705469652835039,
56.6229891492765));
#168119=CARTESIAN_POINT('Ctrl Pts',(63.0158903312778,-0.472850780734742,
56.6225728925549));
#168120=CARTESIAN_POINT('Ctrl Pts',(63.0083792183321,-0.193782659307004,
56.6205773809409));
#168121=CARTESIAN_POINT('Ctrl Pts',(63.0074700259392,-0.147622185050712,
56.6201983997499));
#168122=CARTESIAN_POINT('Ctrl Pts',(63.006574086225,-0.0758064158346538,
56.6195343448282));
#168123=CARTESIAN_POINT('Ctrl Pts',(63.0063569701409,-0.0501543953342147,
56.6192823776814));
#168124=CARTESIAN_POINT('Ctrl Pts',(63.0061457093478,-0.00269292086676632,
56.6187891942779));
#168125=CARTESIAN_POINT('Ctrl Pts',(63.0061230385094,0.0191160765268714,
56.618552061429));
#168126=CARTESIAN_POINT('Ctrl Pts',(63.0062420791469,0.0693062479474148,
56.6179820379973));
#168127=CARTESIAN_POINT('Ctrl Pts',(63.006435382794,0.0976869089277555,
56.617641795673));
#168128=CARTESIAN_POINT('Ctrl Pts',(63.0074427319032,0.187235856074897,
56.6165108651902));
#168129=CARTESIAN_POINT('Ctrl Pts',(63.008715915933,0.248396566000516,56.6156539759828));
#168130=CARTESIAN_POINT('Ctrl Pts',(63.0184259441006,0.567997460409354,
56.6107209291361));
#168131=CARTESIAN_POINT('Ctrl Pts',(63.0367170380479,0.826006183880536,
56.6051794327142));
#168132=CARTESIAN_POINT('Ctrl Pts',(63.1334101599791,1.69300303724305,56.5806779675544));
#168133=CARTESIAN_POINT('Ctrl Pts',(63.25963213391,2.29486024221408,56.5537057007334));
#168134=CARTESIAN_POINT('Ctrl Pts',(63.500892638895,3.06905337443102,56.5035814234627));
#168135=CARTESIAN_POINT('Ctrl Pts',(63.5655845641365,3.25611292617718,56.4902301950731));
#168136=CARTESIAN_POINT('Ctrl Pts',(63.6603134830605,3.50488340961284,56.4707607076978));
#168137=CARTESIAN_POINT('Ctrl Pts',(63.6853302238838,3.56852787414792,56.465625807306));
#168138=CARTESIAN_POINT('Ctrl Pts',(63.7277513709704,3.67315314557332,56.4569287111113));
#168139=CARTESIAN_POINT('Ctrl Pts',(63.7447670543967,3.71429508499674,56.4534427487512));
#168140=CARTESIAN_POINT('Ctrl Pts',(63.7786185223381,3.79455747131133,56.4465125044715));
#168141=CARTESIAN_POINT('Ctrl Pts',(63.7954298849918,3.83368748356148,56.443073017419));
#168142=CARTESIAN_POINT('Ctrl Pts',(63.8359941654029,3.92639666985897,56.4347790344227));
#168143=CARTESIAN_POINT('Ctrl Pts',(63.8599773790326,3.97986909359566,56.429879367455));
#168144=CARTESIAN_POINT('Ctrl Pts',(63.9438512138028,4.16236946002337,56.412758319666));
#168145=CARTESIAN_POINT('Ctrl Pts',(64.0061080455079,4.29024477489271,56.4000732153486));
#168146=CARTESIAN_POINT('Ctrl Pts',(64.1667180715454,4.60225824568439,56.3674150360299));
#168147=CARTESIAN_POINT('Ctrl Pts',(64.2682717164075,4.78459800433314,56.3468202175828));
#168148=CARTESIAN_POINT('Ctrl Pts',(64.5246663128105,5.21136054059977,56.2950271687821));
#168149=CARTESIAN_POINT('Ctrl Pts',(64.6847764424568,5.45225071430965,56.2628362507192));
#168150=CARTESIAN_POINT('Ctrl Pts',(65.0562216874646,5.95917156752946,56.1887981878117));
#168151=CARTESIAN_POINT('Ctrl Pts',(65.2713472417803,6.22183166709789,56.1463001040846));
#168152=CARTESIAN_POINT('Ctrl Pts',(65.5454901724754,6.52186677953113,56.0930068462174));
#168153=CARTESIAN_POINT('Ctrl Pts',(65.59148852512,6.57113338955384,56.0840919239196));
#168154=CARTESIAN_POINT('Ctrl Pts',(65.6589636675872,6.64185876114554,56.0710583318046));
#168155=CARTESIAN_POINT('Ctrl Pts',(65.6800251815459,6.66372118754364,56.0669961133184));
#168156=CARTESIAN_POINT('Ctrl Pts',(65.7175278111001,6.70227325825661,56.0597740556079));
#168157=CARTESIAN_POINT('Ctrl Pts',(65.7339264651989,6.71900477355933,56.0566198703855));
#168158=CARTESIAN_POINT('Ctrl Pts',(65.769755424473,6.75528769292943,56.0497366972799));
#168159=CARTESIAN_POINT('Ctrl Pts',(65.78920917177,6.77481475013885,56.0460046078108));
#168160=CARTESIAN_POINT('Ctrl Pts',(65.8452184814091,6.83054100844442,56.0352736823481));
#168161=CARTESIAN_POINT('Ctrl Pts',(65.8819837963559,6.86652255685391,56.02824685625));
#168162=CARTESIAN_POINT('Ctrl Pts',(66.2045633178061,7.17706385419258,55.9667269602566));
#168163=CARTESIAN_POINT('Ctrl Pts',(66.5070134402033,7.4333039653498,55.9099347347465));
#168164=CARTESIAN_POINT('Ctrl Pts',(67.2468054604889,7.98344971704667,55.7714739233163));
#168165=CARTESIAN_POINT('Ctrl Pts',(67.694384990695,8.2608602358875,55.6879930552982));
#168166=CARTESIAN_POINT('Ctrl Pts',(68.2412859584078,8.53880768467192,55.5852861202919));
#168167=CARTESIAN_POINT('Ctrl Pts',(68.3207880524256,8.57779076856391,55.570341393945));
#168168=CARTESIAN_POINT('Ctrl Pts',(68.4488976763201,8.63834839773323,55.5462337554238));
#168169=CARTESIAN_POINT('Ctrl Pts',(68.4971652485335,8.66065843933449,55.5371450293802));
#168170=CARTESIAN_POINT('Ctrl Pts',(68.5834417130519,8.69963910682542,55.5208886229814));
#168171=CARTESIAN_POINT('Ctrl Pts',(68.621378167446,8.71647311521148,55.5137369203664));
#168172=CARTESIAN_POINT('Ctrl Pts',(68.7011587395927,8.75123510638607,55.4986890876233));
#168173=CARTESIAN_POINT('Ctrl Pts',(68.7430237709636,8.76911027582995,55.4907882610334));
#168174=CARTESIAN_POINT('Ctrl Pts',(68.8538854190036,8.8154810367184,55.4698544469925));
#168175=CARTESIAN_POINT('Ctrl Pts',(68.9230903630514,8.8434485186948,55.4567745383863));
#168176=CARTESIAN_POINT('Ctrl Pts',(69.2682526784094,8.97809914497562,55.3914786174327));
#168177=CARTESIAN_POINT('Ctrl Pts',(69.548710500393,9.07226064872847,55.3382288845659));
#168178=CARTESIAN_POINT('Ctrl Pts',(70.1668832416476,9.24722317947999,55.2205736727544));
#168179=CARTESIAN_POINT('Ctrl Pts',(70.505588672187,9.32271153541284,55.1559278539401));
#168180=CARTESIAN_POINT('Ctrl Pts',(71.2280333597365,9.44129039968847,55.018196396144));
#168181=CARTESIAN_POINT('Ctrl Pts',(71.6118780328604,9.4796880791591,54.9451078323308));
#168182=CARTESIAN_POINT('Ctrl Pts',(72.064452436974,9.49629949500186,54.8596882082981));
#168183=CARTESIAN_POINT('Ctrl Pts',(72.1318693912012,9.49802993185262,54.8469839017132));
#168184=CARTESIAN_POINT('Ctrl Pts',(72.2256162144575,9.49940219307597,54.8293506638683));
#168185=CARTESIAN_POINT('Ctrl Pts',(72.2519314844745,9.49967417411436,54.8244045025594));
#168186=CARTESIAN_POINT('Ctrl Pts',(72.2999330840384,9.49996379432037,54.8153891609369));
#168187=CARTESIAN_POINT('Ctrl Pts',(72.3216188479708,9.50001777310287,54.8113188710497));
#168188=CARTESIAN_POINT('Ctrl Pts',(72.366762842118,9.49997013945874,54.802851213075));
#168189=CARTESIAN_POINT('Ctrl Pts',(72.3902208756095,9.49985545870245,54.7984543078638));
#168190=CARTESIAN_POINT('Ctrl Pts',(72.4522682021779,9.49931425883601,54.7868321513294));
#168191=CARTESIAN_POINT('Ctrl Pts',(72.4908566582702,9.49873431089071,54.7796120959425));
#168192=CARTESIAN_POINT('Ctrl Pts',(72.6728524530838,9.49485114642883,54.7455942552908));
#168193=CARTESIAN_POINT('Ctrl Pts',(72.8161928622921,9.48843043562868,54.7189019812377));
#168194=CARTESIAN_POINT('Ctrl Pts',(73.2482509079764,9.45892269217232,54.6386418160273));
#168195=CARTESIAN_POINT('Ctrl Pts',(73.5361475678402,9.4255384738796,54.5854222547199));
#168196=CARTESIAN_POINT('Ctrl Pts',(74.4074689976157,9.28251837826274,54.4243855960287));
#168197=CARTESIAN_POINT('Ctrl Pts',(74.9825551345731,9.12996383677311,54.3180520805766));
#168198=CARTESIAN_POINT('Ctrl Pts',(75.6346424247745,8.88757546275032,54.1959999981996));
#168199=CARTESIAN_POINT('Ctrl Pts',(75.7293912938865,8.85056189003455,54.1782307582996));
#168200=CARTESIAN_POINT('Ctrl Pts',(75.8714788050035,8.79233028683736,54.1515276443941));
#168201=CARTESIAN_POINT('Ctrl Pts',(75.9192728784128,8.77227118345709,54.142535833178));
#168202=CARTESIAN_POINT('Ctrl Pts',(76.0047993741645,8.73552586772809,54.1264275362523));
#168203=CARTESIAN_POINT('Ctrl Pts',(76.0425924403916,8.71898778531994,54.1193032450804));
#168204=CARTESIAN_POINT('Ctrl Pts',(76.1230079048321,8.68315460977871,54.1041308926769));
#168205=CARTESIAN_POINT('Ctrl Pts',(76.1655977719933,8.66378751482831,54.0960871671847));
#168206=CARTESIAN_POINT('Ctrl Pts',(76.2811236426335,8.61019148723119,54.0742463352153));
#168207=CARTESIAN_POINT('Ctrl Pts',(76.3537681635725,8.57532826400436,54.0604883251766));
#168208=CARTESIAN_POINT('Ctrl Pts',(76.8430959574678,8.33257438134261,53.9676542582478));
#168209=CARTESIAN_POINT('Ctrl Pts',(77.2443395148981,8.09426590044972,53.890688505867));
#168210=CARTESIAN_POINT('Ctrl Pts',(78.0093841367439,7.55827125933498,53.7430263679308));
#168211=CARTESIAN_POINT('Ctrl Pts',(78.3720343067702,7.26119636107946,53.6725580848276));
#168212=CARTESIAN_POINT('Ctrl Pts',(78.7564490765101,6.89501641006542,53.5983289894072));
#168213=CARTESIAN_POINT('Ctrl Pts',(78.8009811114762,6.85174880886952,53.5897383474476));
#168214=CARTESIAN_POINT('Ctrl Pts',(78.8661819108371,6.787134839058,53.5771768078695));
#168215=CARTESIAN_POINT('Ctrl Pts',(78.8871756400428,6.76613262704809,53.5731347171465));
#168216=CARTESIAN_POINT('Ctrl Pts',(78.9244982501218,6.72844076320482,53.5659537884372));
#168217=CARTESIAN_POINT('Ctrl Pts',(78.9408641104192,6.71178988869277,53.5628067745242));
#168218=CARTESIAN_POINT('Ctrl Pts',(78.9770482353132,6.6747014325592,53.5558529342696));
#168219=CARTESIAN_POINT('Ctrl Pts',(78.9968366417043,6.65423413168898,53.552052677177));
#168220=CARTESIAN_POINT('Ctrl Pts',(79.0551614614934,6.59335986069459,53.5408588098267));
#168221=CARTESIAN_POINT('Ctrl Pts',(79.0934376842599,6.55269492202907,53.5335219884846));
#168222=CARTESIAN_POINT('Ctrl Pts',(79.1813467109718,6.4576246267802,53.5166883797742));
#168223=CARTESIAN_POINT('Ctrl Pts',(79.2307137207254,6.40296857267175,53.5072479025901));
#168224=CARTESIAN_POINT('Ctrl Pts',(79.4009217115848,6.21003926904902,53.4747280630421));
#168225=CARTESIAN_POINT('Ctrl Pts',(79.5184267884624,6.0687648685244,53.4523294721632));
#168226=CARTESIAN_POINT('Ctrl Pts',(80.0069152335273,5.44539984906099,53.3591640048695));
#168227=CARTESIAN_POINT('Ctrl Pts',(80.3356543188246,4.93090226056861,53.2962266732256));
#168228=CARTESIAN_POINT('Ctrl Pts',(80.6730303960008,4.27059756054935,53.2294276028492));
#168229=CARTESIAN_POINT('Ctrl Pts',(80.7304863243917,4.15214632014954,53.2179566607241));
#168230=CARTESIAN_POINT('Ctrl Pts',(80.8074861057222,3.98464594931615,53.202436251855));
#168231=CARTESIAN_POINT('Ctrl Pts',(80.8290950047086,3.93659324884282,53.1980630778914));
#168232=CARTESIAN_POINT('Ctrl Pts',(80.8660164081746,3.85263510295497,53.1905593473035));
#168233=CARTESIAN_POINT('Ctrl Pts',(80.8815080047392,3.81681236055175,53.1874007537807));
#168234=CARTESIAN_POINT('Ctrl Pts',(80.9135102763582,3.74154525083389,53.1808540485433));
#168235=CARTESIAN_POINT('Ctrl Pts',(80.9299767197412,3.7020824303408,53.1774728802268));
#168236=CARTESIAN_POINT('Ctrl Pts',(80.968741686554,3.60739333612914,53.1694821560375));
#168237=CARTESIAN_POINT('Ctrl Pts',(80.9907906994876,3.55206361323786,53.1649117173043));
#168238=CARTESIAN_POINT('Ctrl Pts',(81.0657476691169,3.35872375019643,53.1492835296927));
#168239=CARTESIAN_POINT('Ctrl Pts',(81.115978782651,3.21966537406848,53.1386459342224));
#168240=CARTESIAN_POINT('Ctrl Pts',(81.2317263970142,2.8743652716097,53.1137102932119));
#168241=CARTESIAN_POINT('Ctrl Pts',(81.2935211652247,2.66692257399266,53.1000034635478));
#168242=CARTESIAN_POINT('Ctrl Pts',(81.4318744016013,2.13757404759784,53.0682844376273));
#168243=CARTESIAN_POINT('Ctrl Pts',(81.4989227246745,1.81338860362256,53.0518329643473));
#168244=CARTESIAN_POINT('Ctrl Pts',(81.6072433598528,1.1081318123274,53.022821058296));
#168245=CARTESIAN_POINT('Ctrl Pts',(81.6427654782644,0.72671346380171,53.0112929320736));
#168246=CARTESIAN_POINT('Ctrl Pts',(81.6578886087804,0.276722274049013,
53.0031342417759));
#168247=CARTESIAN_POINT('Ctrl Pts',(81.6594498991434,0.209314703980056,
53.0020555649737));
#168248=CARTESIAN_POINT('Ctrl Pts',(81.6606569610688,0.114496078260597,
53.0007444782374));
#168249=CARTESIAN_POINT('Ctrl Pts',(81.6608896428737,0.0870961888499821,
53.0003898246238));
#168250=CARTESIAN_POINT('Ctrl Pts',(81.6610909333258,0.0397972357573462,
52.9998197807963));
#168251=CARTESIAN_POINT('Ctrl Pts',(81.6611144031703,0.0198986838339381,
52.9995928490222));
#168252=CARTESIAN_POINT('Ctrl Pts',(81.6610766756267,4.47259269587928E-12,
52.9993788854899));
#168253=CARTESIAN_POINT('Origin',(73.035119430904,-4.33680868994202E-16,
58.7874639765594));
#168254=CARTESIAN_POINT('',(82.5462364603111,-3.03519734642508E-8,56.9158101410025));
#168255=CARTESIAN_POINT('',(82.39079308452,-1.59709532818419E-15,57.1378062887238));
#168256=CARTESIAN_POINT('',(82.39079308452,-1.59709532818419E-15,57.1378062887238));
#168257=CARTESIAN_POINT('Ctrl Pts',(82.5462364601441,-3.03547367494313E-8,
56.915810141241));
#168258=CARTESIAN_POINT('Ctrl Pts',(82.5394791927201,1.22772898505908,56.9254605240026));
#168259=CARTESIAN_POINT('Ctrl Pts',(82.3004566029504,2.36750148144016,56.9793265804536));
#168260=CARTESIAN_POINT('Ctrl Pts',(81.6097765366974,4.21810104194341,57.1158850602721));
#168261=CARTESIAN_POINT('Ctrl Pts',(81.1769289619715,5.0196562288422,57.1971869538061));
#168262=CARTESIAN_POINT('Ctrl Pts',(80.3683710665038,6.11649038759656,57.34709448945));
#168263=CARTESIAN_POINT('Ctrl Pts',(80.069467258252,6.46633420673903,57.4023163122276));
#168264=CARTESIAN_POINT('Ctrl Pts',(78.8544190108279,7.69413928944279,57.6284971380434));
#168265=CARTESIAN_POINT('Ctrl Pts',(77.7887687197478,8.40501154231076,57.8292098024945));
#168266=CARTESIAN_POINT('Ctrl Pts',(75.7162159760365,9.25735872008406,58.2099244804492));
#168267=CARTESIAN_POINT('Ctrl Pts',(74.7560968307291,9.48744079427912,58.3836063847351));
#168268=CARTESIAN_POINT('Ctrl Pts',(72.3919766058581,9.66844304883471,58.8140516484161));
#168269=CARTESIAN_POINT('Ctrl Pts',(71.1462539173082,9.44699055352527,59.0467388176038));
#168270=CARTESIAN_POINT('Ctrl Pts',(69.304796347293,8.82095876131073,59.3871655574635));
#168271=CARTESIAN_POINT('Ctrl Pts',(68.5394038610483,8.43938374434001,59.5275098223593));
#168272=CARTESIAN_POINT('Ctrl Pts',(67.4999205036203,7.73139162193156,59.7177539829203));
#168273=CARTESIAN_POINT('Ctrl Pts',(67.1788228698108,7.48086138733766,59.7765194114987));
#168274=CARTESIAN_POINT('Ctrl Pts',(66.1091496978421,6.52721452808879,59.9736525925835));
#168275=CARTESIAN_POINT('Ctrl Pts',(65.4640288365233,5.72283346920203,60.0969323016118));
#168276=CARTESIAN_POINT('Ctrl Pts',(64.5534632021598,4.12018849825052,60.2726887746335));
#168277=CARTESIAN_POINT('Ctrl Pts',(64.2398628362638,3.35652371332293,60.3336831026002));
#168278=CARTESIAN_POINT('Ctrl Pts',(64.0263520775731,2.56296981511781,60.375952723877));
#168279=CARTESIAN_POINT('Origin',(73.035119430904,-4.33680868994202E-16,
58.7874639765594));
#168280=CARTESIAN_POINT('Origin',(72.2537026314029,-4.33680868994202E-16,
54.3558290880045));
#168281=CARTESIAN_POINT('',(62.5686102705547,3.28094194101619E-11,57.0166456920447));
#168282=CARTESIAN_POINT('',(62.5638890606905,-3.07089118677747E-11,56.9898703803749));
#168283=CARTESIAN_POINT('',(62.4056251012807,-1.65832766814156E-15,56.0923108646735));
#168284=CARTESIAN_POINT('',(76.6496952865773,-8.99107646638512,54.0790152794585));
#168285=CARTESIAN_POINT('Ctrl Pts',(62.5686102705547,6.5620497147992E-11,
57.0166456920447));
#168286=CARTESIAN_POINT('Ctrl Pts',(62.5685931686666,0.00949481003547198,
57.0165487024174));
#168287=CARTESIAN_POINT('Ctrl Pts',(62.5685893034143,0.0189896258170846,
57.0164489074448));
#168288=CARTESIAN_POINT('Ctrl Pts',(62.5686245154731,0.0546590393284597,
57.0160634979369));
#168289=CARTESIAN_POINT('Ctrl Pts',(62.5687509591852,0.0808332025605581,
57.0157594299316));
#168290=CARTESIAN_POINT('Ctrl Pts',(62.5694109838782,0.156908809992044,
57.0148143792232));
#168291=CARTESIAN_POINT('Ctrl Pts',(62.5702097450935,0.206806476872946,
57.0141178915667));
#168292=CARTESIAN_POINT('Ctrl Pts',(62.5812022844503,0.677655472505252,
57.0068335645316));
#168293=CARTESIAN_POINT('Ctrl Pts',(62.6170777414993,1.09751123819944,56.9949813703744));
#168294=CARTESIAN_POINT('Ctrl Pts',(62.7772610752319,2.17611177745555,56.952210362231));
#168295=CARTESIAN_POINT('Ctrl Pts',(62.9409331099227,2.82662380432915,56.914370342928));
#168296=CARTESIAN_POINT('Ctrl Pts',(63.2028308187524,3.55301820666139,56.8593144038791));
#168297=CARTESIAN_POINT('Ctrl Pts',(63.2395042796987,3.6500064231196,56.851683891133));
#168298=CARTESIAN_POINT('Ctrl Pts',(63.2970458462827,3.79534464003068,56.8398263299778));
#168299=CARTESIAN_POINT('Ctrl Pts',(63.3168090952313,3.84413840190321,56.8357725971545));
#168300=CARTESIAN_POINT('Ctrl Pts',(63.3529324808322,3.9313471081286,56.8283962528255));
#168301=CARTESIAN_POINT('Ctrl Pts',(63.369151024419,3.96982121447812,56.8250958401242));
#168302=CARTESIAN_POINT('Ctrl Pts',(63.4041974662658,4.05153158218341,56.8179877955404));
#168303=CARTESIAN_POINT('Ctrl Pts',(63.4230906979521,4.09473781598478,56.814169950057));
#168304=CARTESIAN_POINT('Ctrl Pts',(63.4750952395725,4.21141774879543,56.8036982139025));
#168305=CARTESIAN_POINT('Ctrl Pts',(63.5087853591859,4.28462135804108,56.7969536717606));
#168306=CARTESIAN_POINT('Ctrl Pts',(63.7140831478127,4.71690802153265,56.7560762678939));
#168307=CARTESIAN_POINT('Ctrl Pts',(63.9059480925585,5.06566528059715,56.7187809113607));
#168308=CARTESIAN_POINT('Ctrl Pts',(64.2775530262497,5.65507833823716,56.6475024582404));
#168309=CARTESIAN_POINT('Ctrl Pts',(64.4484320726923,5.90088720053665,56.6150003138333));
#168310=CARTESIAN_POINT('Ctrl Pts',(64.7263329313838,6.26462888920473,56.5622352149397));
#168311=CARTESIAN_POINT('Ctrl Pts',(64.8256734777039,6.38841120222158,56.5433883991211));
#168312=CARTESIAN_POINT('Ctrl Pts',(65.0416190896722,6.64470626388179,56.5023733078897));
#168313=CARTESIAN_POINT('Ctrl Pts',(65.1588690692999,6.77658307013366,56.480077510073));
#168314=CARTESIAN_POINT('Ctrl Pts',(65.3103902693084,6.93814801427767,56.4511627079599));
#168315=CARTESIAN_POINT('Ctrl Pts',(65.341503665052,6.97087418729542,56.4452201255802));
#168316=CARTESIAN_POINT('Ctrl Pts',(65.3910395910919,7.02227228460847,56.4357491367867));
#168317=CARTESIAN_POINT('Ctrl Pts',(65.4093179219078,7.04108811820308,56.4322523557138));
#168318=CARTESIAN_POINT('Ctrl Pts',(65.4442560166114,7.07676996905371,56.4255641409131));
#168319=CARTESIAN_POINT('Ctrl Pts',(65.4609022407199,7.09364932422797,56.4223756724639));
#168320=CARTESIAN_POINT('Ctrl Pts',(65.500890200341,7.13390812031383,56.4147120269516));
#168321=CARTESIAN_POINT('Ctrl Pts',(65.5242873191044,7.15722984841443,56.4102245973399));
#168322=CARTESIAN_POINT('Ctrl Pts',(65.6054669157639,7.23734412275618,56.3946444049743));
#168323=CARTESIAN_POINT('Ctrl Pts',(65.6638160395522,7.29353376969087,56.3834278350622));
#168324=CARTESIAN_POINT('Ctrl Pts',(65.8104477559555,7.43131412919587,56.3552091290267));
#168325=CARTESIAN_POINT('Ctrl Pts',(65.8995224735566,7.51200847800988,56.3380395757951));
#168326=CARTESIAN_POINT('Ctrl Pts',(66.3097465810958,7.87023483209404,56.2589171939135));
#168327=CARTESIAN_POINT('Ctrl Pts',(66.6467668404386,8.12820303385394,56.1937991707027));
#168328=CARTESIAN_POINT('Ctrl Pts',(67.3507618757592,8.59804670772538,56.0586588105352));
#168329=CARTESIAN_POINT('Ctrl Pts',(67.7169564898264,8.8095210453915,55.9887881688906));
#168330=CARTESIAN_POINT('Ctrl Pts',(68.1676576844471,9.03211541989052,55.9035840143207));
#168331=CARTESIAN_POINT('Ctrl Pts',(68.2402913230476,9.06687398848686,55.8898752203572));
#168332=CARTESIAN_POINT('Ctrl Pts',(68.3562224385685,9.12059472436967,55.8680306475622));
#168333=CARTESIAN_POINT('Ctrl Pts',(68.3992468473656,9.1401520682891,55.8599314749069));
#168334=CARTESIAN_POINT('Ctrl Pts',(68.480039378945,9.17616936533186,55.8447371902219));
#168335=CARTESIAN_POINT('Ctrl Pts',(68.5177735984549,9.19270466941119,55.8376465899271));
#168336=CARTESIAN_POINT('Ctrl Pts',(68.6025437256243,9.22921096226979,55.8217306694835));
#168337=CARTESIAN_POINT('Ctrl Pts',(68.6496331977045,9.24905145350947,55.8128984482855));
#168338=CARTESIAN_POINT('Ctrl Pts',(68.7904402123359,9.30707550747282,55.7865148074635));
#168339=CARTESIAN_POINT('Ctrl Pts',(68.884591039805,9.34416392126299,55.7689081535047));
#168340=CARTESIAN_POINT('Ctrl Pts',(69.3246383188335,9.50961615068189,55.6867707097593));
#168341=CARTESIAN_POINT('Ctrl Pts',(69.6769592990388,9.61962438373294,55.621458900797));
#168342=CARTESIAN_POINT('Ctrl Pts',(70.5371960288035,9.83528754798808,55.4625864613907));
#168343=CARTESIAN_POINT('Ctrl Pts',(71.048908636252,9.92074096312156,55.3685832667829));
#168344=CARTESIAN_POINT('Ctrl Pts',(71.7627018734177,9.9817681495456,55.2366069271219));
#168345=CARTESIAN_POINT('Ctrl Pts',(71.9611017592097,9.99258891067112,55.1998277628777));
#168346=CARTESIAN_POINT('Ctrl Pts',(72.203599699639,9.99833155165266,55.1546549956625));
#168347=CARTESIAN_POINT('Ctrl Pts',(72.2475490442521,9.9990724239228,55.1464592656265));
#168348=CARTESIAN_POINT('Ctrl Pts',(72.3164058741999,9.99976338670872,55.1336034720334));
#168349=CARTESIAN_POINT('Ctrl Pts',(72.3413119942273,9.99991702651808,55.1289502857122));
#168350=CARTESIAN_POINT('Ctrl Pts',(72.3855259707677,10.0000188413299,55.1206839567672));
#168351=CARTESIAN_POINT('Ctrl Pts',(72.4048336877748,10.0000054342108,55.1170721372491));
#168352=CARTESIAN_POINT('Ctrl Pts',(72.451123325768,9.99983454951726,55.1084081491416));
#168353=CARTESIAN_POINT('Ctrl Pts',(72.4781044759894,9.999621919639,55.1033542587867));
#168354=CARTESIAN_POINT('Ctrl Pts',(72.5603302356578,9.99862944185504,55.0879412849576));
#168355=CARTESIAN_POINT('Ctrl Pts',(72.6155674512234,9.99748873097646,55.07757194825));
#168356=CARTESIAN_POINT('Ctrl Pts',(73.1223786800342,9.98267180163953,54.9823072472566));
#168357=CARTESIAN_POINT('Ctrl Pts',(73.5723841650235,9.93780530720776,54.8968391548794));
#168358=CARTESIAN_POINT('Ctrl Pts',(74.6122274687567,9.7598650388144,54.6991641364504));
#168359=CARTESIAN_POINT('Ctrl Pts',(75.1962568126423,9.60265922768935,54.5880604160712));
#168360=CARTESIAN_POINT('Ctrl Pts',(75.8642685014173,9.35412961381878,54.4619437842037));
#168361=CARTESIAN_POINT('Ctrl Pts',(75.9653346411857,9.31459158333285,54.4428868311959));
#168362=CARTESIAN_POINT('Ctrl Pts',(76.114319610202,9.25341560240702,54.4148306996414));
#168363=CARTESIAN_POINT('Ctrl Pts',(76.1627401318286,9.23307411184802,54.4057181318169));
#168364=CARTESIAN_POINT('Ctrl Pts',(76.2489646345519,9.19602816007876,54.3895012115302));
#168365=CARTESIAN_POINT('Ctrl Pts',(76.2868291479776,9.17947383065478,54.3823832852544));
#168366=CARTESIAN_POINT('Ctrl Pts',(76.3669161884763,9.14385162252252,54.3673356218294));
#168367=CARTESIAN_POINT('Ctrl Pts',(76.4091113546987,9.12472220695442,54.359411926295));
#168368=CARTESIAN_POINT('Ctrl Pts',(76.5222538670056,9.07245359044907,54.3381768175924));
#168369=CARTESIAN_POINT('Ctrl Pts',(76.5929497175994,9.0387559043459,54.324920629335));
#168370=CARTESIAN_POINT('Ctrl Pts',(76.9868495342344,8.84515095815546,54.2511247644129));
#168371=CARTESIAN_POINT('Ctrl Pts',(77.3016797901881,8.66816136434575,54.1924003023509));
#168372=CARTESIAN_POINT('Ctrl Pts',(77.9709902958771,8.2416025614237,54.0677152862301));
#168373=CARTESIAN_POINT('Ctrl Pts',(78.3203102234116,7.98506816980612,54.0027534996117));
#168374=CARTESIAN_POINT('Ctrl Pts',(78.8273338068105,7.55846796156511,53.907693947408));
#168375=CARTESIAN_POINT('Ctrl Pts',(78.9976561830876,7.40469695446938,53.8756072407743));
#168376=CARTESIAN_POINT('Ctrl Pts',(79.196823627565,7.21184006112934,53.8377489170521));
#168377=CARTESIAN_POINT('Ctrl Pts',(79.2308806640514,7.17837944237662,53.8312627113588));
#168378=CARTESIAN_POINT('Ctrl Pts',(79.2838709764714,7.12555516319683,53.8211490058739));
#168379=CARTESIAN_POINT('Ctrl Pts',(79.3029677609928,7.10636076056874,53.8174997318882));
#168380=CARTESIAN_POINT('Ctrl Pts',(79.3368221267231,7.07205185340416,53.8110220008779));
#168381=CARTESIAN_POINT('Ctrl Pts',(79.3516101682565,7.05696863452912,53.8081895358175));
#168382=CARTESIAN_POINT('Ctrl Pts',(79.3872954209661,7.02033641678031,53.8013475080595));
#168383=CARTESIAN_POINT('Ctrl Pts',(79.4081435121506,6.99873873800463,53.7973444558431));
#168384=CARTESIAN_POINT('Ctrl Pts',(79.472887103537,6.93105197815689,53.7848957028617));
#168385=CARTESIAN_POINT('Ctrl Pts',(79.5164398444057,6.88462875973907,53.7764964389036));
#168386=CARTESIAN_POINT('Ctrl Pts',(79.7397312256811,6.64196310873446,53.7333162623742));
#168387=CARTESIAN_POINT('Ctrl Pts',(79.9120338929608,6.43883812475559,53.6995973295178));
#168388=CARTESIAN_POINT('Ctrl Pts',(80.4910429915452,5.69778386465837,53.5854046058007));
#168389=CARTESIAN_POINT('Ctrl Pts',(80.8516218033384,5.1249567220635,53.5127439344644));
#168390=CARTESIAN_POINT('Ctrl Pts',(81.2045052046764,4.4145165200458,53.4413396392349));
#168391=CARTESIAN_POINT('Ctrl Pts',(81.2547358913952,4.30880570084298,53.4311620728742));
#168392=CARTESIAN_POINT('Ctrl Pts',(81.3253878608425,4.15318401133537,53.416829086828));
#168393=CARTESIAN_POINT('Ctrl Pts',(81.3472580920879,4.10396827141044,53.4123896352064));
#168394=CARTESIAN_POINT('Ctrl Pts',(81.3854810065323,4.01606350294559,53.4046259712041));
#168395=CARTESIAN_POINT('Ctrl Pts',(81.4019872345779,3.97744534865631,53.4012716403612));
#168396=CARTESIAN_POINT('Ctrl Pts',(81.4360602604884,3.89633100871155,53.39434391029));
#168397=CARTESIAN_POINT('Ctrl Pts',(81.4535790343089,3.8538149174761,53.3907799353671));
#168398=CARTESIAN_POINT('Ctrl Pts',(81.4989448627626,3.74154699526084,53.3815451884075));
#168399=CARTESIAN_POINT('Ctrl Pts',(81.526308285344,3.6715951766271,53.3759692528103));
#168400=CARTESIAN_POINT('Ctrl Pts',(81.6549014398985,3.33174312405532,53.3497343074538));
#168401=CARTESIAN_POINT('Ctrl Pts',(81.7453916640756,3.05776684845851,53.3311807258126));
#168402=CARTESIAN_POINT('Ctrl Pts',(82.0082139313181,2.1308095937197,53.276714972163));
#168403=CARTESIAN_POINT('Ctrl Pts',(82.1271784738995,1.46408438971074,53.2510864460441));
#168404=CARTESIAN_POINT('Ctrl Pts',(82.1931395076163,0.603094753541315,
53.2321347455033));
#168405=CARTESIAN_POINT('Ctrl Pts',(82.2022677019319,0.415597777414796,
53.2288426076628));
#168406=CARTESIAN_POINT('Ctrl Pts',(82.2070769805183,0.184138117262164,
53.2257262275492));
#168407=CARTESIAN_POINT('Ctrl Pts',(82.2077021702983,0.140325651796728,
53.225178143409));
#168408=CARTESIAN_POINT('Ctrl Pts',(82.2082371524422,0.0713779561209165,
53.2243800307341));
#168409=CARTESIAN_POINT('Ctrl Pts',(82.2083383205992,0.046245093079615,
53.2241025670669));
#168410=CARTESIAN_POINT('Ctrl Pts',(82.2083513337792,0.00143950189477805,
53.2236316253277));
#168411=CARTESIAN_POINT('Ctrl Pts',(82.2082995334347,-0.0182328740553303,
53.2234329773184));
#168412=CARTESIAN_POINT('Ctrl Pts',(82.2080361066515,-0.0656420563921209,
53.2229738974244));
#168413=CARTESIAN_POINT('Ctrl Pts',(82.2077676701436,-0.0933783996608032,
53.2227215509783));
#168414=CARTESIAN_POINT('Ctrl Pts',(82.2065890355628,-0.178794268618658,
53.2219950719772));
#168415=CARTESIAN_POINT('Ctrl Pts',(82.2052988794444,-0.236467836561447,
53.2215756707227));
#168416=CARTESIAN_POINT('Ctrl Pts',(82.1944060681179,-0.588546837825432,
53.2194608974788));
#168417=CARTESIAN_POINT('Ctrl Pts',(82.1724294942745,-0.88243790565272,
53.2196020910157));
#168418=CARTESIAN_POINT('Ctrl Pts',(82.0822731726419,-1.64151812111276,
53.2254919879159));
#168419=CARTESIAN_POINT('Ctrl Pts',(81.9944941765417,-2.10363409194026,
53.2345433800741));
#168420=CARTESIAN_POINT('Ctrl Pts',(81.785379399967,-2.89923456200442,53.2608445865819));
#168421=CARTESIAN_POINT('Ctrl Pts',(81.6779400874776,-3.23560135778612,
53.2754738746009));
#168422=CARTESIAN_POINT('Ctrl Pts',(81.5246116259184,-3.64133935041874,
53.2976187432487));
#168423=CARTESIAN_POINT('Ctrl Pts',(81.4950606031747,-3.71678883849265,
53.3019329823102));
#168424=CARTESIAN_POINT('Ctrl Pts',(81.4466581165149,-3.83613447830237,
53.3090708071552));
#168425=CARTESIAN_POINT('Ctrl Pts',(81.4283931195386,-3.88027139020126,
53.3117794605117));
#168426=CARTESIAN_POINT('Ctrl Pts',(81.3935834438828,-3.96273216800703,
53.3169694548881));
#168427=CARTESIAN_POINT('Ctrl Pts',(81.3771123605242,-4.0010868763655,53.3194363769157));
#168428=CARTESIAN_POINT('Ctrl Pts',(81.3396269055438,-4.08690797437958,
53.3250751795106));
#168429=CARTESIAN_POINT('Ctrl Pts',(81.3184842492748,-4.13431534304264,
53.3282722461304));
#168430=CARTESIAN_POINT('Ctrl Pts',(81.2541380793106,-4.27566213026408,
53.3380506897363));
#168431=CARTESIAN_POINT('Ctrl Pts',(81.2098637021002,-4.3690916563408,53.3448420829308));
#168432=CARTESIAN_POINT('Ctrl Pts',(80.9912583899368,-4.81268285252289,
53.3786559820135));
#168433=CARTESIAN_POINT('Ctrl Pts',(80.7982406709098,-5.15296585623734,
53.4093446978793));
#168434=CARTESIAN_POINT('Ctrl Pts',(80.3613417059943,-5.82824181038578,
53.4797969457659));
#168435=CARTESIAN_POINT('Ctrl Pts',(80.1155533618687,-6.16106793349038,
53.5199203502594));
#168436=CARTESIAN_POINT('Ctrl Pts',(79.7283107431263,-6.62248904205124,
53.5829706910569));
#168437=CARTESIAN_POINT('Ctrl Pts',(79.6025159653024,-6.76398184540343,
53.6034272604744));
#168438=CARTESIAN_POINT('Ctrl Pts',(79.4411707345731,-6.93533705453489,
53.6295502026618));
#168439=CARTESIAN_POINT('Ctrl Pts',(79.4093138900537,-6.96870113621365,
53.6347027001072));
#168440=CARTESIAN_POINT('Ctrl Pts',(79.3588027252295,-7.02086859285705,
53.6428623218664));
#168441=CARTESIAN_POINT('Ctrl Pts',(79.3403022211868,-7.03982318528284,
53.6458488290259));
#168442=CARTESIAN_POINT('Ctrl Pts',(79.3051007124267,-7.07560071712405,
53.6515270435608));
#168443=CARTESIAN_POINT('Ctrl Pts',(79.2884148380019,-7.09243837342628,
53.654216721746));
#168444=CARTESIAN_POINT('Ctrl Pts',(79.2485560113145,-7.13237222496328,
53.6606375865655));
#168445=CARTESIAN_POINT('Ctrl Pts',(79.2253293412192,-7.15541328442209,
53.6643758686284));
#168446=CARTESIAN_POINT('Ctrl Pts',(79.1458234574229,-7.23350661259238,
53.6771621491895));
#168447=CARTESIAN_POINT('Ctrl Pts',(79.0890084007561,-7.28799729217439,
53.6862823131678));
#168448=CARTESIAN_POINT('Ctrl Pts',(78.9472362368661,-7.42076340791128,
53.70901044749));
#168449=CARTESIAN_POINT('Ctrl Pts',(78.8615564050088,-7.49823271888026,
53.722720614747));
#168450=CARTESIAN_POINT('Ctrl Pts',(78.4928148849061,-7.82010270632613,
53.7816783144235));
#168451=CARTESIAN_POINT('Ctrl Pts',(78.1975549213685,-8.04971976131072,
53.8287842325848));
#168452=CARTESIAN_POINT('Ctrl Pts',(77.4946396176575,-8.53511901737442,
53.9415857835965));
#168453=CARTESIAN_POINT('Ctrl Pts',(77.0800086819011,-8.77880988180894,
54.0086030220957));
#168454=CARTESIAN_POINT('Ctrl Pts',(76.6496952865772,-8.99107646638516,
54.0790152794585));
#168455=CARTESIAN_POINT('',(77.9145171600383,-8.24294705479842,53.8559930573772));
#168456=CARTESIAN_POINT('Origin',(72.3389200802052,-4.33680868994202E-16,
54.8391212561108));
#168457=CARTESIAN_POINT('Ctrl Pts',(77.9145171600384,-8.24294705479845,
53.8559930573776));
#168458=CARTESIAN_POINT('Ctrl Pts',(78.3213525049871,-7.95968552154139,
53.7882909406893));
#168459=CARTESIAN_POINT('Ctrl Pts',(78.7066406568712,-7.64588391010058,
53.7242405516931));
#168460=CARTESIAN_POINT('Ctrl Pts',(79.1153143825233,-7.25872586587658,
53.6576053048667));
#168461=CARTESIAN_POINT('Ctrl Pts',(79.1628447870651,-7.21279207225363,
53.6498776832898));
#168462=CARTESIAN_POINT('Ctrl Pts',(79.2316566723277,-7.1449561476965,53.638727453146));
#168463=CARTESIAN_POINT('Ctrl Pts',(79.2532933544652,-7.12342974689743,
53.6352269656706));
#168464=CARTESIAN_POINT('Ctrl Pts',(79.2913755032853,-7.08519266371684,
53.6290761688813));
#168465=CARTESIAN_POINT('Ctrl Pts',(79.3078606857158,-7.06852344330279,
53.626417065223));
#168466=CARTESIAN_POINT('Ctrl Pts',(79.3437537073191,-7.03197327270077,
53.6206351724958));
#168467=CARTESIAN_POINT('Ctrl Pts',(79.3631378764722,-7.01206882310716,
53.61751757868));
#168468=CARTESIAN_POINT('Ctrl Pts',(79.41767310297,-6.95560051615191,53.6087599817631));
#168469=CARTESIAN_POINT('Ctrl Pts',(79.4526324307376,-6.91884619202492,
53.6031618804814));
#168470=CARTESIAN_POINT('Ctrl Pts',(79.7280591780775,-6.6248273401461,53.559174211131));
#168471=CARTESIAN_POINT('Ctrl Pts',(79.9552681604661,-6.35506292800244,
53.523594164842));
#168472=CARTESIAN_POINT('Ctrl Pts',(80.4054397376295,-5.75936374378995,
53.4538920402273));
#168473=CARTESIAN_POINT('Ctrl Pts',(80.6244033749147,-5.43106846241846,
53.4204820818717));
#168474=CARTESIAN_POINT('Ctrl Pts',(80.9688584891665,-4.84215658921231,
53.3682552409087));
#168475=CARTESIAN_POINT('Ctrl Pts',(81.1034470810526,-4.58755226200957,
53.3479645477279));
#168476=CARTESIAN_POINT('Ctrl Pts',(81.2590761590207,-4.25980281262834,
53.3245849008017));
#168477=CARTESIAN_POINT('Ctrl Pts',(81.2904303026423,-4.19182407550534,
53.3198798723704));
#168478=CARTESIAN_POINT('Ctrl Pts',(81.3398082712556,-4.08154844968708,
53.3124782783543));
#168479=CARTESIAN_POINT('Ctrl Pts',(81.3583041848338,-4.03947115945202,
53.3097077474962));
#168480=CARTESIAN_POINT('Ctrl Pts',(81.3931809781168,-3.9586295611547,53.3044872579642));
#168481=CARTESIAN_POINT('Ctrl Pts',(81.4096081113492,-3.91988674847484,
53.3020300536218));
#168482=CARTESIAN_POINT('Ctrl Pts',(81.4465963369226,-3.83110678990619,
53.2965012025719));
#168483=CARTESIAN_POINT('Ctrl Pts',(81.4669986327005,-3.78100338387256,
53.2934544259837));
#168484=CARTESIAN_POINT('Ctrl Pts',(81.5305771698515,-3.62119512750036,
53.2839696316962));
#168485=CARTESIAN_POINT('Ctrl Pts',(81.572236572607,-3.51088379625024,53.2777694512274));
#168486=CARTESIAN_POINT('Ctrl Pts',(81.8651240172146,-2.69216385682614,
53.2343112982109));
#168487=CARTESIAN_POINT('Ctrl Pts',(82.0385197218235,-1.95789195221018,
53.2091171996664));
#168488=CARTESIAN_POINT('Ctrl Pts',(82.1557779714219,-0.992821857504143,
53.1961360517622));
#168489=CARTESIAN_POINT('Ctrl Pts',(82.1752039634383,-0.773882537922454,
53.1945149798879));
#168490=CARTESIAN_POINT('Ctrl Pts',(82.194423697907,-0.432031790683103,
53.1941895029693));
#168491=CARTESIAN_POINT('Ctrl Pts',(82.199097873528,-0.309465939716292,
53.1945131090541));
#168492=CARTESIAN_POINT('Ctrl Pts',(82.2023080731677,-0.149763588622181,
53.1955318282972));
#168493=CARTESIAN_POINT('Ctrl Pts',(82.2028513961955,-0.112675467650475,
53.1958103295903));
#168494=CARTESIAN_POINT('Ctrl Pts',(82.2034079333408,-0.0521905018019316,
53.1963337441948));
#168495=CARTESIAN_POINT('Ctrl Pts',(82.2035428066805,-0.0287949156210848,
53.1965530888186));
#168496=CARTESIAN_POINT('Ctrl Pts',(82.2036492377446,0.0168896857020898,
53.1970146422514));
#168497=CARTESIAN_POINT('Ctrl Pts',(82.2036282217056,0.03917850045416,53.1972552920767));
#168498=CARTESIAN_POINT('Ctrl Pts',(82.2034176645911,0.089117039237505,
53.1978288885152));
#168499=CARTESIAN_POINT('Ctrl Pts',(82.2031887983291,0.11676636883879,53.1981701078976));
#168500=CARTESIAN_POINT('Ctrl Pts',(82.2019882750365,0.214051685765103,
53.199453157529));
#168501=CARTESIAN_POINT('Ctrl Pts',(82.2004164388026,0.283676631147189,
53.2005200694232));
#168502=CARTESIAN_POINT('Ctrl Pts',(82.1854431741609,0.739836407447927,
53.2084635920051));
#168503=CARTESIAN_POINT('Ctrl Pts',(82.1507781497542,1.12527542774975,53.2196531721575));
#168504=CARTESIAN_POINT('Ctrl Pts',(82.0472356809411,1.82541293831156,53.2473373839046));
#168505=CARTESIAN_POINT('Ctrl Pts',(81.9851889410471,2.14065632040254,53.262601494305));
#168506=CARTESIAN_POINT('Ctrl Pts',(81.8147773529143,2.83107629400283,53.3018785874066));
#168507=CARTESIAN_POINT('Ctrl Pts',(81.6994566408859,3.20393279213455,53.327027734262));
#168508=CARTESIAN_POINT('Ctrl Pts',(81.534409024631,3.645013793902,53.361444931191));
#168509=CARTESIAN_POINT('Ctrl Pts',(81.5050244062944,3.72073359133889,53.3675253981988));
#168510=CARTESIAN_POINT('Ctrl Pts',(81.4570803095161,3.83997159893516,53.3773740258539));
#168511=CARTESIAN_POINT('Ctrl Pts',(81.4391230893453,3.88373578376918,53.3810477506789));
#168512=CARTESIAN_POINT('Ctrl Pts',(81.4047440391612,3.96586499924193,53.388053381821));
#168513=CARTESIAN_POINT('Ctrl Pts',(81.3883905835414,4.00425844883778,53.3913745616527));
#168514=CARTESIAN_POINT('Ctrl Pts',(81.3509570056587,4.09064416497588,53.398951955667));
#168515=CARTESIAN_POINT('Ctrl Pts',(81.3297400306502,4.13857388585655,53.4032295829852));
#168516=CARTESIAN_POINT('Ctrl Pts',(81.2643845016779,4.28314263220271,53.416355706068));
#168517=CARTESIAN_POINT('Ctrl Pts',(81.2190916104298,4.37923486845521,53.4253850558867));
#168518=CARTESIAN_POINT('Ctrl Pts',(80.9515672387241,4.92418214483371,53.4783601702573));
#168519=CARTESIAN_POINT('Ctrl Pts',(80.6976545542606,5.356188667899,53.527248938));
#168520=CARTESIAN_POINT('Ctrl Pts',(80.3075667002764,5.91868773389435,53.6015669614577));
#168521=CARTESIAN_POINT('Ctrl Pts',(80.1981682730969,6.06744525204309,53.6223445870643));
#168522=CARTESIAN_POINT('Ctrl Pts',(79.9024844656567,6.44698191690618,53.6784726869544));
#168523=CARTESIAN_POINT('Ctrl Pts',(79.7099997632217,6.67252150865751,53.7149802152015));
#168524=CARTESIAN_POINT('Ctrl Pts',(79.4742736725412,6.92500277122591,53.7599509479243));
#168525=CARTESIAN_POINT('Ctrl Pts',(79.440355264385,6.9607946606352,53.7664277800239));
#168526=CARTESIAN_POINT('Ctrl Pts',(79.3873681495772,7.0158821806866,53.7765571260367));
#168527=CARTESIAN_POINT('Ctrl Pts',(79.3684806038538,7.03535822530672,53.7801699742222));
#168528=CARTESIAN_POINT('Ctrl Pts',(79.3331054726813,7.07153807419901,53.7869410716904));
#168529=CARTESIAN_POINT('Ctrl Pts',(79.3166377119049,7.08826153616138,53.7900949671569));
#168530=CARTESIAN_POINT('Ctrl Pts',(79.2784323070172,7.12678621626691,53.7974161046985));
#168531=CARTESIAN_POINT('Ctrl Pts',(79.2566531709839,7.14854412365631,53.801592526273));
#168532=CARTESIAN_POINT('Ctrl Pts',(79.1852675547447,7.21919989637126,53.8152903251426));
#168533=CARTESIAN_POINT('Ctrl Pts',(79.135256140556,7.26766846322225,53.8249003507436));
#168534=CARTESIAN_POINT('Ctrl Pts',(78.8156881144894,7.57091353084329,53.8863716156883));
#168535=CARTESIAN_POINT('Ctrl Pts',(78.5328018589116,7.81063953083945,53.9410611683261));
#168536=CARTESIAN_POINT('Ctrl Pts',(77.9736667631488,8.23267027361622,54.0488349431247));
#168537=CARTESIAN_POINT('Ctrl Pts',(77.700321763642,8.41811447270732,54.101392894075));
#168538=CARTESIAN_POINT('Ctrl Pts',(77.250526983879,8.69111022486983,54.1873553235274));
#168539=CARTESIAN_POINT('Ctrl Pts',(77.0797732891893,8.7878289353557,54.2198784292574));
#168540=CARTESIAN_POINT('Ctrl Pts',(76.785694745722,8.94287577886063,54.2756668084484));
#168541=CARTESIAN_POINT('Ctrl Pts',(76.6638197830142,9.00389919819087,54.2987246169373));
#168542=CARTESIAN_POINT('Ctrl Pts',(76.4889155403398,9.08692943818848,54.3317219233844));
#168543=CARTESIAN_POINT('Ctrl Pts',(76.4368897146813,9.11106585925497,54.3415256087708));
#168544=CARTESIAN_POINT('Ctrl Pts',(76.3463917995033,9.15208231039055,54.3585589846606));
#168545=CARTESIAN_POINT('Ctrl Pts',(76.3080161228249,9.16917655127408,54.3657758426482));
#168546=CARTESIAN_POINT('Ctrl Pts',(76.2338986411413,9.20161794471294,54.3797024288626));
#168547=CARTESIAN_POINT('Ctrl Pts',(76.1981727962142,9.21700046941069,54.3864100301935));
#168548=CARTESIAN_POINT('Ctrl Pts',(76.1036783887938,9.25701661837335,54.4041378260982));
#168549=CARTESIAN_POINT('Ctrl Pts',(76.0447613359343,9.28128620366111,54.415177129959));
#168550=CARTESIAN_POINT('Ctrl Pts',(75.8317856267572,9.36657683651875,54.4550333811033));
#168551=CARTESIAN_POINT('Ctrl Pts',(75.6764373842164,9.42422345570597,54.4840128765064));
#168552=CARTESIAN_POINT('Ctrl Pts',(74.8861778054217,9.69467707166735,54.6310206618911));
#168553=CARTESIAN_POINT('Ctrl Pts',(74.2322948513584,9.8452152704738,54.7511907050721));
#168554=CARTESIAN_POINT('Ctrl Pts',(73.3553891374439,9.95344756785505,54.9129267442595));
#168555=CARTESIAN_POINT('Ctrl Pts',(73.1414358637586,9.97265178972028,54.9524469832369));
#168556=CARTESIAN_POINT('Ctrl Pts',(72.8071601079025,9.99146775348171,55.0144367613227));
#168557=CARTESIAN_POINT('Ctrl Pts',(72.6871530679604,9.99598246383561,55.0367406512944));
#168558=CARTESIAN_POINT('Ctrl Pts',(72.5307022724023,9.99895120171713,55.0659064767255));
#168559=CARTESIAN_POINT('Ctrl Pts',(72.4942950130809,9.99943627525533,55.0726998440897));
#168560=CARTESIAN_POINT('Ctrl Pts',(72.4349003857445,9.99989195619382,55.0837936189728));
#168561=CARTESIAN_POINT('Ctrl Pts',(72.4119135490329,9.99998629424917,55.0880898326846));
#168562=CARTESIAN_POINT('Ctrl Pts',(72.3670090019568,10.0000103582077,55.0964880155532));
#168563=CARTESIAN_POINT('Ctrl Pts',(72.3450914454647,9.9999475308271,55.100589712496));
#168564=CARTESIAN_POINT('Ctrl Pts',(72.2959657850777,9.99963955696024,55.1097887977387));
#168565=CARTESIAN_POINT('Ctrl Pts',(72.2687583024436,9.99935404929783,55.1148874216539));
#168566=CARTESIAN_POINT('Ctrl Pts',(72.1729253539559,9.99794349796811,55.1328591367949));
#168567=CARTESIAN_POINT('Ctrl Pts',(72.1043141550645,9.99620210960415,55.1457490745891));
#168568=CARTESIAN_POINT('Ctrl Pts',(71.645274960245,9.97965440789786,55.2321211755954));
#168569=CARTESIAN_POINT('Ctrl Pts',(71.2561008595327,9.94190193294541,55.3059772517661));
#168570=CARTESIAN_POINT('Ctrl Pts',(70.4847514458789,9.81952100541946,55.4525715979359));
#168571=CARTESIAN_POINT('Ctrl Pts',(70.1032452753374,9.73505714580995,55.5251789894049));
#168572=CARTESIAN_POINT('Ctrl Pts',(69.4320850895938,9.54327503097831,55.652511085974));
#168573=CARTESIAN_POINT('Ctrl Pts',(69.1405515740728,9.44476816389429,55.7076831163667));
#168574=CARTESIAN_POINT('Ctrl Pts',(68.7833624712188,9.30486945645273,55.7750318353828));
#168575=CARTESIAN_POINT('Ctrl Pts',(68.7130477992302,9.27637724207569,55.7882779236005));
#168576=CARTESIAN_POINT('Ctrl Pts',(68.6008143123456,9.22936499221988,55.8094016020938));
#168577=CARTESIAN_POINT('Ctrl Pts',(68.5586882449006,9.21136904367418,55.817325852638));
#168578=CARTESIAN_POINT('Ctrl Pts',(68.4787057422203,9.17653225900244,55.8323629426998));
#168579=CARTESIAN_POINT('Ctrl Pts',(68.4408274936767,9.15974614989543,55.8394806768922));
#168580=CARTESIAN_POINT('Ctrl Pts',(68.3543291058352,9.12075216394802,55.8557266595136));
#168581=CARTESIAN_POINT('Ctrl Pts',(68.3057797977727,9.09838394398872,55.8648392750116));
#168582=CARTESIAN_POINT('Ctrl Pts',(68.1784093339627,9.03842665574957,55.8887316524423));
#168583=CARTESIAN_POINT('Ctrl Pts',(68.0998943524999,9.00017211488093,55.9034445281792));
#168584=CARTESIAN_POINT('Ctrl Pts',(67.4174763785686,8.6562795829925,56.0312022940559));
#168585=CARTESIAN_POINT('Ctrl Pts',(66.8453167095885,8.28921705592231,56.1373274536897));
#168586=CARTESIAN_POINT('Ctrl Pts',(66.0921755905048,7.68770791482057,56.27811528857));
#168587=CARTESIAN_POINT('Ctrl Pts',(65.8772541971612,7.500227094911,56.3184617932426));
#168588=CARTESIAN_POINT('Ctrl Pts',(65.6230393573239,7.25825490948418,56.3666777561398));
#168589=CARTESIAN_POINT('Ctrl Pts',(65.5758733348315,7.21245257664757,56.375645869119));
#168590=CARTESIAN_POINT('Ctrl Pts',(65.5075619195612,7.14477532374694,56.3886719304733));
#168591=CARTESIAN_POINT('Ctrl Pts',(65.4860585427239,7.12327357177135,56.3927778538137));
#168592=CARTESIAN_POINT('Ctrl Pts',(65.4481971095436,7.08506308867001,56.4000175881125));
#168593=CARTESIAN_POINT('Ctrl Pts',(65.4317989422668,7.06839559957553,56.4031566899719));
#168594=CARTESIAN_POINT('Ctrl Pts',(65.3960775986516,7.03182834483428,56.4100026170094));
#168595=CARTESIAN_POINT('Ctrl Pts',(65.3767786109534,7.01190491220764,56.4137062061511));
#168596=CARTESIAN_POINT('Ctrl Pts',(65.3224396491735,6.95533235989226,56.4241476894208));
#168597=CARTESIAN_POINT('Ctrl Pts',(65.2875953067392,6.91849167356383,56.4308592284819));
#168598=CARTESIAN_POINT('Ctrl Pts',(65.0075613497781,6.61780879386758,56.4849184093134));
#168599=CARTESIAN_POINT('Ctrl Pts',(64.7765038215339,6.34081331571827,56.5302699266778));
#168600=CARTESIAN_POINT('Ctrl Pts',(64.404975324249,5.8426753477537,56.6038621944375));
#168601=CARTESIAN_POINT('Ctrl Pts',(64.2573004463,5.62755015863068,56.6333328284688));
#168602=CARTESIAN_POINT('Ctrl Pts',(63.905344448837,5.06920505870918,56.7038769641504));
#168603=CARTESIAN_POINT('Ctrl Pts',(63.712735334331,4.71890369121622,56.7427704946597));
#168604=CARTESIAN_POINT('Ctrl Pts',(63.5067271573156,4.28490486719319,56.7845103748413));
#168605=CARTESIAN_POINT('Ctrl Pts',(63.4730211685367,4.21163965241819,56.7913457848994));
#168606=CARTESIAN_POINT('Ctrl Pts',(63.4209947451818,4.09488400238202,56.8019058025251));
#168607=CARTESIAN_POINT('Ctrl Pts',(63.4020981755873,4.05166448965373,56.8057433879861));
#168608=CARTESIAN_POINT('Ctrl Pts',(63.3670479653965,3.96994297956643,56.8128654431831));
#168609=CARTESIAN_POINT('Ctrl Pts',(63.3508292279652,3.93147113120173,56.8161626817023));
#168610=CARTESIAN_POINT('Ctrl Pts',(63.3147095875646,3.84428658170562,56.8235095826429));
#168611=CARTESIAN_POINT('Ctrl Pts',(63.2949489908331,3.79551479842813,56.8275317193774));
#168612=CARTESIAN_POINT('Ctrl Pts',(63.2361204593854,3.64699491858422,56.8395146673658));
#168613=CARTESIAN_POINT('Ctrl Pts',(63.1982501354834,3.54676204119937,56.8472407375714));
#168614=CARTESIAN_POINT('Ctrl Pts',(62.9432194224137,2.83789119790707,56.89937257243));
#168615=CARTESIAN_POINT('Ctrl Pts',(62.7829543507186,2.20960977442238,56.9325536750684));
#168616=CARTESIAN_POINT('Ctrl Pts',(62.6675377370273,1.46603257831083,56.9587000277526));
#168617=CARTESIAN_POINT('Ctrl Pts',(62.653025353269,1.36186430567599,56.9620734877445));
#168618=CARTESIAN_POINT('Ctrl Pts',(62.6008696196287,0.939452770540981,
56.9746222950362));
#168619=CARTESIAN_POINT('Ctrl Pts',(62.576706760898,0.61967254587812,56.9815288742265));
#168620=CARTESIAN_POINT('Ctrl Pts',(62.5661492407005,0.240484801933824,
56.9870292662832));
#168621=CARTESIAN_POINT('Ctrl Pts',(62.5650259598434,0.181705807685922,
56.9878057787459));
#168622=CARTESIAN_POINT('Ctrl Pts',(62.5641260848524,0.0949716285669506,
56.988842406409));
#168623=CARTESIAN_POINT('Ctrl Pts',(62.5639521579111,0.0670225197836035,
56.9891597235968));
#168624=CARTESIAN_POINT('Ctrl Pts',(62.5638673523048,0.0260486050623847,
56.9896007351212));
#168625=CARTESIAN_POINT('Ctrl Pts',(62.5638656015227,0.0130243126943486,
56.9897373368234));
#168626=CARTESIAN_POINT('Ctrl Pts',(62.5638890606905,-6.14161654078813E-11,
56.9898703803749));
#168627=CARTESIAN_POINT('Origin',(72.2537026314029,-4.33680868994202E-16,
54.3558290880045));
#168628=CARTESIAN_POINT('',(62.6814815860384,9.62546012605022E-15,57.6567707315034));
#168629=CARTESIAN_POINT('',(62.6767603761739,-1.97855053433324E-11,57.6299954198325));
#168630=CARTESIAN_POINT('',(62.4056251012807,-1.65832766814156E-15,56.0923108646735));
#168631=CARTESIAN_POINT('Ctrl Pts',(62.6814815860384,1.02164152390125E-14,
57.6567707315033));
#168632=CARTESIAN_POINT('Ctrl Pts',(62.6814467800136,0.0193239827663985,
57.6565733367276));
#168633=CARTESIAN_POINT('Ctrl Pts',(62.6814667819337,0.0386379061186494,
57.6563644329446));
#168634=CARTESIAN_POINT('Ctrl Pts',(62.6816358108951,0.0822795851394926,
57.6558663163279));
#168635=CARTESIAN_POINT('Ctrl Pts',(62.6818168480097,0.106597020978416,
57.6555704717971));
#168636=CARTESIAN_POINT('Ctrl Pts',(62.6827503906637,0.191328778297451,
57.6544763814131));
#168637=CARTESIAN_POINT('Ctrl Pts',(62.6839522664629,0.25173563754625,57.6535843353215));
#168638=CARTESIAN_POINT('Ctrl Pts',(62.6983697979476,0.752610954394169,
57.6452757657968));
#168639=CARTESIAN_POINT('Ctrl Pts',(62.7395768586216,1.19170326118966,57.6321602557347));
#168640=CARTESIAN_POINT('Ctrl Pts',(62.8721327213917,2.02001406534445,57.597587283528));
#168641=CARTESIAN_POINT('Ctrl Pts',(62.958223972576,2.40926975985943,57.5770725453641));
#168642=CARTESIAN_POINT('Ctrl Pts',(63.1185718279245,2.97360922428409,57.5414229492147));
#168643=CARTESIAN_POINT('Ctrl Pts',(63.1751777127269,3.15347783855469,57.5291430864392));
#168644=CARTESIAN_POINT('Ctrl Pts',(63.2806723227062,3.45850066534843,57.5067595373642));
#168645=CARTESIAN_POINT('Ctrl Pts',(63.3270884274095,3.58448352257791,57.4970475776677));
#168646=CARTESIAN_POINT('Ctrl Pts',(63.396953821441,3.76300576530805,57.4826159410961));
#168647=CARTESIAN_POINT('Ctrl Pts',(63.4183615824116,3.81635388271896,57.4782166045481));
#168648=CARTESIAN_POINT('Ctrl Pts',(63.4563555472384,3.90873254769104,57.4704473416695));
#168649=CARTESIAN_POINT('Ctrl Pts',(63.4727342466018,3.94784951390339,57.4671099446272));
#168650=CARTESIAN_POINT('Ctrl Pts',(63.5048385716458,4.02318046549636,57.4605906168753));
#168651=CARTESIAN_POINT('Ctrl Pts',(63.5205311644477,4.05940811246652,57.4574138738473));
#168652=CARTESIAN_POINT('Ctrl Pts',(63.5626945743402,4.15519228201309,57.4489042030205));
#168653=CARTESIAN_POINT('Ctrl Pts',(63.5895306704828,4.21458079301957,57.4435140775963));
#168654=CARTESIAN_POINT('Ctrl Pts',(63.689980181044,4.43122553157555,57.4234303374262));
#168655=CARTESIAN_POINT('Ctrl Pts',(63.7670758267679,4.58678145308591,57.4081909112725));
#168656=CARTESIAN_POINT('Ctrl Pts',(64.131180340086,5.27584275154966,57.3368970300171));
#168657=CARTESIAN_POINT('Ctrl Pts',(64.4619130310351,5.78405141775196,57.2739778488605));
#168658=CARTESIAN_POINT('Ctrl Pts',(64.9943877287862,6.45942005174256,57.1729082461595));
#168659=CARTESIAN_POINT('Ctrl Pts',(65.1603691071588,6.65403590688992,57.1414140701367));
#168660=CARTESIAN_POINT('Ctrl Pts',(65.3758470383112,6.88783488184467,57.1003384048787));
#168661=CARTESIAN_POINT('Ctrl Pts',(65.4185970285261,6.93335197496354,57.0921802957506));
#168662=CARTESIAN_POINT('Ctrl Pts',(65.4823633296937,6.99997734498814,57.0799947906232));
#168663=CARTESIAN_POINT('Ctrl Pts',(65.503056940761,7.02140516208031,57.0760377535803));
#168664=CARTESIAN_POINT('Ctrl Pts',(65.5385697534532,7.05784878325061,57.0692421329395));
#168665=CARTESIAN_POINT('Ctrl Pts',(65.5533419502679,7.07291192194743,57.0664139352711));
#168666=CARTESIAN_POINT('Ctrl Pts',(65.5872939540203,7.10731283037035,57.0599103117759));
#168667=CARTESIAN_POINT('Ctrl Pts',(65.6065047626977,7.12661822762156,57.056228017566));
#168668=CARTESIAN_POINT('Ctrl Pts',(65.6601141629369,7.18005022526594,57.0459461950387));
#168669=CARTESIAN_POINT('Ctrl Pts',(65.6946799705971,7.21400088796866,57.0393098887401));
#168670=CARTESIAN_POINT('Ctrl Pts',(65.9060084709376,7.41854867042736,56.9987022317964));
#168671=CARTESIAN_POINT('Ctrl Pts',(66.0886844941911,7.58265997151768,56.9634565764544));
#168672=CARTESIAN_POINT('Ctrl Pts',(66.6180849498278,8.02372293234134,56.8613030623954));
#168673=CARTESIAN_POINT('Ctrl Pts',(66.9773936236622,8.28408060060196,56.7919794088639));
#168674=CARTESIAN_POINT('Ctrl Pts',(67.5417517737355,8.63728005446337,56.6839593586341));
#168675=CARTESIAN_POINT('Ctrl Pts',(67.7346571205685,8.74901195980444,56.6471710870525));
#168676=CARTESIAN_POINT('Ctrl Pts',(68.0628420757879,8.9243694772397,56.584867931222));
#168677=CARTESIAN_POINT('Ctrl Pts',(68.1961067401817,8.99168665148801,56.5596432026462));
#168678=CARTESIAN_POINT('Ctrl Pts',(68.3844413331462,9.08144787319946,56.5241048839485));
#168679=CARTESIAN_POINT('Ctrl Pts',(68.4382747804767,9.10650320417762,56.5139589210525));
#168680=CARTESIAN_POINT('Ctrl Pts',(68.5309071191952,9.14858921091658,56.4965217049131));
#168681=CARTESIAN_POINT('Ctrl Pts',(68.5695964083469,9.16586300794149,56.4892450483959));
#168682=CARTESIAN_POINT('Ctrl Pts',(68.6436243857457,9.19833617415454,56.4753338204177));
#168683=CARTESIAN_POINT('Ctrl Pts',(68.6789432314978,9.21357990657319,56.4687018850815));
#168684=CARTESIAN_POINT('Ctrl Pts',(68.7618213270094,9.24876839856928,56.4531515140686));
#168685=CARTESIAN_POINT('Ctrl Pts',(68.8094492540546,9.26854449865722,56.4442242470775));
#168686=CARTESIAN_POINT('Ctrl Pts',(68.9505298397407,9.3258120072773,56.4178069543346));
#168687=CARTESIAN_POINT('Ctrl Pts',(69.0444016918334,9.36222751951755,56.4002636867578));
#168688=CARTESIAN_POINT('Ctrl Pts',(69.6558047166414,9.58853688578623,56.2862105400082));
#168689=CARTESIAN_POINT('Ctrl Pts',(70.1878539477727,9.73541835626262,56.1879955390148));
#168690=CARTESIAN_POINT('Ctrl Pts',(71.0320428635474,9.89268614298055,56.0324454695225));
#168691=CARTESIAN_POINT('Ctrl Pts',(71.3373159597415,9.93461146318714,55.976235148332));
#168692=CARTESIAN_POINT('Ctrl Pts',(71.8549439080666,9.98068700579617,55.8805567207322));
#168693=CARTESIAN_POINT('Ctrl Pts',(72.0664301929503,9.99253060617768,55.8413614375923));
#168694=CARTESIAN_POINT('Ctrl Pts',(72.3215090850681,9.99842424619325,55.7938407554123));
#168695=CARTESIAN_POINT('Ctrl Pts',(72.3649323706168,9.99913479020319,55.7857424549098));
#168696=CARTESIAN_POINT('Ctrl Pts',(72.432887762073,9.99978867791876,55.773054049421));
#168697=CARTESIAN_POINT('Ctrl Pts',(72.4574186235897,9.99993131373539,55.7684706799752));
#168698=CARTESIAN_POINT('Ctrl Pts',(72.503480422669,10.0000237508442,55.7598584095973));
#168699=CARTESIAN_POINT('Ctrl Pts',(72.5250111295909,9.99999499713105,55.7558302577256));
#168700=CARTESIAN_POINT('Ctrl Pts',(72.5748484602827,9.99976186526923,55.7465005807097));
#168701=CARTESIAN_POINT('Ctrl Pts',(72.6031543088402,9.9995050533136,55.7411974382303));
#168702=CARTESIAN_POINT('Ctrl Pts',(72.6953785541948,9.99826296194707,55.7239061389232));
#168703=CARTESIAN_POINT('Ctrl Pts',(72.7592857387396,9.99676768883518,55.7119037916169));
#168704=CARTESIAN_POINT('Ctrl Pts',(73.3631586405893,9.97663930622508,55.5983249562949));
#168705=CARTESIAN_POINT('Ctrl Pts',(73.9005638115575,9.91336745251767,55.4960442035739));
#168706=CARTESIAN_POINT('Ctrl Pts',(74.8768633421158,9.71444707239684,55.3104137122434));
#168707=CARTESIAN_POINT('Ctrl Pts',(75.3168347738604,9.59191334476979,55.2268252740692));
#168708=CARTESIAN_POINT('Ctrl Pts',(75.8784107693279,9.39192944166182,55.1206954970908));
#168709=CARTESIAN_POINT('Ctrl Pts',(76.0088951657422,9.34227184804425,55.0960739058512));
#168710=CARTESIAN_POINT('Ctrl Pts',(76.1920017064751,9.26803976442981,55.0615802157063));
#168711=CARTESIAN_POINT('Ctrl Pts',(76.2455092857734,9.24578954932307,55.0515074266961));
#168712=CARTESIAN_POINT('Ctrl Pts',(76.3375595192426,9.20654510345283,55.0341910332881));
#168713=CARTESIAN_POINT('Ctrl Pts',(76.3761931414785,9.18977740701081,55.0269270096716));
#168714=CARTESIAN_POINT('Ctrl Pts',(76.4549500204118,9.15498724871514,55.0121263329532));
#168715=CARTESIAN_POINT('Ctrl Pts',(76.4950627966062,9.13694247373873,55.0045919800011));
#168716=CARTESIAN_POINT('Ctrl Pts',(76.5963392560234,9.09055694127447,54.9855791726483));
#168717=CARTESIAN_POINT('Ctrl Pts',(76.6573393682436,9.06184997572337,54.9741367081107));
#168718=CARTESIAN_POINT('Ctrl Pts',(76.8922677544153,8.94830404035076,54.9301022631335));
#168719=CARTESIAN_POINT('Ctrl Pts',(77.0640274530913,8.85890034629599,54.8979810422508));
#168720=CARTESIAN_POINT('Ctrl Pts',(77.7374145588659,8.48257388663896,54.7722555659475));
#168721=CARTESIAN_POINT('Ctrl Pts',(78.2165102188141,8.15624541629679,54.6833471087575));
#168722=CARTESIAN_POINT('Ctrl Pts',(78.8583656904486,7.63052641390902,54.5632065506372));
#168723=CARTESIAN_POINT('Ctrl Pts',(79.046052664912,7.46445221040781,54.5279196865509));
#168724=CARTESIAN_POINT('Ctrl Pts',(79.2720183543039,7.24859130049152,54.4850424021632));
#168725=CARTESIAN_POINT('Ctrl Pts',(79.3163468927372,7.20543995417531,54.4766109761941));
#168726=CARTESIAN_POINT('Ctrl Pts',(79.3813404360577,7.14096981854607,54.4642153545348));
#168727=CARTESIAN_POINT('Ctrl Pts',(79.4023160899213,7.11997437835274,54.4602095796631));
#168728=CARTESIAN_POINT('Ctrl Pts',(79.4380331741083,7.08389931134314,54.4533790352111));
#168729=CARTESIAN_POINT('Ctrl Pts',(79.4528209754574,7.06886716787826,54.4505481602838));
#168730=CARTESIAN_POINT('Ctrl Pts',(79.4866531021275,7.03425466352652,54.4440649164889));
#168731=CARTESIAN_POINT('Ctrl Pts',(79.5056648237274,7.01464210125918,54.4404168734037));
#168732=CARTESIAN_POINT('Ctrl Pts',(79.5584179895339,6.95976763582236,54.4302814492293));
#168733=CARTESIAN_POINT('Ctrl Pts',(79.591981875593,6.92433171153357,54.4238179607748));
#168734=CARTESIAN_POINT('Ctrl Pts',(79.7965638588489,6.70510676467176,54.3843360198296));
#168735=CARTESIAN_POINT('Ctrl Pts',(79.9608722737452,6.51501149895175,54.3522593994892));
#168736=CARTESIAN_POINT('Ctrl Pts',(80.3920840311058,5.97604670194941,54.2674208018115));
#168737=CARTESIAN_POINT('Ctrl Pts',(80.6435519136396,5.61516681638907,54.2172019806512));
#168738=CARTESIAN_POINT('Ctrl Pts',(80.9869306171769,5.04581875844861,54.1482215178834));
#168739=CARTESIAN_POINT('Ctrl Pts',(81.0966814315515,4.84916834120332,54.1260910013853));
#168740=CARTESIAN_POINT('Ctrl Pts',(81.2688703318115,4.51471138620182,54.0912877876397));
#168741=CARTESIAN_POINT('Ctrl Pts',(81.3349463909953,4.37894758611579,54.0779082500981));
#168742=CARTESIAN_POINT('Ctrl Pts',(81.4230269647992,4.18713452960784,54.0600452865403));
#168743=CARTESIAN_POINT('Ctrl Pts',(81.4476006259695,4.13233514418333,54.0550583321794));
#168744=CARTESIAN_POINT('Ctrl Pts',(81.4888710938237,4.0380560613389,54.0466772699457));
#168745=CARTESIAN_POINT('Ctrl Pts',(81.5058068628168,3.99868699687575,54.0432362906741));
#168746=CARTESIAN_POINT('Ctrl Pts',(81.5376405790069,3.92336838247913,54.0367650370375));
#168747=CARTESIAN_POINT('Ctrl Pts',(81.5525821689485,3.88743887624623,54.0337262026295));
#168748=CARTESIAN_POINT('Ctrl Pts',(81.5870677441897,3.80314194692011,54.026708965883));
#168749=CARTESIAN_POINT('Ctrl Pts',(81.606446418411,3.75470544911803,54.0227629862458));
#168750=CARTESIAN_POINT('Ctrl Pts',(81.6720075827761,3.58708508545596,54.009403032506));
#168751=CARTESIAN_POINT('Ctrl Pts',(81.7163138801765,3.46715189529537,54.0003566798016));
#168752=CARTESIAN_POINT('Ctrl Pts',(81.9773108514265,2.71722016719636,53.9469288886632));
#168753=CARTESIAN_POINT('Ctrl Pts',(82.1338896365648,2.06726251322121,53.9143836481774));
#168754=CARTESIAN_POINT('Ctrl Pts',(82.2344304824298,1.34153292801883,53.8909616529434));
#168755=CARTESIAN_POINT('Ctrl Pts',(82.2427713639767,1.27671987125436,53.8889794911566));
#168756=CARTESIAN_POINT('Ctrl Pts',(82.276435657896,0.993503955104589,53.8807856555322));
#168757=CARTESIAN_POINT('Ctrl Pts',(82.295274739677,0.774361204337858,53.8756581196813));
#168758=CARTESIAN_POINT('Ctrl Pts',(82.3134708763828,0.432230905625216,
53.8693838702499));
#168759=CARTESIAN_POINT('Ctrl Pts',(82.3177570761235,0.309589852688239,
53.8674796615034));
#168760=CARTESIAN_POINT('Ctrl Pts',(82.3204274156931,0.149804214836417,
53.8654232416804));
#168761=CARTESIAN_POINT('Ctrl Pts',(82.3208429435044,0.112708087748638,
53.8649755926801));
#168762=CARTESIAN_POINT('Ctrl Pts',(82.3211871020456,0.0522133541867403,
53.8642932656695));
#168763=CARTESIAN_POINT('Ctrl Pts',(82.3212388760676,0.0288160074678149,
53.8640409935312));
#168764=CARTESIAN_POINT('Ctrl Pts',(82.3211811147386,-0.0168691787927078,
53.8635708552276));
#168765=CARTESIAN_POINT('Ctrl Pts',(82.3210791109962,-0.0391568177109596,
53.8633519112301));
#168766=CARTESIAN_POINT('Ctrl Pts',(82.3206852278142,-0.0890897477102007,
53.8628849579976));
#168767=CARTESIAN_POINT('Ctrl Pts',(82.3203535939649,-0.116734644783884,
53.8626426208118));
#168768=CARTESIAN_POINT('Ctrl Pts',(82.3187874928748,-0.213988775421065,
53.861847756271));
#168769=CARTESIAN_POINT('Ctrl Pts',(82.316946778117,-0.283586979177362,
53.8613828887352));
#168770=CARTESIAN_POINT('Ctrl Pts',(82.2991557836885,-0.767177079712734,
53.858897835677));
#168771=CARTESIAN_POINT('Ctrl Pts',(82.2584877935295,-1.17988250602676,
53.8605891197982));
#168772=CARTESIAN_POINT('Ctrl Pts',(82.1342429030406,-1.952558871361,53.872061384823));
#168773=CARTESIAN_POINT('Ctrl Pts',(82.0560162246229,-2.31271928743464,
53.8809158058714));
#168774=CARTESIAN_POINT('Ctrl Pts',(81.9017699440407,-2.87391172108804,
53.900710332764));
#168775=CARTESIAN_POINT('Ctrl Pts',(81.8386107044225,-3.07821613910783,
53.9092122342016));
#168776=CARTESIAN_POINT('Ctrl Pts',(81.721111382259,-3.41968091595709,53.9256720906166));
#168777=CARTESIAN_POINT('Ctrl Pts',(81.6701355540932,-3.55795232191926,
53.9329770022704));
#168778=CARTESIAN_POINT('Ctrl Pts',(81.5943301119312,-3.75053207398994,
53.9440603926201));
#168779=CARTESIAN_POINT('Ctrl Pts',(81.5719971627679,-3.80583035247125,
53.9473498912265));
#168780=CARTESIAN_POINT('Ctrl Pts',(81.532790358566,-3.90049376959742,53.9531654608353));
#168781=CARTESIAN_POINT('Ctrl Pts',(81.5161516705407,-3.93995733472288,
53.9556454338881));
#168782=CARTESIAN_POINT('Ctrl Pts',(81.483856586521,-4.01521730930301,53.9604813694123));
#168783=CARTESIAN_POINT('Ctrl Pts',(81.4682421529381,-4.05103138978655,
53.9628291141898));
#168784=CARTESIAN_POINT('Ctrl Pts',(81.4270320702046,-4.14407865101693,
53.969049873941));
#168785=CARTESIAN_POINT('Ctrl Pts',(81.4011128110954,-4.20116233767831,
53.9729863851572));
#168786=CARTESIAN_POINT('Ctrl Pts',(81.3086324816435,-4.39990860859872,
53.9871125532471));
#168787=CARTESIAN_POINT('Ctrl Pts',(81.239329630631,-4.54023130294979,53.9978397208571));
#168788=CARTESIAN_POINT('Ctrl Pts',(80.8760439399746,-5.2346670113602,54.0546953060607));
#168789=CARTESIAN_POINT('Ctrl Pts',(80.5344537815953,-5.76148972491485,
54.1101734092115));
#168790=CARTESIAN_POINT('Ctrl Pts',(79.9859644901883,-6.45510492963111,
54.1995242663509));
#168791=CARTESIAN_POINT('Ctrl Pts',(79.8178538190413,-6.65149857516524,
54.2269227678547));
#168792=CARTESIAN_POINT('Ctrl Pts',(79.5996556815575,-6.8871536861063,54.2622927574894));
#168793=CARTESIAN_POINT('Ctrl Pts',(79.5565196799058,-6.9328624728543,54.2692762472393));
#168794=CARTESIAN_POINT('Ctrl Pts',(79.4922205496177,-6.99971254116264,
54.2796691103541));
#168795=CARTESIAN_POINT('Ctrl Pts',(79.4713879305112,-7.02117646285454,
54.2830337910988));
#168796=CARTESIAN_POINT('Ctrl Pts',(79.4356553716273,-7.05766004312809,
54.2888001245902));
#168797=CARTESIAN_POINT('Ctrl Pts',(79.4208034451506,-7.07272732810432,
54.2911954217731));
#168798=CARTESIAN_POINT('Ctrl Pts',(79.386696360594,-7.1071080938456,54.2966928072899));
#168799=CARTESIAN_POINT('Ctrl Pts',(79.3674099458245,-7.12638943274464,
54.2997990151119));
#168800=CARTESIAN_POINT('Ctrl Pts',(79.3136539070021,-7.17968955146655,
54.3084507749134));
#168801=CARTESIAN_POINT('Ctrl Pts',(79.2790159480114,-7.2135338331821,54.3140187729977));
#168802=CARTESIAN_POINT('Ctrl Pts',(79.0719423924536,-7.41291726011599,
54.3472720541034));
#168803=CARTESIAN_POINT('Ctrl Pts',(78.8938754519389,-7.57236573321312,
54.3757324256153));
#168804=CARTESIAN_POINT('Ctrl Pts',(78.3618087989894,-8.01520743096129,
54.4607512174312));
#168805=CARTESIAN_POINT('Ctrl Pts',(77.9940960363526,-8.28074318692409,
54.5195051476434));
#168806=CARTESIAN_POINT('Ctrl Pts',(77.4201452423074,-8.63796573448676,
54.6121014683613));
#168807=CARTESIAN_POINT('Ctrl Pts',(77.2265779505194,-8.74950131171391,
54.6434634275847));
#168808=CARTESIAN_POINT('Ctrl Pts',(76.8973138924305,-8.92459729154222,
54.6970927062953));
#168809=CARTESIAN_POINT('Ctrl Pts',(76.7636018757933,-8.99183526526654,
54.71894516354));
#168810=CARTESIAN_POINT('Ctrl Pts',(76.5746385525104,-9.08151251093388,
54.7499368035909));
#168811=CARTESIAN_POINT('Ctrl Pts',(76.5206034625095,-9.10655673823455,
54.7588112586674));
#168812=CARTESIAN_POINT('Ctrl Pts',(76.427619709887,-9.14862977136467,54.77410350098));
#168813=CARTESIAN_POINT('Ctrl Pts',(76.3887788727589,-9.16590134471883,
54.7804975534351));
#168814=CARTESIAN_POINT('Ctrl Pts',(76.3144570255503,-9.19837386356399,
54.7927444144432));
#168815=CARTESIAN_POINT('Ctrl Pts',(76.2789955185052,-9.21361906807648,
54.7985929234747));
#168816=CARTESIAN_POINT('Ctrl Pts',(76.195774683438,-9.24881597525119,54.8123300449534));
#168817=CARTESIAN_POINT('Ctrl Pts',(76.1479477075382,-9.2685987854853,54.8202338683988));
#168818=CARTESIAN_POINT('Ctrl Pts',(76.0062493555896,-9.32590025881121,
54.8436771996773));
#168819=CARTESIAN_POINT('Ctrl Pts',(75.9119651267375,-9.36234106087739,
54.8593102153508));
#168820=CARTESIAN_POINT('Ctrl Pts',(75.3118761807926,-9.58366164047387,
54.9590132520356));
#168821=CARTESIAN_POINT('Ctrl Pts',(74.7925845473,-9.72782934484848,55.0462669218385));
#168822=CARTESIAN_POINT('Ctrl Pts',(74.0644117936631,-9.86642499906641,
55.1688941422367));
#168823=CARTESIAN_POINT('Ctrl Pts',(73.8633764656079,-9.89819553156769,
55.2027692482083));
#168824=CARTESIAN_POINT('Ctrl Pts',(73.4413329594399,-9.95138883419935,
55.2737825627323));
#168825=CARTESIAN_POINT('Ctrl Pts',(73.220287607698,-9.97159664074993,55.3109177917393));
#168826=CARTESIAN_POINT('Ctrl Pts',(72.8760764633516,-9.99122019912003,
55.3684894585483));
#168827=CARTESIAN_POINT('Ctrl Pts',(72.7532945491389,-9.99588891031017,
55.388975041455));
#168828=CARTESIAN_POINT('Ctrl Pts',(72.5936643706124,-9.99893268868906,
55.4155170311351));
#168829=CARTESIAN_POINT('Ctrl Pts',(72.5568768047025,-9.99942547234498,
55.42162744313));
#168830=CARTESIAN_POINT('Ctrl Pts',(72.4969617697601,-9.99988827267009,
55.4315681290353));
#168831=CARTESIAN_POINT('Ctrl Pts',(72.473836281552,-9.99998447862849,55.4354022329856));
#168832=CARTESIAN_POINT('Ctrl Pts',(72.4287486002363,-10.0000113655624,
55.4428720045041));
#168833=CARTESIAN_POINT('Ctrl Pts',(72.4067866556855,-9.99995013715283,
55.4465078942291));
#168834=CARTESIAN_POINT('Ctrl Pts',(72.3576527872722,-9.99964687954154,
55.4546366461243));
#168835=CARTESIAN_POINT('Ctrl Pts',(72.3304810170454,-9.99936540541892,
55.4591281662376));
#168836=CARTESIAN_POINT('Ctrl Pts',(72.236069194814,-9.99799207134238,55.4747220460726));
#168837=CARTESIAN_POINT('Ctrl Pts',(72.168836279222,-9.99631730448874,55.4858048194902));
#168838=CARTESIAN_POINT('Ctrl Pts',(71.6332099388321,-9.97742156908948,
55.5739475648411));
#168839=CARTESIAN_POINT('Ctrl Pts',(71.1664022631159,-9.92709917372414,
55.649874924514));
#168840=CARTESIAN_POINT('Ctrl Pts',(70.2990500426836,-9.76972412554119,
55.7908978432573));
#168841=CARTESIAN_POINT('Ctrl Pts',(69.8981505391108,-9.67039968655334,
55.8560566156195));
#168842=CARTESIAN_POINT('Ctrl Pts',(69.360426388242,-9.50038366337385,55.9438648269308));
#168843=CARTESIAN_POINT('Ctrl Pts',(69.2173034382342,-9.45144975200689,
55.9672747092599));
#168844=CARTESIAN_POINT('Ctrl Pts',(68.9688955928456,-9.36002750779578,
56.0079846396261));
#168845=CARTESIAN_POINT('Ctrl Pts',(68.863116536288,-9.31899384159476,56.025345613222));
#168846=CARTESIAN_POINT('Ctrl Pts',(68.7084819839311,-9.25589200635337,
56.0507639611599));
#168847=CARTESIAN_POINT('Ctrl Pts',(68.6590658553943,-9.23525193677671,
56.0588927447682));
#168848=CARTESIAN_POINT('Ctrl Pts',(68.571604027354,-9.19787496467867,56.0732903662859));
#168849=CARTESIAN_POINT('Ctrl Pts',(68.5334920325762,-9.18129991243966,
56.0795677664839));
#168850=CARTESIAN_POINT('Ctrl Pts',(68.4534208575969,-9.14586866114537,
56.092763620191));
#168851=CARTESIAN_POINT('Ctrl Pts',(68.4114862316701,-9.12695825300877,
56.0996788183473));
#168852=CARTESIAN_POINT('Ctrl Pts',(68.3003198882863,-9.07588229154613,
56.1180217880321));
#168853=CARTESIAN_POINT('Ctrl Pts',(68.2313240728367,-9.04319972476277,
56.1294180387994));
#168854=CARTESIAN_POINT('Ctrl Pts',(67.90868660651,-8.88572754178351,56.1827600856701));
#168855=CARTESIAN_POINT('Ctrl Pts',(67.6600492701548,-8.75076564379417,
56.2240219958622));
#168856=CARTESIAN_POINT('Ctrl Pts',(67.3490278159051,-8.5641259941554,56.2757336587115));
#168857=CARTESIAN_POINT('Ctrl Pts',(67.281081731324,-8.52221891537737,56.2870364344169));
#168858=CARTESIAN_POINT('Ctrl Pts',(66.8475450273114,-8.24748818106823,
56.3591748668246));
#168859=CARTESIAN_POINT('Ctrl Pts',(66.4968897155404,-7.9913824010402,56.4176380260284));
#168860=CARTESIAN_POINT('Ctrl Pts',(66.1388228350229,-7.69190120586487,
56.4768040865882));
#168861=CARTESIAN_POINT('Ctrl Pts',(66.1139167964462,-7.67086064018072,
56.4809164238193));
#168862=CARTESIAN_POINT('Ctrl Pts',(65.9345674453173,-7.51782555568169,
56.5105048782737));
#168863=CARTESIAN_POINT('Ctrl Pts',(65.784032712273,-7.38117650470982,56.5352075344276));
#168864=CARTESIAN_POINT('Ctrl Pts',(65.604254505522,-7.20765368370613,56.5644391530346));
#168865=CARTESIAN_POINT('Ctrl Pts',(65.5710237318134,-7.17512718210399,
56.5698305674089));
#168866=CARTESIAN_POINT('Ctrl Pts',(65.5189726379127,-7.123461954634,56.5782549195736));
#168867=CARTESIAN_POINT('Ctrl Pts',(65.5000027673707,-7.10448025204775,
56.5813207922665));
#168868=CARTESIAN_POINT('Ctrl Pts',(65.4644883849773,-7.06865608901523,
56.5870519399276));
#168869=CARTESIAN_POINT('Ctrl Pts',(65.4479270456507,-7.05183142572946,
56.5897209315517));
#168870=CARTESIAN_POINT('Ctrl Pts',(65.4090356116518,-7.0120404790486,56.5959802635103));
#168871=CARTESIAN_POINT('Ctrl Pts',(65.386755163371,-6.98902434700317,56.5995596607279));
#168872=CARTESIAN_POINT('Ctrl Pts',(65.3129436490221,-6.91203825063574,
56.6113969656744));
#168873=CARTESIAN_POINT('Ctrl Pts',(65.2618982686334,-6.85758993200706,
56.6195494011052));
#168874=CARTESIAN_POINT('Ctrl Pts',(65.1388223373986,-6.72332668785601,
56.6391321476672));
#168875=CARTESIAN_POINT('Ctrl Pts',(65.0674497246677,-6.64290133226429,
56.6504250103216));
#168876=CARTESIAN_POINT('Ctrl Pts',(64.7757628926427,-6.30334296580469,
56.696356036263));
#168877=CARTESIAN_POINT('Ctrl Pts',(64.567279703089,-6.03403361031762,56.728652476967));
#168878=CARTESIAN_POINT('Ctrl Pts',(64.0898352801356,-5.347693351677,56.8019553473707));
#168879=CARTESIAN_POINT('Ctrl Pts',(63.8371691512065,-4.92014170759687,
56.8401663806758));
#168880=CARTESIAN_POINT('Ctrl Pts',(63.5697093128545,-4.37985868116106,
56.8804099584722));
#168881=CARTESIAN_POINT('Ctrl Pts',(63.5239486482656,-4.28360130353994,
56.8872844017001));
#168882=CARTESIAN_POINT('Ctrl Pts',(63.4579255521113,-4.13883253849201,
56.8971878629492));
#168883=CARTESIAN_POINT('Ctrl Pts',(63.4365041515282,-4.09087068057834,
56.9003985406832));
#168884=CARTESIAN_POINT('Ctrl Pts',(63.3987144393805,-4.00444992785842,
56.9060579923265));
#168885=CARTESIAN_POINT('Ctrl Pts',(63.3822088239391,-3.96605384609136,
56.9085282719715));
#168886=CARTESIAN_POINT('Ctrl Pts',(63.3475157417985,-3.88394384615661,
56.9137169970989));
#168887=CARTESIAN_POINT('Ctrl Pts',(63.3293963000288,-3.84020162926648,
56.9164247921415));
#168888=CARTESIAN_POINT('Ctrl Pts',(63.2810364195707,-3.72108702589698,
56.9236456267113));
#168889=CARTESIAN_POINT('Ctrl Pts',(63.2513960239245,-3.64546930100763,
56.9280646315525));
#168890=CARTESIAN_POINT('Ctrl Pts',(63.0854956548177,-3.2066900231416,56.9527544844642));
#168891=CARTESIAN_POINT('Ctrl Pts',(62.969323373679,-2.83611714315204,56.9698823456802));
#168892=CARTESIAN_POINT('Ctrl Pts',(62.7617540923111,-2.01021801408222,
56.9996293841591));
#168893=CARTESIAN_POINT('Ctrl Pts',(62.6797801102224,-1.55339843102113,
57.0107007668451));
#168894=CARTESIAN_POINT('Ctrl Pts',(62.5986264616137,-0.81308586318316,
57.0190240053952));
#168895=CARTESIAN_POINT('Ctrl Pts',(62.5795904035836,-0.53250455818361,
57.0199893052929));
#168896=CARTESIAN_POINT('Ctrl Pts',(62.5709959477977,-0.207453005027223,
57.0183414650338));
#168897=CARTESIAN_POINT('Ctrl Pts',(62.5701165430882,-0.163395897912248,
57.0180593755872));
#168898=CARTESIAN_POINT('Ctrl Pts',(62.5691510877258,-0.0918065422875012,
57.0175041376516));
#168899=CARTESIAN_POINT('Ctrl Pts',(62.5688911701614,-0.0642769573281793,
57.0172673519341));
#168900=CARTESIAN_POINT('Ctrl Pts',(62.5686764252568,-0.0244979264229797,
57.0168912699599));
#168901=CARTESIAN_POINT('Ctrl Pts',(62.568632333185,-0.0122489680148922,
57.0167708154386));
#168902=CARTESIAN_POINT('Ctrl Pts',(62.5686102705547,6.5620497147992E-11,
57.0166456920447));
#168903=CARTESIAN_POINT('Ctrl Pts',(62.5638890606905,-6.14161654078813E-11,
56.9898703803749));
#168904=CARTESIAN_POINT('Ctrl Pts',(62.5639048106942,-0.00874425629257516,
56.9899597030843));
#168905=CARTESIAN_POINT('Ctrl Pts',(62.5639319241146,-0.0174885217134871,
56.9900474219547));
#168906=CARTESIAN_POINT('Ctrl Pts',(62.5640841001605,-0.0520730401625098,
56.9903879897772));
#168907=CARTESIAN_POINT('Ctrl Pts',(62.5642970225908,-0.0779128924089415,
56.9906283809511));
#168908=CARTESIAN_POINT('Ctrl Pts',(62.5651762302007,-0.15070063633938,
56.9912654398587));
#168909=CARTESIAN_POINT('Ctrl Pts',(62.5660707769559,-0.197645389445814,
56.9916293213419));
#168910=CARTESIAN_POINT('Ctrl Pts',(62.5736186133931,-0.487618141777484,
56.9935805014495));
#168911=CARTESIAN_POINT('Ctrl Pts',(62.5887144581143,-0.730354657305291,
56.9939254030249));
#168912=CARTESIAN_POINT('Ctrl Pts',(62.6602708834771,-1.45741667314123,
56.9907005442943));
#168913=CARTESIAN_POINT('Ctrl Pts',(62.7429552688184,-1.93841296625004,
56.9828230429895));
#168914=CARTESIAN_POINT('Ctrl Pts',(62.9483681114407,-2.77006385693597,
56.957743000169));
#168915=CARTESIAN_POINT('Ctrl Pts',(63.0564139232463,-3.12346042605179,
56.9432843019352));
#168916=CARTESIAN_POINT('Ctrl Pts',(63.2184791926907,-3.56570967861722,
56.9201024405613));
#168917=CARTESIAN_POINT('Ctrl Pts',(63.2549803027769,-3.6608505069661,56.9148064003663));
#168918=CARTESIAN_POINT('Ctrl Pts',(63.3121282485612,-3.80334462471342,
56.9064056031722));
#168919=CARTESIAN_POINT('Ctrl Pts',(63.331717051862,-3.85112708511771,56.9035081504862));
#168920=CARTESIAN_POINT('Ctrl Pts',(63.3677908177045,-3.93723865233663,
56.8981407074137));
#168921=CARTESIAN_POINT('Ctrl Pts',(63.3841494476181,-3.97562091678728,
56.8956954780285));
#168922=CARTESIAN_POINT('Ctrl Pts',(63.4198205618877,-4.05790219711481,
56.8903398536623));
#168923=CARTESIAN_POINT('Ctrl Pts',(63.4392083692609,-4.1017664498802,56.8874146633555));
#168924=CARTESIAN_POINT('Ctrl Pts',(63.4925678346612,-4.22020616114003,
56.8793260952426));
#168925=CARTESIAN_POINT('Ctrl Pts',(63.5271319264544,-4.29450261412776,
56.8740465054666));
#168926=CARTESIAN_POINT('Ctrl Pts',(63.7590275000885,-4.77752680016275,
56.8383760630443));
#168927=CARTESIAN_POINT('Ctrl Pts',(63.9826338898768,-5.17265936184192,
56.8028104026162));
#168928=CARTESIAN_POINT('Ctrl Pts',(64.4547827721841,-5.88924006652601,
56.7265466941171));
#168929=CARTESIAN_POINT('Ctrl Pts',(64.6977265994312,-6.21338701041532,
56.6868723392755));
#168930=CARTESIAN_POINT('Ctrl Pts',(65.0356423656362,-6.61131597155861,
56.6318696549662));
#168931=CARTESIAN_POINT('Ctrl Pts',(65.113356983297,-6.69961181644092,56.6192323398752));
#168932=CARTESIAN_POINT('Ctrl Pts',(65.2463560925697,-6.8454178625359,56.5976524902197));
#168933=CARTESIAN_POINT('Ctrl Pts',(65.3008083608359,-6.90368830470944,
56.588830066336));
#168934=CARTESIAN_POINT('Ctrl Pts',(65.3786909853988,-6.98504357620948,
56.5762367162863));
#168935=CARTESIAN_POINT('Ctrl Pts',(65.401548852792,-7.0086841747057,56.5725436880927));
#168936=CARTESIAN_POINT('Ctrl Pts',(65.4411028926908,-7.04918753222754,
56.5661589571686));
#168937=CARTESIAN_POINT('Ctrl Pts',(65.4577433836709,-7.06610545522635,
56.5634746450491));
#168938=CARTESIAN_POINT('Ctrl Pts',(65.4930300338297,-7.10172363384591,
56.5577864140044));
#168939=CARTESIAN_POINT('Ctrl Pts',(65.5116902391882,-7.12040918973532,
56.554780625295));
#168940=CARTESIAN_POINT('Ctrl Pts',(65.5628939954417,-7.17127433189184,
56.546538332892));
#168941=CARTESIAN_POINT('Ctrl Pts',(65.5955845506883,-7.20330184430556,
56.5412822664836));
#168942=CARTESIAN_POINT('Ctrl Pts',(65.7607424802654,-7.36288330519642,
56.5147536748528));
#168943=CARTESIAN_POINT('Ctrl Pts',(65.8964832888361,-7.48692321207819,
56.4930324849991));
#168944=CARTESIAN_POINT('Ctrl Pts',(66.4009042442753,-7.92274306796178,
56.4123979103522));
#168945=CARTESIAN_POINT('Ctrl Pts',(66.7885361015779,-8.21100398364867,
56.3505541015775));
#168946=CARTESIAN_POINT('Ctrl Pts',(67.5031435033192,-8.66532340663204,
56.2354021021567));
#168947=CARTESIAN_POINT('Ctrl Pts',(67.8214377641631,-8.84371012032256,
56.1837646318747));
#168948=CARTESIAN_POINT('Ctrl Pts',(68.2193241461475,-9.03851891805217,
56.1186290174417));
#168949=CARTESIAN_POINT('Ctrl Pts',(68.2904110854443,-9.07227142317338,
56.1069705707629));
#168950=CARTESIAN_POINT('Ctrl Pts',(68.4041374089743,-9.12460444621562,
56.0882849371297));
#168951=CARTESIAN_POINT('Ctrl Pts',(68.4465240490322,-9.14374564342729,
56.0813131965866));
#168952=CARTESIAN_POINT('Ctrl Pts',(68.5269485355556,-9.17937837010611,
56.0680708893829));
#168953=CARTESIAN_POINT('Ctrl Pts',(68.5649588266528,-9.19593181819053,
56.0618063860581));
#168954=CARTESIAN_POINT('Ctrl Pts',(68.6514798250429,-9.23296110311935,
56.0475334547496));
#168955=CARTESIAN_POINT('Ctrl Pts',(68.7000508742162,-9.25328742867254,
56.03951147355));
#168956=CARTESIAN_POINT('Ctrl Pts',(68.8493684080386,-9.31436638570483,
56.0148216675348));
#168957=CARTESIAN_POINT('Ctrl Pts',(68.950614579436,-9.35382920653745,55.9980408258301));
#168958=CARTESIAN_POINT('Ctrl Pts',(69.6239156277413,-9.60344000676977,
55.8861985455837));
#168959=CARTESIAN_POINT('Ctrl Pts',(70.2132461915203,-9.76124515803727,
55.7870277437451));
#168960=CARTESIAN_POINT('Ctrl Pts',(71.2518707369074,-9.93740617960594,
55.612090530215));
#168961=CARTESIAN_POINT('Ctrl Pts',(71.6950729655319,-9.9816310694202,55.5374264880331));
#168962=CARTESIAN_POINT('Ctrl Pts',(72.1989191972304,-9.9971887668825,55.4534789531029));
#168963=CARTESIAN_POINT('Ctrl Pts',(72.2580211260633,-9.9984747446368,55.4436466337144));
#168964=CARTESIAN_POINT('Ctrl Pts',(72.344917857463,-9.99957344353141,55.4292154920077));
#168965=CARTESIAN_POINT('Ctrl Pts',(72.3727040188649,-9.99980575215838,
55.4246047638297));
#168966=CARTESIAN_POINT('Ctrl Pts',(72.421983935016,-10.000006713663,55.4164345823164));
#168967=CARTESIAN_POINT('Ctrl Pts',(72.4434769586677,-10.0000231723034,
55.4128736532062));
#168968=CARTESIAN_POINT('Ctrl Pts',(72.4903076247572,-9.99990392767021,
55.4051202020519));
#168969=CARTESIAN_POINT('Ctrl Pts',(72.5156450036992,-9.9997404871866,55.4009286412189));
#168970=CARTESIAN_POINT('Ctrl Pts',(72.5866015198404,-9.99900574340614,
55.3891993138661));
#168971=CARTESIAN_POINT('Ctrl Pts',(72.6322189492257,-9.99821268572863,
55.3816690364506));
#168972=CARTESIAN_POINT('Ctrl Pts',(72.9050365506192,-9.99155150476078,
55.3366902802793));
#168973=CARTESIAN_POINT('Ctrl Pts',(73.1320239336223,-9.97805050031943,
55.299500524875));
#168974=CARTESIAN_POINT('Ctrl Pts',(73.8723630421821,-9.90795594389078,
55.1786006524985));
#168975=CARTESIAN_POINT('Ctrl Pts',(74.3819007130795,-9.81851031796833,
55.0959777979692));
#168976=CARTESIAN_POINT('Ctrl Pts',(75.2492126808648,-9.59414504533403,
54.9547787271946));
#168977=CARTESIAN_POINT('Ctrl Pts',(75.6105586599862,-9.47785607708538,
54.8957844722876));
#168978=CARTESIAN_POINT('Ctrl Pts',(76.039138866956,-9.31184736326088,54.8254460527912));
#168979=CARTESIAN_POINT('Ctrl Pts',(76.1135603183451,-9.28196303542946,
54.8132189354172));
#168980=CARTESIAN_POINT('Ctrl Pts',(76.2308611590211,-9.23317719069522,
54.7939259638552));
#168981=CARTESIAN_POINT('Ctrl Pts',(76.2739822738814,-9.21487874247212,
54.786829121736));
#168982=CARTESIAN_POINT('Ctrl Pts',(76.3549685073991,-9.17982407794511,
54.7734920087945));
#168983=CARTESIAN_POINT('Ctrl Pts',(76.3928614109974,-9.16313602837341,
54.7672481484521));
#168984=CARTESIAN_POINT('Ctrl Pts',(76.4782058085163,-9.12490215953699,
54.7531775854325));
#168985=CARTESIAN_POINT('Ctrl Pts',(76.5255945940612,-9.10321640661647,
54.7453591941456));
#168986=CARTESIAN_POINT('Ctrl Pts',(76.6688345474428,-9.0362802123121,54.7217107756027));
#168987=CARTESIAN_POINT('Ctrl Pts',(76.7641363743965,-8.98984686695501,
54.705954640819));
#168988=CARTESIAN_POINT('Ctrl Pts',(77.2461724703858,-8.74523439689092,
54.6261599702734));
#168989=CARTESIAN_POINT('Ctrl Pts',(77.620400450887,-8.52293752160539,54.5638520549711));
#168990=CARTESIAN_POINT('Ctrl Pts',(78.3814407573017,-7.99977242272465,
54.4371933896669));
#168991=CARTESIAN_POINT('Ctrl Pts',(78.7631499228351,-7.69334239791074,
54.3736980258993));
#168992=CARTESIAN_POINT('Ctrl Pts',(79.1833438484766,-7.30170514217075,
54.3050300703362));
#168993=CARTESIAN_POINT('Ctrl Pts',(79.2447723351254,-7.24296442069717,
54.2950260769044));
#168994=CARTESIAN_POINT('Ctrl Pts',(79.3295202093867,-7.15982482882853,
54.2812822949792));
#168995=CARTESIAN_POINT('Ctrl Pts',(79.3534667918142,-7.13609334314239,
54.277405419675));
#168996=CARTESIAN_POINT('Ctrl Pts',(79.3941592448955,-7.09535577787191,
54.2708294768964));
#168997=CARTESIAN_POINT('Ctrl Pts',(79.4109641753367,-7.07841117522327,
54.2681173388886));
#168998=CARTESIAN_POINT('Ctrl Pts',(79.4459815862858,-7.04284874296726,
54.2624736145624));
#168999=CARTESIAN_POINT('Ctrl Pts',(79.4641824196779,-7.02421949107003,
54.2595445691453));
#169000=CARTESIAN_POINT('Ctrl Pts',(79.513008143897,-6.97385198985392,54.2516984130922));
#169001=CARTESIAN_POINT('Ctrl Pts',(79.5434984041737,-6.94197945022565,
54.2468108204876));
#169002=CARTESIAN_POINT('Ctrl Pts',(79.6861602446116,-6.79085968815471,
54.2239955429386));
#169003=CARTESIAN_POINT('Ctrl Pts',(79.7956455858884,-6.66902459748612,
54.2066429991632));
#169004=CARTESIAN_POINT('Ctrl Pts',(80.2267826464556,-6.16487688083918,
54.1387986603288));
#169005=CARTESIAN_POINT('Ctrl Pts',(80.5229187285858,-5.76103577948711,
54.0933115275005));
#169006=CARTESIAN_POINT('Ctrl Pts',(80.9859758920753,-5.01893562440335,
54.0228232777364));
#169007=CARTESIAN_POINT('Ctrl Pts',(81.1662796979998,-4.6904340730106,53.9956134771049));
#169008=CARTESIAN_POINT('Ctrl Pts',(81.3622967684329,-4.28055019252815,
53.966158591484));
#169009=CARTESIAN_POINT('Ctrl Pts',(81.395833003133,-4.2082274332321,53.961125131984));
#169010=CARTESIAN_POINT('Ctrl Pts',(81.4477768954247,-4.09262701861121,
53.9533378873362));
#169011=CARTESIAN_POINT('Ctrl Pts',(81.4667446710304,-4.049610798616,53.9504963383642));
#169012=CARTESIAN_POINT('Ctrl Pts',(81.5020247955879,-3.96805749591278,
53.9452149160665));
#169013=CARTESIAN_POINT('Ctrl Pts',(81.518399363777,-3.92954906842659,53.9427652968102));
#169014=CARTESIAN_POINT('Ctrl Pts',(81.5549902306172,-3.84198567105462,
53.9372951733079));
#169015=CARTESIAN_POINT('Ctrl Pts',(81.5750603612961,-3.79286957566594,
53.9342975599772));
#169016=CARTESIAN_POINT('Ctrl Pts',(81.6352357774534,-3.64221830543486,
53.9253188579434));
#169017=CARTESIAN_POINT('Ctrl Pts',(81.6740835041807,-3.54017802959526,
53.9195349312583));
#169018=CARTESIAN_POINT('Ctrl Pts',(81.9237696760773,-2.85086037712017,
53.882460478916));
#169019=CARTESIAN_POINT('Ctrl Pts',(82.0814713195126,-2.2453733369779,53.8594438534479));
#169020=CARTESIAN_POINT('Ctrl Pts',(82.256746478396,-1.17615855835889,53.8368639699584));
#169021=CARTESIAN_POINT('Ctrl Pts',(82.3001946479318,-0.71871137215977,
53.8327602561505));
#169022=CARTESIAN_POINT('Ctrl Pts',(82.3140815183159,-0.209373276771355,
53.835255984522));
#169023=CARTESIAN_POINT('Ctrl Pts',(82.3150838110856,-0.158830585887076,
53.8355808789653));
#169024=CARTESIAN_POINT('Ctrl Pts',(82.3160370752743,-0.0819760675386363,
53.8361943511674));
#169025=CARTESIAN_POINT('Ctrl Pts',(82.3162617093688,-0.0556680090297576,
53.8364256253505));
#169026=CARTESIAN_POINT('Ctrl Pts',(82.3164863334048,-0.00762243364845737,
53.8368871971331));
#169027=CARTESIAN_POINT('Ctrl Pts',(82.3165185791312,0.0141146339893455,
53.8371107070966));
#169028=CARTESIAN_POINT('Ctrl Pts',(82.3164346784136,0.063224861308948,
53.837648825507));
#169029=CARTESIAN_POINT('Ctrl Pts',(82.3162778802675,0.0905975249978633,
53.8379719860563));
#169030=CARTESIAN_POINT('Ctrl Pts',(82.3155865374829,0.161507002415424,
53.8388687996983));
#169031=CARTESIAN_POINT('Ctrl Pts',(82.314883587652,0.205041158632895,53.8394776570823));
#169032=CARTESIAN_POINT('Ctrl Pts',(82.3079889008431,0.510802990607056,
53.8441577376328));
#169033=CARTESIAN_POINT('Ctrl Pts',(82.2919674719939,0.772677712118657,
53.8502504859091));
#169034=CARTESIAN_POINT('Ctrl Pts',(82.2177367663576,1.51415398010765,53.8729831907986));
#169035=CARTESIAN_POINT('Ctrl Pts',(82.135457198763,1.99047392445941,53.8941270711762));
#169036=CARTESIAN_POINT('Ctrl Pts',(81.9262807030074,2.83553129188075,53.9423026425108));
#169037=CARTESIAN_POINT('Ctrl Pts',(81.8114387948367,3.20636697051633,53.9673391598683));
#169038=CARTESIAN_POINT('Ctrl Pts',(81.6471251739613,3.64541629284319,54.0016021234051));
#169039=CARTESIAN_POINT('Ctrl Pts',(81.6177722627172,3.72104582720717,54.0076758855493));
#169040=CARTESIAN_POINT('Ctrl Pts',(81.5698686599173,3.84017489669624,54.0175160569567));
#169041=CARTESIAN_POINT('Ctrl Pts',(81.5519183455955,3.88391965542935,54.021188325486));
#169042=CARTESIAN_POINT('Ctrl Pts',(81.5175446855735,3.96603189838918,54.0281927897874));
#169043=CARTESIAN_POINT('Ctrl Pts',(81.5011894137835,4.00442767400094,54.0315143061468));
#169044=CARTESIAN_POINT('Ctrl Pts',(81.4637405211422,4.09084432015889,54.0390947269212));
#169045=CARTESIAN_POINT('Ctrl Pts',(81.4425096293239,4.13880245320339,54.0433751099671));
#169046=CARTESIAN_POINT('Ctrl Pts',(81.3770694274902,4.28354766761194,54.0565180611151));
#169047=CARTESIAN_POINT('Ctrl Pts',(81.3317015292353,4.37978590023679,54.0655621495879));
#169048=CARTESIAN_POINT('Ctrl Pts',(81.0663475117984,4.92020669174828,54.1181058290861));
#169049=CARTESIAN_POINT('Ctrl Pts',(80.8153664984999,5.34790961034214,54.1664424600943));
#169050=CARTESIAN_POINT('Ctrl Pts',(80.340863807801,6.03429225825351,54.2568583282166));
#169051=CARTESIAN_POINT('Ctrl Pts',(80.1336697962211,6.30350740048645,54.2961101599799));
#169052=CARTESIAN_POINT('Ctrl Pts',(79.8436844595481,6.64296231786595,54.3512072844235));
#169053=CARTESIAN_POINT('Ctrl Pts',(79.7727129014199,6.72337284533554,54.3647040892111));
#169054=CARTESIAN_POINT('Ctrl Pts',(79.650315335197,6.85761401006886,54.3880221602967));
#169055=CARTESIAN_POINT('Ctrl Pts',(79.5995467102453,6.91205498687755,54.3977057535891));
#169056=CARTESIAN_POINT('Ctrl Pts',(79.5261295227144,6.98903240629104,54.4117319905841));
#169057=CARTESIAN_POINT('Ctrl Pts',(79.5039662296407,7.01204730899201,54.415969143727));
#169058=CARTESIAN_POINT('Ctrl Pts',(79.4652776506389,7.05183683794212,54.4233711958869));
#169059=CARTESIAN_POINT('Ctrl Pts',(79.4488019709314,7.06866133000351,54.4265251517593));
#169060=CARTESIAN_POINT('Ctrl Pts',(79.4134698112614,7.10448596620821,54.4332927672804));
#169061=CARTESIAN_POINT('Ctrl Pts',(79.3945965053637,7.12346829623868,54.4369101356577));
#169062=CARTESIAN_POINT('Ctrl Pts',(79.3428075179754,7.1751370199094,54.4468421140114));
#169063=CARTESIAN_POINT('Ctrl Pts',(79.3097423312075,7.20766626817661,54.4531896283703));
#169064=CARTESIAN_POINT('Ctrl Pts',(79.1308126585927,7.38124353577852,54.4875672255652));
#169065=CARTESIAN_POINT('Ctrl Pts',(78.9809592267362,7.5179392764787,54.5164585031576));
#169066=CARTESIAN_POINT('Ctrl Pts',(78.7659132462544,7.70230324834318,54.5579463371169));
#169067=CARTESIAN_POINT('Ctrl Pts',(78.7041060083003,7.75399196895421,54.5698736847609));
#169068=CARTESIAN_POINT('Ctrl Pts',(78.3651033906683,8.03050374358188,54.6352864840647));
#169069=CARTESIAN_POINT('Ctrl Pts',(78.0767261091754,8.24069103972816,54.690895673929));
#169070=CARTESIAN_POINT('Ctrl Pts',(77.4559767767363,8.6432051992923,54.8099060922709));
#169071=CARTESIAN_POINT('Ctrl Pts',(77.1224530774971,8.83260080551398,54.8734731198974));
#169072=CARTESIAN_POINT('Ctrl Pts',(76.7077133980001,9.03679804891313,54.9518660116191));
#169073=CARTESIAN_POINT('Ctrl Pts',(76.6361534303869,9.0709509493595,54.965370282055));
#169074=CARTESIAN_POINT('Ctrl Pts',(76.5219475383449,9.12375354817043,54.9868873388191));
#169075=CARTESIAN_POINT('Ctrl Pts',(76.4795658829586,9.14298064343171,54.9948647314446));
#169076=CARTESIAN_POINT('Ctrl Pts',(76.3993259076638,9.17869067788625,55.0099538449014));
#169077=CARTESIAN_POINT('Ctrl Pts',(76.3614967980352,9.19523835344236,55.0170616746659));
#169078=CARTESIAN_POINT('Ctrl Pts',(76.2756299004896,9.2321495804909,55.0331821347635));
#169079=CARTESIAN_POINT('Ctrl Pts',(76.227532501316,9.25236785124801,55.0422024450543));
#169080=CARTESIAN_POINT('Ctrl Pts',(76.0805651359703,9.3127595752547,55.069736909107));
#169081=CARTESIAN_POINT('Ctrl Pts',(75.9812043418301,9.35168845087595,55.0883135700301));
#169082=CARTESIAN_POINT('Ctrl Pts',(75.2931596348921,9.60826605919751,55.2167002413699));
#169083=CARTESIAN_POINT('Ctrl Pts',(74.6855912582973,9.76989317578111,55.3286928604313));
#169084=CARTESIAN_POINT('Ctrl Pts',(73.6321391316903,9.94318768375844,55.522789014864));
#169085=CARTESIAN_POINT('Ctrl Pts',(73.1930053790114,9.98493428019243,55.6037117635221));
#169086=CARTESIAN_POINT('Ctrl Pts',(72.7029467250109,9.9979256930175,55.694960163832));
#169087=CARTESIAN_POINT('Ctrl Pts',(72.6531315046462,9.99886095488647,55.7042467602897));
#169088=CARTESIAN_POINT('Ctrl Pts',(72.5774259419976,9.99969682257542,55.7183787647901));
#169089=CARTESIAN_POINT('Ctrl Pts',(72.5515377852804,9.99987862366171,55.7232146832859));
#169090=CARTESIAN_POINT('Ctrl Pts',(72.5042828402994,10.0000205845329,55.7320484211217));
#169091=CARTESIAN_POINT('Ctrl Pts',(72.4829163066571,10.0000139057263,55.7360450880897));
#169092=CARTESIAN_POINT('Ctrl Pts',(72.4346726634354,9.99983880914977,55.7450747031514));
#169093=CARTESIAN_POINT('Ctrl Pts',(72.4077962778869,9.99962911452292,55.7501088994363));
#169094=CARTESIAN_POINT('Ctrl Pts',(72.3382258937914,9.99879598271771,55.7631494480421));
#169095=CARTESIAN_POINT('Ctrl Pts',(72.2955354281879,9.99800165579471,55.7711606540961));
#169096=CARTESIAN_POINT('Ctrl Pts',(71.9981023893323,9.99049448649122,55.8270343437193));
#169097=CARTESIAN_POINT('Ctrl Pts',(71.7437457656726,9.97398701442876,55.8751104491177));
#169098=CARTESIAN_POINT('Ctrl Pts',(71.017115524852,9.89786623642907,56.0128432983893));
#169099=CARTESIAN_POINT('Ctrl Pts',(70.5481352206956,9.81338292517933,56.1021881265229));
#169100=CARTESIAN_POINT('Ctrl Pts',(69.7147906404286,9.59883684736049,56.2604668434973));
#169101=CARTESIAN_POINT('Ctrl Pts',(69.3484224369646,9.48090110005274,56.3298824314981));
#169102=CARTESIAN_POINT('Ctrl Pts',(68.914951695536,9.31238457812526,56.4116298632164));
#169103=CARTESIAN_POINT('Ctrl Pts',(68.8405360341388,9.28239052189889,56.4256505178875));
#169104=CARTESIAN_POINT('Ctrl Pts',(68.723348061904,9.23346461477021,56.447708708801));
#169105=CARTESIAN_POINT('Ctrl Pts',(68.680335524265,9.21514227075404,56.4558003620636));
#169106=CARTESIAN_POINT('Ctrl Pts',(68.5996154173579,9.18006900149048,56.470977171782));
#169107=CARTESIAN_POINT('Ctrl Pts',(68.5618800883034,9.16338727445543,56.4780685528012));
#169108=CARTESIAN_POINT('Ctrl Pts',(68.4769738101259,9.1252065933094,56.4940166647823));
#169109=CARTESIAN_POINT('Ctrl Pts',(68.4298639917344,9.10356914712618,56.5028598990496));
#169110=CARTESIAN_POINT('Ctrl Pts',(68.2877655275524,9.03692717279299,56.5295178725263));
#169111=CARTESIAN_POINT('Ctrl Pts',(68.1933114847173,8.9907544385833,56.5472156600384));
#169112=CARTESIAN_POINT('Ctrl Pts',(67.6546182481865,8.71655948243433,56.6480378507247));
#169113=CARTESIAN_POINT('Ctrl Pts',(67.2271018241678,8.45602107943999,56.7275604431778));
#169114=CARTESIAN_POINT('Ctrl Pts',(66.5517277760748,7.9700333942638,56.8534110931146));
#169115=CARTESIAN_POINT('Ctrl Pts',(66.2923705569563,7.76273645738784,56.9018160669044));
#169116=CARTESIAN_POINT('Ctrl Pts',(65.9645120735511,7.47234456209885,56.9635291811305));
#169117=CARTESIAN_POINT('Ctrl Pts',(65.8863336212564,7.40081784720911,56.9782876158395));
#169118=CARTESIAN_POINT('Ctrl Pts',(65.7556739998463,7.27734528441009,57.0030475955759));
#169119=CARTESIAN_POINT('Ctrl Pts',(65.702603167529,7.22605357069181,57.0131318585195));
#169120=CARTESIAN_POINT('Ctrl Pts',(65.6274599925117,7.15177926468331,57.0274558840965));
#169121=CARTESIAN_POINT('Ctrl Pts',(65.6049212325227,7.12928424235837,57.0317582982299));
#169122=CARTESIAN_POINT('Ctrl Pts',(65.5659147023901,7.0899743725922,57.0392153422113));
#169123=CARTESIAN_POINT('Ctrl Pts',(65.5493980458749,7.07320966962676,57.0423764221574));
#169124=CARTESIAN_POINT('Ctrl Pts',(65.5141827325608,7.03720861808358,57.0491239349662));
#169125=CARTESIAN_POINT('Ctrl Pts',(65.4955021198739,7.01795468533027,57.0527079444153));
#169126=CARTESIAN_POINT('Ctrl Pts',(65.4445585189366,6.96501731238261,57.0624941354596));
#169127=CARTESIAN_POINT('Ctrl Pts',(65.41245347542,6.93117891323654,57.0686750931842));
#169128=CARTESIAN_POINT('Ctrl Pts',(65.2388941725803,6.7456338973516,57.1021584877965));
#169129=CARTESIAN_POINT('Ctrl Pts',(65.101948446706,6.58966703048029,57.1288306617375));
#169130=CARTESIAN_POINT('Ctrl Pts',(64.715974954414,6.12119937601435,57.2045269214451));
#169131=CARTESIAN_POINT('Ctrl Pts',(64.4806217066703,5.79761807739396,57.2513563251151));
#169132=CARTESIAN_POINT('Ctrl Pts',(64.0394473529066,5.10750264809855,57.3397137575542));
#169133=CARTESIAN_POINT('Ctrl Pts',(63.8359665871407,4.74035477580107,57.3807975050775));
#169134=CARTESIAN_POINT('Ctrl Pts',(63.6209177553964,4.28775468594752,57.4243679176016));
#169135=CARTESIAN_POINT('Ctrl Pts',(63.5869006210728,4.21386704673098,57.4312662880771));
#169136=CARTESIAN_POINT('Ctrl Pts',(63.5345098509273,4.09634855309728,57.4419001186997));
#169137=CARTESIAN_POINT('Ctrl Pts',(63.5155468574939,4.05299496798558,57.4457511486891));
#169138=CARTESIAN_POINT('Ctrl Pts',(63.4804355900086,3.97116021103539,57.4528855368321));
#169139=CARTESIAN_POINT('Ctrl Pts',(63.4642200661139,3.93271016472813,57.4561820861494));
#169140=CARTESIAN_POINT('Ctrl Pts',(63.4281854864458,3.84576416205288,57.4635116003861));
#169141=CARTESIAN_POINT('Ctrl Pts',(63.408503651082,3.79721041781361,57.4675176448319));
#169142=CARTESIAN_POINT('Ctrl Pts',(63.3501713437566,3.65003093824365,57.4793992832138));
#169143=CARTESIAN_POINT('Ctrl Pts',(63.3126866358481,3.55093299042886,57.4870463754278));
#169144=CARTESIAN_POINT('Ctrl Pts',(63.0121248439304,2.71696932840247,57.5484809650592));
#169145=CARTESIAN_POINT('Ctrl Pts',(62.8329579683888,1.95358456771351,57.5856285162755));
#169146=CARTESIAN_POINT('Ctrl Pts',(62.7095641700797,0.883623259656689,
57.6159490756503));
#169147=CARTESIAN_POINT('Ctrl Pts',(62.6885800130487,0.589144199610154,
57.6221186997156));
#169148=CARTESIAN_POINT('Ctrl Pts',(62.6789394557067,0.236476854729755,
57.627207924134));
#169149=CARTESIAN_POINT('Ctrl Pts',(62.6778570011712,0.178800735331424,
57.6279669991883));
#169150=CARTESIAN_POINT('Ctrl Pts',(62.6769860189733,0.0933820479571085,
57.6289857077668));
#169151=CARTESIAN_POINT('Ctrl Pts',(62.6768174887749,0.0656452109127856,
57.6293000326176));
#169152=CARTESIAN_POINT('Ctrl Pts',(62.6767385858228,0.0252719382420035,
57.6297339172685));
#169153=CARTESIAN_POINT('Ctrl Pts',(62.6767376164588,0.0126359830890657,
57.6298663430741));
#169154=CARTESIAN_POINT('Ctrl Pts',(62.6767603761739,-3.95693523589967E-11,
57.6299954198325));
#169155=CARTESIAN_POINT('Origin',(72.2537026314029,-4.33680868994202E-16,
54.3558290880045));
#169156=CARTESIAN_POINT('',(62.7943529015217,3.0501608000356E-11,58.2968957709606));
#169157=CARTESIAN_POINT('',(62.7896316916575,-2.89921316295001E-11,58.2701204592907));
#169158=CARTESIAN_POINT('',(62.4056251012807,-1.65832766814156E-15,56.0923108646735));
#169159=CARTESIAN_POINT('Ctrl Pts',(62.7943529015217,6.10048743283802E-11,
58.2968957709606));
#169160=CARTESIAN_POINT('Ctrl Pts',(62.7943293344815,0.0130842026143754,
58.2967621156339));
#169161=CARTESIAN_POINT('Ctrl Pts',(62.7943309036955,0.0261683656279026,
58.2966231335219));
#169162=CARTESIAN_POINT('Ctrl Pts',(62.7944147362689,0.0672353263688407,
58.2961702621673));
#169163=CARTESIAN_POINT('Ctrl Pts',(62.7945868500452,0.0952175476144742,
58.2958374185394));
#169164=CARTESIAN_POINT('Ctrl Pts',(62.7954790261329,0.182158258854861,
58.2947285382218));
#169165=CARTESIAN_POINT('Ctrl Pts',(62.7965947593984,0.241110378516977,
58.2938698386951));
#169166=CARTESIAN_POINT('Ctrl Pts',(62.8109561299922,0.761463163301568,
58.2853646196334));
#169167=CARTESIAN_POINT('Ctrl Pts',(62.8549919718124,1.2213647278526,58.2714431684893));
#169168=CARTESIAN_POINT('Ctrl Pts',(63.0289148515734,2.2744655743346,58.2265182963711));
#169169=CARTESIAN_POINT('Ctrl Pts',(63.1810736254434,2.86200269780546,58.191669630014));
#169170=CARTESIAN_POINT('Ctrl Pts',(63.4220714370871,3.53570538406769,58.1409193129469));
#169171=CARTESIAN_POINT('Ctrl Pts',(63.4609455944977,3.63898426690543,58.1328229898742));
#169172=CARTESIAN_POINT('Ctrl Pts',(63.5210776754935,3.79109434510471,58.1204277642212));
#169173=CARTESIAN_POINT('Ctrl Pts',(63.5410417054879,3.84044432826453,58.1163318334652));
#169174=CARTESIAN_POINT('Ctrl Pts',(63.5773843881548,3.92826654711039,58.1089093017307));
#169175=CARTESIAN_POINT('Ctrl Pts',(63.593613513274,3.96680124299856,58.1056061430119));
#169176=CARTESIAN_POINT('Ctrl Pts',(63.6285156588286,4.04824729677221,58.0985261637471));
#169177=CARTESIAN_POINT('Ctrl Pts',(63.6472487224153,4.09113100479396,58.0947399579927));
#169178=CARTESIAN_POINT('Ctrl Pts',(63.698377787519,4.20597898835893,58.0844423272796));
#169179=CARTESIAN_POINT('Ctrl Pts',(63.7313211842534,4.27768812336586,58.077845173602));
#169180=CARTESIAN_POINT('Ctrl Pts',(63.9189449681989,4.67370765463693,58.0404716424053));
#169181=CARTESIAN_POINT('Ctrl Pts',(64.0900305241596,4.98970407511549,58.0071314223973));
#169182=CARTESIAN_POINT('Ctrl Pts',(64.5050712194121,5.6666362814385,57.9273147193814));
#169183=CARTESIAN_POINT('Ctrl Pts',(64.7563347286539,6.02207380364771,57.8796449442551));
#169184=CARTESIAN_POINT('Ctrl Pts',(65.177562157959,6.5423027201162,57.7996877421493));
#169185=CARTESIAN_POINT('Ctrl Pts',(65.3318004113855,6.71957783593003,57.770397640488));
#169186=CARTESIAN_POINT('Ctrl Pts',(65.5249411939834,6.92632376194569,57.7335497497995));
#169187=CARTESIAN_POINT('Ctrl Pts',(65.5580849452905,6.96128937182639,57.7272207167366));
#169188=CARTESIAN_POINT('Ctrl Pts',(65.6103144474867,7.01559409779447,57.7172362668764));
#169189=CARTESIAN_POINT('Ctrl Pts',(65.6292310718141,7.03510161678302,57.713617878005));
#169190=CARTESIAN_POINT('Ctrl Pts',(65.6629829608783,7.06962348767211,57.7071575156229));
#169191=CARTESIAN_POINT('Ctrl Pts',(65.677787053521,7.08466913084751,57.7043224280844));
#169192=CARTESIAN_POINT('Ctrl Pts',(65.7136620417849,7.12089787138151,57.6974486524499));
#169193=CARTESIAN_POINT('Ctrl Pts',(65.7347797384007,7.14203225950021,57.6933995959993));
#169194=CARTESIAN_POINT('Ctrl Pts',(65.8006608754384,7.20737303200271,57.6807597907767));
#169195=CARTESIAN_POINT('Ctrl Pts',(65.8457426192756,7.25124273526741,57.6720992635608));
#169196=CARTESIAN_POINT('Ctrl Pts',(66.0790231114065,7.47396920349584,57.6272398867786));
#169197=CARTESIAN_POINT('Ctrl Pts',(66.273641838713,7.64567789291229,57.5896707955479));
#169198=CARTESIAN_POINT('Ctrl Pts',(66.9852626886022,8.22526528380116,57.4523596920884));
#169199=CARTESIAN_POINT('Ctrl Pts',(67.5354362690946,8.5881803337454,57.346430318815));
#169200=CARTESIAN_POINT('Ctrl Pts',(68.2295637926754,8.95152273838138,57.2148010286963));
#169201=CARTESIAN_POINT('Ctrl Pts',(68.3430123292046,9.00811476097755,57.1933418215872));
#169202=CARTESIAN_POINT('Ctrl Pts',(68.5041284454596,9.0845932463496,57.1629459012025));
#169203=CARTESIAN_POINT('Ctrl Pts',(68.5509168967525,9.10634851806559,57.15412814532));
#169204=CARTESIAN_POINT('Ctrl Pts',(68.6328905672464,9.14367379770937,57.1386956445957));
#169205=CARTESIAN_POINT('Ctrl Pts',(68.6680007905951,9.15940981475496,57.1320908966931));
#169206=CARTESIAN_POINT('Ctrl Pts',(68.7419714211186,9.192036972856,57.1181867589041));
#169207=CARTESIAN_POINT('Ctrl Pts',(68.7808503467378,9.20888312137265,57.1108849831111));
#169208=CARTESIAN_POINT('Ctrl Pts',(68.8744716352097,9.24872420912049,57.0933170042366));
#169209=CARTESIAN_POINT('Ctrl Pts',(68.9293148943754,9.27147192285284,57.0830378198933));
#169210=CARTESIAN_POINT('Ctrl Pts',(69.1222746074005,9.34944268669734,57.0469133533909));
#169211=CARTESIAN_POINT('Ctrl Pts',(69.2614260595878,9.40198714322001,57.0209371562456));
#169212=CARTESIAN_POINT('Ctrl Pts',(69.606914981838,9.52345520121727,56.9566090683839));
#169213=CARTESIAN_POINT('Ctrl Pts',(69.8144426648795,9.58866924081918,56.9181128988772));
#169214=CARTESIAN_POINT('Ctrl Pts',(70.3660865441529,9.74184751387493,56.8160554259573));
#169215=CARTESIAN_POINT('Ctrl Pts',(70.7130834328755,9.81795943782242,56.7521389818632));
#169216=CARTESIAN_POINT('Ctrl Pts',(71.4611692896431,9.93944803065652,56.6143037617848));
#169217=CARTESIAN_POINT('Ctrl Pts',(71.8624991917176,9.97913694636592,56.5403357430162));
#169218=CARTESIAN_POINT('Ctrl Pts',(72.3338195128043,9.99617727907689,56.4527018156264));
#169219=CARTESIAN_POINT('Ctrl Pts',(72.4026881310376,9.99793038223455,56.4398773694351));
#169220=CARTESIAN_POINT('Ctrl Pts',(72.498828970038,9.99934960489475,56.4219420978089));
#169221=CARTESIAN_POINT('Ctrl Pts',(72.5260938234216,9.99963669123889,56.4168521568661));
#169222=CARTESIAN_POINT('Ctrl Pts',(72.5752915408565,9.99994650746719,56.4076607194083));
#169223=CARTESIAN_POINT('Ctrl Pts',(72.597224265041,10.0000099567593,56.4035606085988));
#169224=CARTESIAN_POINT('Ctrl Pts',(72.6421217494904,9.99998698524796,56.3951621072308));
#169225=CARTESIAN_POINT('Ctrl Pts',(72.6650862724819,9.9998933663003,56.3908635256155));
#169226=CARTESIAN_POINT('Ctrl Pts',(72.724358031512,9.99944041524586,56.3797618043508));
#169227=CARTESIAN_POINT('Ctrl Pts',(72.7606632790489,9.99895828896922,56.3729549571492));
#169228=CARTESIAN_POINT('Ctrl Pts',(72.9160861014167,9.99601788440495,56.3437878713826));
#169229=CARTESIAN_POINT('Ctrl Pts',(73.0351460548074,9.99156084653281,56.3213770087204));
#169230=CARTESIAN_POINT('Ctrl Pts',(73.365918175375,9.97304476408488,56.2589742797523));
#169231=CARTESIAN_POINT('Ctrl Pts',(73.5772877629782,9.95421003460366,56.2189377542272));
#169232=CARTESIAN_POINT('Ctrl Pts',(74.5446760547878,9.83577703077049,56.0353602003182));
#169233=CARTESIAN_POINT('Ctrl Pts',(75.2882383596671,9.65380022996709,55.8935469931949));
#169234=CARTESIAN_POINT('Ctrl Pts',(76.1021830207998,9.34939493430575,55.7398984002603));
#169235=CARTESIAN_POINT('Ctrl Pts',(76.1999081944058,9.31103315447107,55.7214730661648));
#169236=CARTESIAN_POINT('Ctrl Pts',(76.3449530058481,9.25137097475403,55.6941602286289));
#169237=CARTESIAN_POINT('Ctrl Pts',(76.3927370477044,9.23126823608833,55.6851678015874));
#169238=CARTESIAN_POINT('Ctrl Pts',(76.4782612750357,9.19448216626113,55.6690830959504));
#169239=CARTESIAN_POINT('Ctrl Pts',(76.5160582416034,9.17793962010214,55.6619780861258));
#169240=CARTESIAN_POINT('Ctrl Pts',(76.5964565489322,9.14214199517785,55.6468723892491));
#169241=CARTESIAN_POINT('Ctrl Pts',(76.6390277839466,9.12281905823337,55.6388783511088));
#169242=CARTESIAN_POINT('Ctrl Pts',(76.7543073810453,9.06949133230654,55.6172429952161));
#169243=CARTESIAN_POINT('Ctrl Pts',(76.8267467978321,9.03489011645201,55.6036607149198));
#169244=CARTESIAN_POINT('Ctrl Pts',(77.2657555781029,8.81850531417105,55.521420489191));
#169245=CARTESIAN_POINT('Ctrl Pts',(77.6213831384325,8.61455960666906,55.4551361083359));
#169246=CARTESIAN_POINT('Ctrl Pts',(78.2850049499963,8.17656555069726,55.3315369244969));
#169247=CARTESIAN_POINT('Ctrl Pts',(78.5940060417588,7.94546023602887,55.2740240934562));
#169248=CARTESIAN_POINT('Ctrl Pts',(79.0606723178237,7.55162368283231,55.1865131385399));
#169249=CARTESIAN_POINT('Ctrl Pts',(79.2275311838521,7.40073428094589,55.1550728350098));
#169250=CARTESIAN_POINT('Ctrl Pts',(79.423277209432,7.21114332310874,55.1178636401614));
#169251=CARTESIAN_POINT('Ctrl Pts',(79.457168511617,7.17783958152459,55.1114088340873));
#169252=CARTESIAN_POINT('Ctrl Pts',(79.5099578575737,7.12520988486224,55.1013333215394));
#169253=CARTESIAN_POINT('Ctrl Pts',(79.5290174159989,7.10605110411441,55.0976911088358));
#169254=CARTESIAN_POINT('Ctrl Pts',(79.5628405344995,7.07177119001523,55.0912192771218));
#169255=CARTESIAN_POINT('Ctrl Pts',(79.5776342189003,7.05668099755745,55.0883856942888));
#169256=CARTESIAN_POINT('Ctrl Pts',(79.6133777293118,7.01998591484583,55.0815324063195));
#169257=CARTESIAN_POINT('Ctrl Pts',(79.6342779798912,6.99833188913727,55.0775192720024));
#169258=CARTESIAN_POINT('Ctrl Pts',(79.6993520310903,6.93029079258811,55.0650067299684));
#169259=CARTESIAN_POINT('Ctrl Pts',(79.7431778854462,6.88356457752861,55.056554470086));
#169260=CARTESIAN_POINT('Ctrl Pts',(79.9691590169313,6.63788276321501,55.012851795521));
#169261=CARTESIAN_POINT('Ctrl Pts',(80.1436651777642,6.43185179817786,54.9786944060639));
#169262=CARTESIAN_POINT('Ctrl Pts',(80.3847360351059,6.12249470125553,54.9311377423839));
#169263=CARTESIAN_POINT('Ctrl Pts',(80.4580475296599,6.02475451610943,54.9166201363671));
#169264=CARTESIAN_POINT('Ctrl Pts',(80.8639746050662,5.46229627324746,54.8359912114885));
#169265=CARTESIAN_POINT('Ctrl Pts',(81.1583945238756,4.97037240264469,54.7766231134293));
#169266=CARTESIAN_POINT('Ctrl Pts',(81.4498591380089,4.37300962317045,54.7176154916836));
#169267=CARTESIAN_POINT('Ctrl Pts',(81.4889241406627,4.29009331337702,54.7096985266908));
#169268=CARTESIAN_POINT('Ctrl Pts',(81.5493853819688,4.15708846364673,54.6974333486501));
#169269=CARTESIAN_POINT('Ctrl Pts',(81.5715111487678,4.10735064173061,54.6929421599415));
#169270=CARTESIAN_POINT('Ctrl Pts',(81.610026113258,4.01884891995319,54.685119365165));
#169271=CARTESIAN_POINT('Ctrl Pts',(81.6265763995364,3.9801594017487,54.681756161049));
#169272=CARTESIAN_POINT('Ctrl Pts',(81.6605962527342,3.89923597663324,54.6748394054917));
#169273=CARTESIAN_POINT('Ctrl Pts',(81.6780222419108,3.85698408309974,54.6712944060832));
#169274=CARTESIAN_POINT('Ctrl Pts',(81.7228403145991,3.7461886805504,54.6621714655065));
#169275=CARTESIAN_POINT('Ctrl Pts',(81.7497716814511,3.6774544648187,54.6566838692268));
#169276=CARTESIAN_POINT('Ctrl Pts',(81.8723984160978,3.3541031237216,54.6316682167266));
#169277=CARTESIAN_POINT('Ctrl Pts',(81.9585948862542,3.0958660756909,54.6140020814812));
#169278=CARTESIAN_POINT('Ctrl Pts',(82.1959543207427,2.27611767193012,54.5648906558562));
#169279=CARTESIAN_POINT('Ctrl Pts',(82.3094081381817,1.70455321714498,54.5407101351508));
#169280=CARTESIAN_POINT('Ctrl Pts',(82.4051349782228,0.836190511055383,
54.5168394758559));
#169281=CARTESIAN_POINT('Ctrl Pts',(82.4245618667854,0.544923089900452,
54.5109457745998));
#169282=CARTESIAN_POINT('Ctrl Pts',(82.4323856717708,0.208842427196565,
54.5062972627666));
#169283=CARTESIAN_POINT('Ctrl Pts',(82.4331260232878,0.164482173895023,
54.5057267287932));
#169284=CARTESIAN_POINT('Ctrl Pts',(82.4338528819693,0.0924989155547868,
54.5048692787617));
#169285=CARTESIAN_POINT('Ctrl Pts',(82.4340184471795,0.0648786374945988,
54.5045565971891));
#169286=CARTESIAN_POINT('Ctrl Pts',(82.4341117519754,0.0155095810496853,
54.50402648799));
#169287=CARTESIAN_POINT('Ctrl Pts',(82.4340825682918,-0.00623873017125077,
54.5038029233805));
#169288=CARTESIAN_POINT('Ctrl Pts',(82.4338637165141,-0.0540865559119959,
54.5033329252075));
#169289=CARTESIAN_POINT('Ctrl Pts',(82.4336431174273,-0.0801856147328861,
54.5030909120679));
#169290=CARTESIAN_POINT('Ctrl Pts',(82.4327104851214,-0.155825802968483,
54.5024316101472));
#169291=CARTESIAN_POINT('Ctrl Pts',(82.4317350194961,-0.205363242757256,
54.5020521751577));
#169292=CARTESIAN_POINT('Ctrl Pts',(82.419855199437,-0.644529275792791,
54.4991629057913));
#169293=CARTESIAN_POINT('Ctrl Pts',(82.3867795976834,-1.03325092763291,
54.4999298655147));
#169294=CARTESIAN_POINT('Ctrl Pts',(82.2347873349296,-2.0926359449325,54.5125266370394));
#169295=CARTESIAN_POINT('Ctrl Pts',(82.0706568649973,-2.75462038157244,
54.5322643312027));
#169296=CARTESIAN_POINT('Ctrl Pts',(81.8016976589154,-3.50690289598401,
54.5704295648089));
#169297=CARTESIAN_POINT('Ctrl Pts',(81.7596171380991,-3.61836617779735,
54.5765050728406));
#169298=CARTESIAN_POINT('Ctrl Pts',(81.6955103624837,-3.77951718314554,
54.5859068210986));
#169299=CARTESIAN_POINT('Ctrl Pts',(81.6750275000285,-3.82982511027735,
54.5889307125001));
#169300=CARTESIAN_POINT('Ctrl Pts',(81.6379481696952,-3.91883890119254,
54.5944393390176));
#169301=CARTESIAN_POINT('Ctrl Pts',(81.6215123252486,-3.9576121617823,54.5968925903749));
#169302=CARTESIAN_POINT('Ctrl Pts',(81.5866749558957,-4.03838963780071,
54.6021160251081));
#169303=CARTESIAN_POINT('Ctrl Pts',(81.5682291437554,-4.08037311971113,
54.6048949145853));
#169304=CARTESIAN_POINT('Ctrl Pts',(81.5191199552964,-4.19011629676324,
54.6123269809385));
#169305=CARTESIAN_POINT('Ctrl Pts',(81.4879960161064,-4.25766057610092,
54.6170705160356));
#169306=CARTESIAN_POINT('Ctrl Pts',(81.3346696993241,-4.58097316062581,
54.6405916395179));
#169307=CARTESIAN_POINT('Ctrl Pts',(81.2025488201186,-4.83174865825036,
54.6613157508934));
#169308=CARTESIAN_POINT('Ctrl Pts',(80.8848337654175,-5.37768182249967,
54.7119100517247));
#169309=CARTESIAN_POINT('Ctrl Pts',(80.6941551282675,-5.66935819423127,
54.7427551495191));
#169310=CARTESIAN_POINT('Ctrl Pts',(80.2677488282208,-6.25281247888802,
54.812092071968));
#169311=CARTESIAN_POINT('Ctrl Pts',(80.030029883529,-6.54241802822165,54.8509324155893));
#169312=CARTESIAN_POINT('Ctrl Pts',(79.729398638128,-6.86918597568535,54.8996853943373));
#169313=CARTESIAN_POINT('Ctrl Pts',(79.6815443567259,-6.92011125200681,
54.9074353950827));
#169314=CARTESIAN_POINT('Ctrl Pts',(79.6117819860961,-6.99279638261426,
54.9187133179158));
#169315=CARTESIAN_POINT('Ctrl Pts',(79.5902995076981,-7.01497071938764,
54.9221835250505));
#169316=CARTESIAN_POINT('Ctrl Pts',(79.5522621372452,-7.0538679235337,54.9283226737659));
#169317=CARTESIAN_POINT('Ctrl Pts',(79.5357502005065,-7.07063327665491,
54.9309859123285));
#169318=CARTESIAN_POINT('Ctrl Pts',(79.5000279104884,-7.10664637834109,
54.9367436990345));
#169319=CARTESIAN_POINT('Ctrl Pts',(79.480798068143,-7.1258738404656,54.939840833986));
#169320=CARTESIAN_POINT('Ctrl Pts',(79.4264072765182,-7.17981212388787,
54.9485948738223));
#169321=CARTESIAN_POINT('Ctrl Pts',(79.3910674668997,-7.21433757931758,
54.9542756243836));
#169322=CARTESIAN_POINT('Ctrl Pts',(79.1418332135287,-7.45421296459466,
54.9942981879214));
#169323=CARTESIAN_POINT('Ctrl Pts',(78.9191750005361,-7.65004089996804,
55.0298477965208));
#169324=CARTESIAN_POINT('Ctrl Pts',(78.5456971516658,-7.94991608812042,
55.0895301929499));
#169325=CARTESIAN_POINT('Ctrl Pts',(78.4000929857515,-8.06033423153442,
55.112809104865));
#169326=CARTESIAN_POINT('Ctrl Pts',(77.8449643651606,-8.45758730772135,
55.2017645334436));
#169327=CARTESIAN_POINT('Ctrl Pts',(77.4172790396777,-8.71700622504059,
55.2707390480504));
#169328=CARTESIAN_POINT('Ctrl Pts',(76.8779988768541,-8.99044595534622,
55.3588337402779));
#169329=CARTESIAN_POINT('Ctrl Pts',(76.782995899608,-9.03670711578353,55.3743908818577));
#169330=CARTESIAN_POINT('Ctrl Pts',(76.6401247635967,-9.10344911357804,
55.3978446687676));
#169331=CARTESIAN_POINT('Ctrl Pts',(76.5927939561801,-9.12510296840012,
55.4056238646237));
#169332=CARTESIAN_POINT('Ctrl Pts',(76.5075136666594,-9.16330172526239,
55.4196571761092));
#169333=CARTESIAN_POINT('Ctrl Pts',(76.4696255856313,-9.17998559055107,
55.4258977602181));
#169334=CARTESIAN_POINT('Ctrl Pts',(76.3886046501467,-9.21505247829252,
55.4392553398522));
#169335=CARTESIAN_POINT('Ctrl Pts',(76.3454441599627,-9.23336666764757,
55.4463785523404));
#169336=CARTESIAN_POINT('Ctrl Pts',(76.2279185402163,-9.28224467637531,
55.4657952017962));
#169337=CARTESIAN_POINT('Ctrl Pts',(76.1533138309441,-9.31220128856702,
55.4781426512809));
#169338=CARTESIAN_POINT('Ctrl Pts',(75.7204713969116,-9.47984949739519,
55.5499021176183));
#169339=CARTESIAN_POINT('Ctrl Pts',(75.3550051431997,-9.59721854715605,
55.6109876179549));
#169340=CARTESIAN_POINT('Ctrl Pts',(74.5475159396625,-9.80500481622996,
55.7465757420032));
#169341=CARTESIAN_POINT('Ctrl Pts',(74.1042568569665,-9.88685085552179,
55.8213983490645));
#169342=CARTESIAN_POINT('Ctrl Pts',(73.3746708383493,-9.96981270256432,
55.9440788354323));
#169343=CARTESIAN_POINT('Ctrl Pts',(73.0910954109453,-9.98953030366832,
55.9916394685481));
#169344=CARTESIAN_POINT('Ctrl Pts',(72.763363819548,-9.99792646581856,56.0461953891899));
#169345=CARTESIAN_POINT('Ctrl Pts',(72.7196999342711,-9.99875100568503,
56.0534554470616));
#169346=CARTESIAN_POINT('Ctrl Pts',(72.6488124556432,-9.99961233763443,
56.065226781678));
#169347=CARTESIAN_POINT('Ctrl Pts',(72.6215925147344,-9.99982886981166,
56.0697431882756));
#169348=CARTESIAN_POINT('Ctrl Pts',(72.5729163586274,-10.0000118731696,
56.0778127469671));
#169349=CARTESIAN_POINT('Ctrl Pts',(72.5514608518911,-10.000021597109,56.0813672247771));
#169350=CARTESIAN_POINT('Ctrl Pts',(72.5042304644808,-9.9998868466809,56.0891863598581));
#169351=CARTESIAN_POINT('Ctrl Pts',(72.478455856296,-9.99971094296779,56.0934499287059));
#169352=CARTESIAN_POINT('Ctrl Pts',(72.40368484573,-9.99890368887334,56.1058087321512));
#169353=CARTESIAN_POINT('Ctrl Pts',(72.3546906263827,-9.99800478995449,
56.1138949369193));
#169354=CARTESIAN_POINT('Ctrl Pts',(71.912449173706,-9.98655110407041,56.1867869673729));
#169355=CARTESIAN_POINT('Ctrl Pts',(71.5200327365673,-9.95254291377877,
56.2507850857573));
#169356=CARTESIAN_POINT('Ctrl Pts',(70.4483325154485,-9.79387743191931,
56.4251780552333));
#169357=CARTESIAN_POINT('Ctrl Pts',(69.7782597175951,-9.6207014238564,56.5339133418886));
#169358=CARTESIAN_POINT('Ctrl Pts',(69.0468560195961,-9.34638531395464,
56.653840627167));
#169359=CARTESIAN_POINT('Ctrl Pts',(68.9624800994791,-9.31339554115896,
56.6676920872827));
#169360=CARTESIAN_POINT('Ctrl Pts',(68.8285955541576,-9.25889269734186,
56.689697977193));
#169361=CARTESIAN_POINT('Ctrl Pts',(68.7787910001814,-9.23813602597271,
56.6978900881166));
#169362=CARTESIAN_POINT('Ctrl Pts',(68.6907696983954,-9.20059472937169,
56.7123788851772));
#169363=CARTESIAN_POINT('Ctrl Pts',(68.6524850944088,-9.18397607802619,
56.7186843296913));
#169364=CARTESIAN_POINT('Ctrl Pts',(68.5728256152086,-9.14879027356494,
56.7318115667791));
#169365=CARTESIAN_POINT('Ctrl Pts',(68.5314707345536,-9.13017931382513,
56.7386307051019));
#169366=CARTESIAN_POINT('Ctrl Pts',(68.4235923858018,-9.08072684503501,
56.7564298077484));
#169367=CARTESIAN_POINT('Ctrl Pts',(68.3572795579069,-9.04942268914026,
56.7673816508158));
#169368=CARTESIAN_POINT('Ctrl Pts',(68.0430277694203,-8.89673768247053,
56.8193296453327));
#169369=CARTESIAN_POINT('Ctrl Pts',(67.7998539091083,-8.76562020034719,
56.8596758587761));
#169370=CARTESIAN_POINT('Ctrl Pts',(66.9445219438104,-8.25676000969842,
57.0018635706515));
#169371=CARTESIAN_POINT('Ctrl Pts',(66.3681103195645,-7.82203377352227,
57.098363879586));
#169372=CARTESIAN_POINT('Ctrl Pts',(65.7902698355847,-7.27840340345619,
57.1926744948112));
#169373=CARTESIAN_POINT('Ctrl Pts',(65.738209353335,-7.22834704256752,57.2011454526931));
#169374=CARTESIAN_POINT('Ctrl Pts',(65.6657388188699,-7.15713548605935,
57.2128949691012));
#169375=CARTESIAN_POINT('Ctrl Pts',(65.6448796484374,-7.13645688375126,
57.216271787124));
#169376=CARTESIAN_POINT('Ctrl Pts',(65.6072517692323,-7.09882403141038,
57.2223535670278));
#169377=CARTESIAN_POINT('Ctrl Pts',(65.5904524614216,-7.08190171507522,
57.225065298698));
#169378=CARTESIAN_POINT('Ctrl Pts',(65.555800035577,-7.0467446771676,57.2306512449039));
#169379=CARTESIAN_POINT('Ctrl Pts',(65.5379557776114,-7.02850129585407,
57.2335235256053));
#169380=CARTESIAN_POINT('Ctrl Pts',(65.4911266166101,-6.98025630619024,
57.2410506583338));
#169381=CARTESIAN_POINT('Ctrl Pts',(65.4622573624889,-6.95013918773834,
57.2456801258759));
#169382=CARTESIAN_POINT('Ctrl Pts',(65.3279843769467,-6.80829484557587,
57.2671643013652));
#169383=CARTESIAN_POINT('Ctrl Pts',(65.2249381522968,-6.69428815491473,
57.28351301364));
#169384=CARTESIAN_POINT('Ctrl Pts',(64.9177665496709,-6.33828239680599,
57.3319147019146));
#169385=CARTESIAN_POINT('Ctrl Pts',(64.7223443702513,-6.08880373248865,
57.3622400323581));
#169386=CARTESIAN_POINT('Ctrl Pts',(64.233832824973,-5.4002286631775,57.4373804728273));
#169387=CARTESIAN_POINT('Ctrl Pts',(63.962819096328,-4.9462924518367,57.478369650224));
#169388=CARTESIAN_POINT('Ctrl Pts',(63.6816093985632,-4.37782800872695,
57.5206809355739));
#169389=CARTESIAN_POINT('Ctrl Pts',(63.63612695229,-4.28210804313245,57.5275134601793));
#169390=CARTESIAN_POINT('Ctrl Pts',(63.5704181624404,-4.1379889507939,57.5373696743691));
#169391=CARTESIAN_POINT('Ctrl Pts',(63.549048462097,-4.0901317839848,57.5405725753773));
#169392=CARTESIAN_POINT('Ctrl Pts',(63.5113156045274,-4.00382490312059,
57.5462234718173));
#169393=CARTESIAN_POINT('Ctrl Pts',(63.4948166842198,-3.96543729475209,
57.5486927316391));
#169394=CARTESIAN_POINT('Ctrl Pts',(63.4601033267713,-3.88326428312749,
57.553884451202));
#169395=CARTESIAN_POINT('Ctrl Pts',(63.4419580261639,-3.83945010877777,
57.556596086404));
#169396=CARTESIAN_POINT('Ctrl Pts',(63.3934465691909,-3.71993188910788,
57.5638394750176));
#169397=CARTESIAN_POINT('Ctrl Pts',(63.3636874357562,-3.64397971588759,
57.568276099263));
#169398=CARTESIAN_POINT('Ctrl Pts',(63.1950020529328,-3.19757304992833,
57.5933796870426));
#169399=CARTESIAN_POINT('Ctrl Pts',(63.0770087644234,-2.81940685612739,
57.6107719970196));
#169400=CARTESIAN_POINT('Ctrl Pts',(62.864374307043,-1.96433397259502,57.641195723081));
#169401=CARTESIAN_POINT('Ctrl Pts',(62.7812741321484,-1.48552760680555,
57.6523290080425));
#169402=CARTESIAN_POINT('Ctrl Pts',(62.7077436067178,-0.754835660743466,
57.6593095160525));
#169403=CARTESIAN_POINT('Ctrl Pts',(62.6919146816398,-0.506288995406827,
57.6599513901734));
#169404=CARTESIAN_POINT('Ctrl Pts',(62.6838799958966,-0.208933603431457,
57.658479443963));
#169405=CARTESIAN_POINT('Ctrl Pts',(62.6829155563255,-0.160440203136994,
57.6581682739325));
#169406=CARTESIAN_POINT('Ctrl Pts',(62.682036687821,-0.0915736068739256,
57.6576237272076));
#169407=CARTESIAN_POINT('Ctrl Pts',(62.6818376927526,-0.0712042632457356,
57.6574499112884));
#169408=CARTESIAN_POINT('Ctrl Pts',(62.6815847637954,-0.0338865066335313,
57.6571079514006));
#169409=CARTESIAN_POINT('Ctrl Pts',(62.6815121129508,-0.0169482591708172,
57.6569438582266));
#169410=CARTESIAN_POINT('Ctrl Pts',(62.6814815860384,1.77731069449741E-12,
57.6567707315033));
#169411=CARTESIAN_POINT('Ctrl Pts',(62.6767603761739,-3.95693523589967E-11,
57.6299954198325));
#169412=CARTESIAN_POINT('Ctrl Pts',(62.6767730501235,-0.00703645950903762,
57.6300672973722));
#169413=CARTESIAN_POINT('Ctrl Pts',(62.6767930822822,-0.0140729276535245,
57.6301381363992));
#169414=CARTESIAN_POINT('Ctrl Pts',(62.6769183030972,-0.0462422506144614,
57.6304572342398));
#169415=CARTESIAN_POINT('Ctrl Pts',(62.6771099999868,-0.0713747770162598,
57.6306932376319));
#169416=CARTESIAN_POINT('Ctrl Pts',(62.6778933222357,-0.140320776548243,
57.6313037681363));
#169417=CARTESIAN_POINT('Ctrl Pts',(62.6786763049084,-0.184131765194433,
57.6316508424258));
#169418=CARTESIAN_POINT('Ctrl Pts',(62.6843188444241,-0.415569757892112,
57.6332640333996));
#169419=CARTESIAN_POINT('Ctrl Pts',(62.6941211343586,-0.603044268526511,
57.6338051878891));
#169420=CARTESIAN_POINT('Ctrl Pts',(62.7549097502567,-1.36086732614974,
57.6326472034358));
#169421=CARTESIAN_POINT('Ctrl Pts',(62.8490070080706,-1.92666111061175,
57.6240183363885));
#169422=CARTESIAN_POINT('Ctrl Pts',(63.0842531293513,-2.8508970654349,57.5948732928638));
#169423=CARTESIAN_POINT('Ctrl Pts',(63.1990431153161,-3.21478480939138,
57.5793227096225));
#169424=CARTESIAN_POINT('Ctrl Pts',(63.3626097339909,-3.64683809530257,
57.5556861018641));
#169425=CARTESIAN_POINT('Ctrl Pts',(63.3921566667552,-3.72214948882659,
57.5513703062038));
#169426=CARTESIAN_POINT('Ctrl Pts',(63.4403925355549,-3.84089455160905,
57.5442538557541));
#169427=CARTESIAN_POINT('Ctrl Pts',(63.4584916697803,-3.88457080459729,
57.5415687923236));
#169428=CARTESIAN_POINT('Ctrl Pts',(63.4931688744478,-3.96662345095016,
57.5363969656386));
#169429=CARTESIAN_POINT('Ctrl Pts',(63.5096803785325,-4.00502768472232,
57.5339232427941));
#169430=CARTESIAN_POINT('Ctrl Pts',(63.5475184818785,-4.0915546575601,57.5282296993175));
#169431=CARTESIAN_POINT('Ctrl Pts',(63.5689828992801,-4.13961397596239,
57.5249828223105));
#169432=CARTESIAN_POINT('Ctrl Pts',(63.6352761143501,-4.28498869449471,
57.514904388037));
#169433=CARTESIAN_POINT('Ctrl Pts',(63.6812708393281,-4.3817478663855,57.5078441781412));
#169434=CARTESIAN_POINT('Ctrl Pts',(63.9435144839838,-4.91153746887167,
57.4672430703019));
#169435=CARTESIAN_POINT('Ctrl Pts',(64.1889419365388,-5.32895121696058,
57.4279643259112));
#169436=CARTESIAN_POINT('Ctrl Pts',(64.5757289448318,-5.88982000550573,
57.3652675553829));
#169437=CARTESIAN_POINT('Ctrl Pts',(64.6930072265174,-6.04952765619241,
57.3461782181847));
#169438=CARTESIAN_POINT('Ctrl Pts',(64.999649469371,-6.44208536917183,57.2962298659326));
#169439=CARTESIAN_POINT('Ctrl Pts',(65.1948499843389,-6.66999768867731,
57.2644001494803));
#169440=CARTESIAN_POINT('Ctrl Pts',(65.4338351124456,-6.92473448219735,
57.2256963327324));
#169441=CARTESIAN_POINT('Ctrl Pts',(65.4679825907577,-6.96059109360578,
57.2201721467679));
#169442=CARTESIAN_POINT('Ctrl Pts',(65.5213116107772,-7.01575626599036,
57.2115561379527));
#169443=CARTESIAN_POINT('Ctrl Pts',(65.540308519357,-7.03524604937448,57.2084891151116));
#169444=CARTESIAN_POINT('Ctrl Pts',(65.5758763149472,-7.07143727984411,
57.2027511984484));
#169445=CARTESIAN_POINT('Ctrl Pts',(65.5924269566033,-7.08815851063107,
57.2000830106152));
#169446=CARTESIAN_POINT('Ctrl Pts',(65.6308083503078,-7.12666035101376,
57.1938994484052));
#169447=CARTESIAN_POINT('Ctrl Pts',(65.6526810550493,-7.14839782912533,
57.1903785321577));
#169448=CARTESIAN_POINT('Ctrl Pts',(65.7243038983775,-7.21891656845933,
57.1788578299424));
#169449=CARTESIAN_POINT('Ctrl Pts',(65.7744626176174,-7.26727090969583,
57.1708031559143));
#169450=CARTESIAN_POINT('Ctrl Pts',(66.0837652592173,-7.55921828299814,
57.121195528919));
#169451=CARTESIAN_POINT('Ctrl Pts',(66.355212885337,-7.78910569840687,57.0779099055449));
#169452=CARTESIAN_POINT('Ctrl Pts',(66.8719892920037,-8.18105325811043,
56.9952505071063));
#169453=CARTESIAN_POINT('Ctrl Pts',(67.1133916303522,-8.34776397214705,
56.9565481634264));
#169454=CARTESIAN_POINT('Ctrl Pts',(67.5564042013422,-8.62543564657457,
56.8851046338728));
#169455=CARTESIAN_POINT('Ctrl Pts',(67.7552235805904,-8.74057935349551,
56.852902466124));
#169456=CARTESIAN_POINT('Ctrl Pts',(68.0899909044745,-8.91913077708268,
56.798386878696));
#169457=CARTESIAN_POINT('Ctrl Pts',(68.2237471176902,-8.98659394378869,
56.7765312617136));
#169458=CARTESIAN_POINT('Ctrl Pts',(68.4142150470329,-9.07726312014421,
56.745298513356));
#169459=CARTESIAN_POINT('Ctrl Pts',(68.4697173717242,-9.10305075499764,
56.7361843887784));
#169460=CARTESIAN_POINT('Ctrl Pts',(68.5640628649491,-9.14581825546213,
56.7206698024296));
#169461=CARTESIAN_POINT('Ctrl Pts',(68.6027852011337,-9.16306992197531,
56.7142959327222));
#169462=CARTESIAN_POINT('Ctrl Pts',(68.6812299869732,-9.19741154696185,
56.7013710800815));
#169463=CARTESIAN_POINT('Ctrl Pts',(68.7209559650063,-9.21449079724056,
56.6948192636759));
#169464=CARTESIAN_POINT('Ctrl Pts',(68.8191397166746,-9.25593565058751,
56.6786105951197));
#169465=CARTESIAN_POINT('Ctrl Pts',(68.8777191853321,-9.27999710972145,
56.6689263726862));
#169466=CARTESIAN_POINT('Ctrl Pts',(69.0997492156598,-9.36869139438358,
56.6321705461046));
#169467=CARTESIAN_POINT('Ctrl Pts',(69.2646475548105,-9.42947187737469,
56.6047695197724));
#169468=CARTESIAN_POINT('Ctrl Pts',(69.6916485949808,-9.57392626757734,
56.5335836406093));
#169469=CARTESIAN_POINT('Ctrl Pts',(69.9557365363162,-9.65101383200898,
56.4893352656871));
#169470=CARTESIAN_POINT('Ctrl Pts',(70.8356014495849,-9.86796891442351,
56.3414929518335));
#169471=CARTESIAN_POINT('Ctrl Pts',(71.4613113241799,-9.9591250245189,56.2356092294406));
#169472=CARTESIAN_POINT('Ctrl Pts',(72.1876940817472,-9.99361605449846,
56.1142743013188));
#169473=CARTESIAN_POINT('Ctrl Pts',(72.283925344515,-9.99675471409284,56.0982338824842));
#169474=CARTESIAN_POINT('Ctrl Pts',(72.4149306511492,-9.99908189827062,
56.0764566003539));
#169475=CARTESIAN_POINT('Ctrl Pts',(72.449671653634,-9.9995129522664,56.0706872254942));
#169476=CARTESIAN_POINT('Ctrl Pts',(72.5048409769384,-9.9999020204515,56.0615351398569));
#169477=CARTESIAN_POINT('Ctrl Pts',(72.5252675186006,-9.99998176874114,
56.0581486930192));
#169478=CARTESIAN_POINT('Ctrl Pts',(72.5678229536413,-10.0000139510908,
56.0510982084332));
#169479=CARTESIAN_POINT('Ctrl Pts',(72.5899517234821,-9.9999552273227,56.0474345980703));
#169480=CARTESIAN_POINT('Ctrl Pts',(72.6441556196297,-9.99962655807334,
56.0384668595446));
#169481=CARTESIAN_POINT('Ctrl Pts',(72.6762305024331,-9.99927353800509,
56.0331655474039));
#169482=CARTESIAN_POINT('Ctrl Pts',(72.7931227708354,-9.99740923360215,
56.0138637553239));
#169483=CARTESIAN_POINT('Ctrl Pts',(72.8779265259183,-9.99494796000027,
55.9998952290557));
#169484=CARTESIAN_POINT('Ctrl Pts',(73.4095317892232,-9.97256441822664,
55.9125101387846));
#169485=CARTESIAN_POINT('Ctrl Pts',(73.8547227937369,-9.92299041826608,
55.8400988035389));
#169486=CARTESIAN_POINT('Ctrl Pts',(74.8528913103704,-9.74166578596338,
55.6778068135957));
#169487=CARTESIAN_POINT('Ctrl Pts',(75.4010864551881,-9.59185145428424,
55.5886793896532));
#169488=CARTESIAN_POINT('Ctrl Pts',(76.0374947437299,-9.35677851018121,
55.4843722946892));
#169489=CARTESIAN_POINT('Ctrl Pts',(76.1408954633519,-9.31657285902152,
55.467400478894));
#169490=CARTESIAN_POINT('Ctrl Pts',(76.2927394307979,-9.25453735573563,
55.4424399376539));
#169491=CARTESIAN_POINT('Ctrl Pts',(76.3417150974251,-9.23406188663135,
55.4343833679096));
#169492=CARTESIAN_POINT('Ctrl Pts',(76.4286843997551,-9.19686817249914,
55.4200664881765));
#169493=CARTESIAN_POINT('Ctrl Pts',(76.4667416996277,-9.1803053120177,55.4137979545817));
#169494=CARTESIAN_POINT('Ctrl Pts',(76.5469888009104,-9.14477244002966,
55.4005728193999));
#169495=CARTESIAN_POINT('Ctrl Pts',(76.5891523047892,-9.12574425336534,
55.3936197031896));
#169496=CARTESIAN_POINT('Ctrl Pts',(76.7016163445618,-9.07402759935329,
55.3750620831016));
#169497=CARTESIAN_POINT('Ctrl Pts',(76.7716706835233,-9.04080000370248,
55.363490486311));
#169498=CARTESIAN_POINT('Ctrl Pts',(77.1479219861643,-8.85683837482425,
55.3012808761437));
#169499=CARTESIAN_POINT('Ctrl Pts',(77.4466151464932,-8.69095536332824,
55.251666818673));
#169500=CARTESIAN_POINT('Ctrl Pts',(77.9198684905862,-8.3948719008566,55.1729311343635));
#169501=CARTESIAN_POINT('Ctrl Pts',(78.099723584724,-8.27391124224535,55.1429790993635));
#169502=CARTESIAN_POINT('Ctrl Pts',(78.6302781537059,-7.89111577955463,
55.0547332519268));
#169503=CARTESIAN_POINT('Ctrl Pts',(78.9679416977988,-7.61163695975409,
54.998706525971));
#169504=CARTESIAN_POINT('Ctrl Pts',(79.3353174715195,-7.26424259857941,
54.938789279341));
#169505=CARTESIAN_POINT('Ctrl Pts',(79.383741018466,-7.21751477357013,54.9309146061299));
#169506=CARTESIAN_POINT('Ctrl Pts',(79.4536984442701,-7.14862654645227,
54.9195766008154));
#169507=CARTESIAN_POINT('Ctrl Pts',(79.4756014835507,-7.12685710512131,
54.9160323879038));
#169508=CARTESIAN_POINT('Ctrl Pts',(79.5140174351064,-7.08831954481476,
54.9098266532962));
#169509=CARTESIAN_POINT('Ctrl Pts',(79.5305719591037,-7.0715948130502,54.9071559190606));
#169510=CARTESIAN_POINT('Ctrl Pts',(79.5661251393491,-7.03542133399335,
54.9014278543103));
#169511=CARTESIAN_POINT('Ctrl Pts',(79.5851040282734,-7.0159530104727,54.8983748560151));
#169512=CARTESIAN_POINT('Ctrl Pts',(79.6383277509734,-6.96090901401687,
54.8898259702292));
#169513=CARTESIAN_POINT('Ctrl Pts',(79.6723917784638,-6.92515347902827,
54.8843696385213));
#169514=CARTESIAN_POINT('Ctrl Pts',(79.908219719632,-6.67391241297142,54.8466928559278));
#169515=CARTESIAN_POINT('Ctrl Pts',(80.1007629886276,-6.44967898789775,
54.8164323098566));
#169516=CARTESIAN_POINT('Ctrl Pts',(80.3753692817547,-6.09963621108647,
54.7737250646285));
#169517=CARTESIAN_POINT('Ctrl Pts',(80.4649169703354,-5.98007951967056,
54.7598797984591));
#169518=CARTESIAN_POINT('Ctrl Pts',(80.8667413674399,-5.41781870523989,
54.698029213528));
#169519=CARTESIAN_POINT('Ctrl Pts',(81.1457710342195,-4.95184374073563,
54.655829943058));
#169520=CARTESIAN_POINT('Ctrl Pts',(81.4315238242444,-4.37297496881559,
54.6128386239359));
#169521=CARTESIAN_POINT('Ctrl Pts',(81.4756575606616,-4.28000185518985,
54.6062089315844));
#169522=CARTESIAN_POINT('Ctrl Pts',(81.5401421580115,-4.13859566780366,
54.5965362729525));
#169523=CARTESIAN_POINT('Ctrl Pts',(81.5615490161417,-4.09066325865285,
54.5933277826855));
#169524=CARTESIAN_POINT('Ctrl Pts',(81.5993227252462,-4.00427456710424,
54.5876707390799));
#169525=CARTESIAN_POINT('Ctrl Pts',(81.6158264466846,-3.96588089874698,
54.5852007478941));
#169526=CARTESIAN_POINT('Ctrl Pts',(81.6505251769789,-3.88375331949801,
54.5800111886631));
#169527=CARTESIAN_POINT('Ctrl Pts',(81.668651849627,-3.83999097759006,54.5773023198099));
#169528=CARTESIAN_POINT('Ctrl Pts',(81.7170541125251,-3.72076351979598,
54.5700751788798));
#169529=CARTESIAN_POINT('Ctrl Pts',(81.746727711641,-3.64505228686216,54.5656512469584));
#169530=CARTESIAN_POINT('Ctrl Pts',(81.9133955697007,-3.20417084113407,
54.5408473783303));
#169531=CARTESIAN_POINT('Ctrl Pts',(82.0300710656479,-2.83150713910028,
54.523646427459));
#169532=CARTESIAN_POINT('Ctrl Pts',(82.2398850257726,-1.99423984355841,
54.4935909311738));
#169533=CARTESIAN_POINT('Ctrl Pts',(82.3225606237439,-1.52792548356179,
54.4824555261108));
#169534=CARTESIAN_POINT('Ctrl Pts',(82.3729798775079,-1.05279654130084,
54.4774256716504));
#169535=CARTESIAN_POINT('Ctrl Pts',(82.3734724356883,-1.04812404505824,
54.4773768217422));
#169536=CARTESIAN_POINT('Ctrl Pts',(82.4016060224843,-0.779458804999393,
54.4746033673291));
#169537=CARTESIAN_POINT('Ctrl Pts',(82.4189096750665,-0.514469882601093,
54.4738294657436));
#169538=CARTESIAN_POINT('Ctrl Pts',(82.4270068078351,-0.205490529190298,
54.4754107223865));
#169539=CARTESIAN_POINT('Ctrl Pts',(82.4278702324258,-0.161859226207651,
54.4756916412848));
#169540=CARTESIAN_POINT('Ctrl Pts',(82.4288204927573,-0.090823488374513,
54.4762442007747));
#169541=CARTESIAN_POINT('Ctrl Pts',(82.4290767380085,-0.0634216294130038,
54.476480406394));
#169542=CARTESIAN_POINT('Ctrl Pts',(82.4293385200686,-0.0142810983463323,
54.4769457332704));
#169543=CARTESIAN_POINT('Ctrl Pts',(82.4293849340598,0.00745710382980186,
54.4771662470542));
#169544=CARTESIAN_POINT('Ctrl Pts',(82.4293341863736,0.0554785326590305,
54.477685826653));
#169545=CARTESIAN_POINT('Ctrl Pts',(82.4292049693798,0.08176129124716,54.4779916296242));
#169546=CARTESIAN_POINT('Ctrl Pts',(82.4285316766892,0.158468487834349,
54.4789461576016));
#169547=CARTESIAN_POINT('Ctrl Pts',(82.4277155479953,0.208889019182937,
54.4796518192819));
#169548=CARTESIAN_POINT('Ctrl Pts',(82.4159105354718,0.70906493129357,54.4874161870165));
#169549=CARTESIAN_POINT('Ctrl Pts',(82.3755609864959,1.15752836349655,54.5004882693197));
#169550=CARTESIAN_POINT('Ctrl Pts',(82.2068610916447,2.22875953212481,54.5447081719204));
#169551=CARTESIAN_POINT('Ctrl Pts',(82.0494635512867,2.84478283087259,54.5809129284911));
#169552=CARTESIAN_POINT('Ctrl Pts',(81.7988418525356,3.54316768347523,54.6336528733453));
#169553=CARTESIAN_POINT('Ctrl Pts',(81.7606646779194,3.64438470872402,54.6416005012898));
#169554=CARTESIAN_POINT('Ctrl Pts',(81.7014303815819,3.79406607834721,54.6538080178078));
#169555=CARTESIAN_POINT('Ctrl Pts',(81.681607237855,3.84302578750983,54.657874339003));
#169556=CARTESIAN_POINT('Ctrl Pts',(81.6454187762078,3.93041684719629,54.6652643942841));
#169557=CARTESIAN_POINT('Ctrl Pts',(81.6291974172002,3.96890834370733,54.6685655588056));
#169558=CARTESIAN_POINT('Ctrl Pts',(81.5941956370286,4.05053645526604,54.6756649093197));
#169559=CARTESIAN_POINT('Ctrl Pts',(81.5753514938876,4.09364376750275,54.6794730565798));
#169560=CARTESIAN_POINT('Ctrl Pts',(81.5236156664912,4.20976142294565,54.6898913538235));
#169561=CARTESIAN_POINT('Ctrl Pts',(81.490154893451,4.28250630447755,54.696590631967));
#169562=CARTESIAN_POINT('Ctrl Pts',(81.2907477346504,4.70269672627653,54.7363000769308));
#169563=CARTESIAN_POINT('Ctrl Pts',(81.1058777324296,5.04051428627442,54.7722656345596));
#169564=CARTESIAN_POINT('Ctrl Pts',(80.7241133451485,5.65166074140487,54.8455535455307));
#169565=CARTESIAN_POINT('Ctrl Pts',(80.531901771641,5.92736136981478,54.8820932826333));
#169566=CARTESIAN_POINT('Ctrl Pts',(80.1413555983125,6.43134801659066,54.9562323536256));
#169567=CARTESIAN_POINT('Ctrl Pts',(79.9457641775941,6.66135402728018,54.9933232199854));
#169568=CARTESIAN_POINT('Ctrl Pts',(79.7057435020128,6.91893325193734,55.0391076960068));
#169569=CARTESIAN_POINT('Ctrl Pts',(79.6709871232328,6.95566642586564,55.045743818865));
#169570=CARTESIAN_POINT('Ctrl Pts',(79.6167601621197,7.01210909655683,55.0561092813358));
#169571=CARTESIAN_POINT('Ctrl Pts',(79.5974809254804,7.03200889466407,55.0597967666537));
#169572=CARTESIAN_POINT('Ctrl Pts',(79.5617772468385,7.06855487408178,55.0666302994487));
#169573=CARTESIAN_POINT('Ctrl Pts',(79.545376418575,7.08522452647522,55.0697711545597));
#169574=CARTESIAN_POINT('Ctrl Pts',(79.5074829122929,7.12346818551903,55.0770320322302));
#169575=CARTESIAN_POINT('Ctrl Pts',(79.4859504863666,7.14500065226707,55.0811608488297));
#169576=CARTESIAN_POINT('Ctrl Pts',(79.4174480730519,7.21287585899812,55.0943044366918));
#169577=CARTESIAN_POINT('Ctrl Pts',(79.3701224699737,7.25884203766398,55.1033971158815));
#169578=CARTESIAN_POINT('Ctrl Pts',(79.1141926749848,7.50250369588973,55.1526190067117));
#169579=CARTESIAN_POINT('Ctrl Pts',(78.8976913879561,7.69136418084092,55.1944298746371));
#169580=CARTESIAN_POINT('Ctrl Pts',(78.2838825101048,8.18129732708011,55.3128506456284));
#169581=CARTESIAN_POINT('Ctrl Pts',(77.8717753589995,8.46179792821496,55.3921978488658));
#169582=CARTESIAN_POINT('Ctrl Pts',(77.2462945219386,8.82100363719068,55.511396839619));
#169583=CARTESIAN_POINT('Ctrl Pts',(77.0483720389228,8.92577871084782,55.5489582229632));
#169584=CARTESIAN_POINT('Ctrl Pts',(76.783487209225,9.05451937528056,55.5989921319597));
#169585=CARTESIAN_POINT('Ctrl Pts',(76.7195603847006,9.0847328878724,55.611049850424));
#169586=CARTESIAN_POINT('Ctrl Pts',(76.6147074934559,9.13289832527706,55.6307983198773));
#169587=CARTESIAN_POINT('Ctrl Pts',(76.5739730013242,9.15127139462957,55.6384634717442));
#169588=CARTESIAN_POINT('Ctrl Pts',(76.4949112294838,9.18627816191814,55.6533273409854));
#169589=CARTESIAN_POINT('Ctrl Pts',(76.4566001647601,9.20294698566827,55.6605238815318));
#169590=CARTESIAN_POINT('Ctrl Pts',(76.3667529918049,9.24135197633555,55.6773871338504));
#169591=CARTESIAN_POINT('Ctrl Pts',(76.3151360383591,9.26289062336812,55.6870642553344));
#169592=CARTESIAN_POINT('Ctrl Pts',(76.1453233088867,9.33203509825228,55.7188659577552));
#169593=CARTESIAN_POINT('Ctrl Pts',(76.0263920632102,9.37775573475257,55.7410838746758));
#169594=CARTESIAN_POINT('Ctrl Pts',(75.4832938997748,9.57436478447919,55.842311186214));
#169595=CARTESIAN_POINT('Ctrl Pts',(75.0500308355795,9.69791212482701,55.9224049916045));
#169596=CARTESIAN_POINT('Ctrl Pts',(74.0737754918058,9.90416761000369,56.102387699057));
#169597=CARTESIAN_POINT('Ctrl Pts',(73.5291952782041,9.97170823125382,56.2024549930993));
#169598=CARTESIAN_POINT('Ctrl Pts',(72.9079695672571,9.99567491006911,56.3179217619057));
#169599=CARTESIAN_POINT('Ctrl Pts',(72.8337804531382,9.99768193755017,56.3317334082451));
#169600=CARTESIAN_POINT('Ctrl Pts',(72.728284389981,9.99932051509322,56.3514113699516));
#169601=CARTESIAN_POINT('Ctrl Pts',(72.6969865941856,9.99965457759026,56.3572540338713));
#169602=CARTESIAN_POINT('Ctrl Pts',(72.6439812619526,9.99996283038682,56.3671576897605));
#169603=CARTESIAN_POINT('Ctrl Pts',(72.6222738843087,10.0000159269599,56.3712160098394));
#169604=CARTESIAN_POINT('Ctrl Pts',(72.5772235176491,9.99997431923388,56.3796437543126));
#169605=CARTESIAN_POINT('Ctrl Pts',(72.5538808387964,9.99986817156351,56.3840134947001));
#169606=CARTESIAN_POINT('Ctrl Pts',(72.49251572356,9.99936673317937,56.3955083835053));
#169607=CARTESIAN_POINT('Ctrl Pts',(72.4544956172965,9.99883157127421,56.4026377265703));
#169608=CARTESIAN_POINT('Ctrl Pts',(72.2802833109216,9.99535057011472,56.4353365744532));
#169609=CARTESIAN_POINT('Ctrl Pts',(72.1441718469965,9.98974876820901,56.4609719204842));
#169610=CARTESIAN_POINT('Ctrl Pts',(71.7473587831863,9.96500015591874,56.5358905291706));
#169611=CARTESIAN_POINT('Ctrl Pts',(71.4872686788627,9.93814623553098,56.5852240625654));
#169612=CARTESIAN_POINT('Ctrl Pts',(70.580079533466,9.80709571539761,56.7575561715957));
#169613=CARTESIAN_POINT('Ctrl Pts',(69.9424640444626,9.64765091616599,56.8790159863435));
#169614=CARTESIAN_POINT('Ctrl Pts',(69.2054819054799,9.38166958775962,57.0182529712163));
#169615=CARTESIAN_POINT('Ctrl Pts',(69.0867697975335,9.3361763624801,57.0406491832489));
#169616=CARTESIAN_POINT('Ctrl Pts',(68.921054706971,9.26891833849636,57.0718657071906));
#169617=CARTESIAN_POINT('Ctrl Pts',(68.8733093509438,9.2490959576013,57.0808541581039));
#169618=CARTESIAN_POINT('Ctrl Pts',(68.790284730528,9.21384936594005,57.0964745278537));
#169619=CARTESIAN_POINT('Ctrl Pts',(68.7549373319765,9.1985954515273,57.103121750187));
#169620=CARTESIAN_POINT('Ctrl Pts',(68.6809070411261,9.1661266111272,57.1170370300208));
#169621=CARTESIAN_POINT('Ctrl Pts',(68.6422433720346,9.14886803357578,57.1243008328644));
#169622=CARTESIAN_POINT('Ctrl Pts',(68.5497815480908,9.10687096911078,57.1416630629036));
#169623=CARTESIAN_POINT('Ctrl Pts',(68.4960901972944,9.08189174982622,57.1517379490642));
#169624=CARTESIAN_POINT('Ctrl Pts',(68.3088635341918,8.9927051785819,57.1868461008762));
#169625=CARTESIAN_POINT('Ctrl Pts',(68.176525944269,8.92592930494475,57.2116183926266));
#169626=CARTESIAN_POINT('Ctrl Pts',(67.8511540812208,8.75235638610652,57.2724376206627));
#169627=CARTESIAN_POINT('Ctrl Pts',(67.6600578693407,8.64196238927888,57.3080782900684));
#169628=CARTESIAN_POINT('Ctrl Pts',(67.2175591210862,8.36599611620118,57.3905295534725));
#169629=CARTESIAN_POINT('Ctrl Pts',(66.9696341734787,8.19507159405754,57.4366609657191));
#169630=CARTESIAN_POINT('Ctrl Pts',(66.4438464427843,7.79574362683847,57.5347582742036));
#169631=CARTESIAN_POINT('Ctrl Pts',(66.1697767596987,7.56290386938635,57.5860676631683));
#169632=CARTESIAN_POINT('Ctrl Pts',(65.8583775761023,7.26753532360987,57.6451042854397));
#169633=CARTESIAN_POINT('Ctrl Pts',(65.8083895065521,7.21910494183,57.6546059483399));
#169634=CARTESIAN_POINT('Ctrl Pts',(65.7370365720214,7.14849520084388,57.6682097371229));
#169635=CARTESIAN_POINT('Ctrl Pts',(65.7152613999905,7.12674411985674,57.6723669140076));
#169636=CARTESIAN_POINT('Ctrl Pts',(65.6770611289512,7.08822709864953,57.6796703990337));
#169637=CARTESIAN_POINT('Ctrl Pts',(65.6605939355939,7.07150438459761,57.6828222612992));
#169638=CARTESIAN_POINT('Ctrl Pts',(65.6252167011947,7.03532073221709,57.6896013079857));
#169639=CARTESIAN_POINT('Ctrl Pts',(65.6063268311122,7.01584010477385,57.6932257874504));
#169640=CARTESIAN_POINT('Ctrl Pts',(65.5533240088667,6.96072658762479,57.7034085892717));
#169641=CARTESIAN_POINT('Ctrl Pts',(65.5193952313301,6.92491311339782,57.7099421413555));
#169642=CARTESIAN_POINT('Ctrl Pts',(65.283066071036,6.67168263224396,57.7555505508232));
#169643=CARTESIAN_POINT('Ctrl Pts',(65.0901732058478,6.44535836798946,57.7932889557165));
#169644=CARTESIAN_POINT('Ctrl Pts',(64.7885022084069,6.05739191205442,57.8528130777467));
#169645=CARTESIAN_POINT('Ctrl Pts',(64.6738607905233,5.90070242968286,57.8755715312986));
#169646=CARTESIAN_POINT('Ctrl Pts',(64.287253920152,5.33856541730202,57.9526423385588));
#169647=CARTESIAN_POINT('Ctrl Pts',(64.040221105445,4.91621195611723,58.0024542000079));
#169648=CARTESIAN_POINT('Ctrl Pts',(63.7775918557604,4.38120704456539,58.0556145728963));
#169649=CARTESIAN_POINT('Ctrl Pts',(63.7320559606948,4.28459179474932,58.064842932154));
#169650=CARTESIAN_POINT('Ctrl Pts',(63.6664199724308,4.13939055152813,58.078159961223));
#169651=CARTESIAN_POINT('Ctrl Pts',(63.6451582906387,4.09135915692004,58.0824763521399));
#169652=CARTESIAN_POINT('Ctrl Pts',(63.6076744457373,4.00486260710316,58.0900906373594));
#169653=CARTESIAN_POINT('Ctrl Pts',(63.5913148872551,3.96646073489049,58.0934154829661));
#169654=CARTESIAN_POINT('Ctrl Pts',(63.5569524441323,3.88439179869214,58.1004027326542));
#169655=CARTESIAN_POINT('Ctrl Pts',(63.5390163989046,3.84069674659609,58.1040520213532));
#169656=CARTESIAN_POINT('Ctrl Pts',(63.4912016664778,3.72184654249729,58.1137866322386));
#169657=CARTESIAN_POINT('Ctrl Pts',(63.461914474154,3.64644787228342,58.1197559777224));
#169658=CARTESIAN_POINT('Ctrl Pts',(63.2993237374074,3.21250580671838,58.1529389311906));
#169659=CARTESIAN_POINT('Ctrl Pts',(63.185448854058,2.8467383454678,58.176338518366));
#169660=CARTESIAN_POINT('Ctrl Pts',(62.9646140568515,1.96398543113634,58.2226196055605));
#169661=CARTESIAN_POINT('Ctrl Pts',(62.8766945410915,1.44324608427282,58.2419059869019));
#169662=CARTESIAN_POINT('Ctrl Pts',(62.8096001378845,0.692362390434222,
58.2599719580861));
#169663=CARTESIAN_POINT('Ctrl Pts',(62.7970198741906,0.46623249628501,58.2641754945589));
#169664=CARTESIAN_POINT('Ctrl Pts',(62.7910382678108,0.193820077886311,
58.2678904327133));
#169665=CARTESIAN_POINT('Ctrl Pts',(62.7903421927524,0.147778305705106,
58.2684720525722));
#169666=CARTESIAN_POINT('Ctrl Pts',(62.7897489103399,0.0760961461433343,
58.2693071413881));
#169667=CARTESIAN_POINT('Ctrl Pts',(62.7896343689182,0.0504585672256714,
58.2695917929293));
#169668=CARTESIAN_POINT('Ctrl Pts',(62.7896120602203,0.0165471062013723,
58.2699499944522));
#169669=CARTESIAN_POINT('Ctrl Pts',(62.789616789492,0.00827354424855654,
58.2700359449107));
#169670=CARTESIAN_POINT('Ctrl Pts',(62.7896316916575,-5.79826049313321E-11,
58.2701204592907));
#169671=CARTESIAN_POINT('Origin',(72.2537026314029,-4.33680868994202E-16,
54.3558290880045));
#169672=CARTESIAN_POINT('',(62.9072242170052,2.7021311761062E-11,58.9370208104186));
#169673=CARTESIAN_POINT('',(62.9025030071409,2.44438148519277E-14,58.910245498748));
#169674=CARTESIAN_POINT('',(62.4056251012807,-1.65832766814156E-15,56.0923108646735));
#169675=CARTESIAN_POINT('Ctrl Pts',(62.9072242170052,5.40442818497922E-11,
58.9370208104186));
#169676=CARTESIAN_POINT('Ctrl Pts',(62.9072099714203,0.00790901692578116,
58.9369400196918));
#169677=CARTESIAN_POINT('Ctrl Pts',(62.9072049102169,0.0158180443091237,
58.9368572823768));
#169678=CARTESIAN_POINT('Ctrl Pts',(62.9072223236603,0.0492122228663902,
58.9364997435817));
#169679=CARTESIAN_POINT('Ctrl Pts',(62.9073309856082,0.0746970095420169,
58.9362067275076));
#169680=CARTESIAN_POINT('Ctrl Pts',(62.9078983196514,0.145548068002589,
58.9353365036641));
#169681=CARTESIAN_POINT('Ctrl Pts',(62.9085639252973,0.19091154185888,58.9347159484371));
#169682=CARTESIAN_POINT('Ctrl Pts',(62.914083478072,0.449523595448512,58.930821944839));
#169683=CARTESIAN_POINT('Ctrl Pts',(62.9253196393055,0.662561934454989,
58.9262334789076));
#169684=CARTESIAN_POINT('Ctrl Pts',(62.9979891074459,1.52433953176591,58.9024195406952));
#169685=CARTESIAN_POINT('Ctrl Pts',(63.1149747013286,2.16649684139304,58.8726607003243));
#169686=CARTESIAN_POINT('Ctrl Pts',(63.3443570660399,2.97374699778817,58.821663746837));
#169687=CARTESIAN_POINT('Ctrl Pts',(63.4009550725885,3.1535826411818,58.8093857239716));
#169688=CARTESIAN_POINT('Ctrl Pts',(63.5064351023077,3.45855579379913,58.7870053930245));
#169689=CARTESIAN_POINT('Ctrl Pts',(63.5528456303677,3.58452159447197,58.7772946324959));
#169690=CARTESIAN_POINT('Ctrl Pts',(63.6227038128266,3.76302421421529,58.7628645056372));
#169691=CARTESIAN_POINT('Ctrl Pts',(63.6441105610017,3.81636952546874,58.758465381957));
#169692=CARTESIAN_POINT('Ctrl Pts',(63.6821033324133,3.90874492530129,58.7506963692028));
#169693=CARTESIAN_POINT('Ctrl Pts',(63.6984818927013,3.94786141543798,58.747359002905));
#169694=CARTESIAN_POINT('Ctrl Pts',(63.7305864134983,4.02319256790192,58.7408396397097));
#169695=CARTESIAN_POINT('Ctrl Pts',(63.7462793550074,4.05942088576101,58.7376628283205));
#169696=CARTESIAN_POINT('Ctrl Pts',(63.7884448525589,4.15520941778614,58.7291527424406));
#169697=CARTESIAN_POINT('Ctrl Pts',(63.8152827515735,4.21460159034845,58.7237622603097));
#169698=CARTESIAN_POINT('Ctrl Pts',(63.9157462712276,4.43127501901037,58.7036757439514));
#169699=CARTESIAN_POINT('Ctrl Pts',(63.9928553458238,4.58685535633015,58.6884337066871));
#169700=CARTESIAN_POINT('Ctrl Pts',(64.3299796384894,5.2248400448046,58.6224229689439));
#169701=CARTESIAN_POINT('Ctrl Pts',(64.6250941257276,5.68701860783708,58.5661299263498));
#169702=CARTESIAN_POINT('Ctrl Pts',(65.1409671780277,6.36513302978434,58.4681738755596));
#169703=CARTESIAN_POINT('Ctrl Pts',(65.3367536087514,6.59933673394019,58.4310616145545));
#169704=CARTESIAN_POINT('Ctrl Pts',(65.5886306731084,6.87397495057979,58.3830608139658));
#169705=CARTESIAN_POINT('Ctrl Pts',(65.6349741409503,6.92348032315649,58.3742189546327));
#169706=CARTESIAN_POINT('Ctrl Pts',(65.7030811716782,6.99475923142845,58.3612055093332));
#169707=CARTESIAN_POINT('Ctrl Pts',(65.7244532444699,7.01691964646535,58.3571191606363));
#169708=CARTESIAN_POINT('Ctrl Pts',(65.7621127677075,7.05560708156892,58.3499133524138));
#169709=CARTESIAN_POINT('Ctrl Pts',(65.7783566498744,7.07217784936632,58.3468035043139));
#169710=CARTESIAN_POINT('Ctrl Pts',(65.8138969522583,7.10818028216566,58.3399955198663));
#169711=CARTESIAN_POINT('Ctrl Pts',(65.833215376259,7.12758875897559,58.3362925247325));
#169712=CARTESIAN_POINT('Ctrl Pts',(65.8874094294959,7.18158694534945,58.3258983437606));
#169713=CARTESIAN_POINT('Ctrl Pts',(65.9224581545836,7.21599447354607,58.3191690945198));
#169714=CARTESIAN_POINT('Ctrl Pts',(66.1460933339935,7.43230066183781,58.2761949037771));
#169715=CARTESIAN_POINT('Ctrl Pts',(66.3414265066577,7.60678559789629,58.2384969884545));
#169716=CARTESIAN_POINT('Ctrl Pts',(66.96643879466,8.12189261756985,58.1178935357555));
#169717=CARTESIAN_POINT('Ctrl Pts',(67.4173223138905,8.43418822257564,58.0309712340087));
#169718=CARTESIAN_POINT('Ctrl Pts',(68.0868740326202,8.81918656896863,57.903365161378));
#169719=CARTESIAN_POINT('Ctrl Pts',(68.2860330616276,8.92469844476276,57.8655674196164));
#169720=CARTESIAN_POINT('Ctrl Pts',(68.5523425875103,9.05416498403435,57.815263723373));
#169721=CARTESIAN_POINT('Ctrl Pts',(68.6164147943805,9.08445319839993,57.8031784602715));
#169722=CARTESIAN_POINT('Ctrl Pts',(68.7214455199851,9.13270684668133,57.7833963626669));
#169723=CARTESIAN_POINT('Ctrl Pts',(68.7622111693946,9.15109621926484,57.7757253014748));
#169724=CARTESIAN_POINT('Ctrl Pts',(68.8412908242867,9.18611473125428,57.7608579913955));
#169725=CARTESIAN_POINT('Ctrl Pts',(68.8795883491662,9.20277960523408,57.7536639543031));
#169726=CARTESIAN_POINT('Ctrl Pts',(68.9693383521251,9.24114781486347,57.7368188421719));
#169727=CARTESIAN_POINT('Ctrl Pts',(69.020871161784,9.26265489952566,57.7271574233656));
#169728=CARTESIAN_POINT('Ctrl Pts',(69.1901106536621,9.33158027280642,57.6954627846869));
#169729=CARTESIAN_POINT('Ctrl Pts',(69.3085460544608,9.37713114827548,57.6733370777983));
#169730=CARTESIAN_POINT('Ctrl Pts',(69.8579557704563,9.57617069789906,57.5709306182368));
#169731=CARTESIAN_POINT('Ctrl Pts',(70.2983559506258,9.70132920320212,57.4895274646193));
#169732=CARTESIAN_POINT('Ctrl Pts',(71.2942694631327,9.90964150232231,57.305932341899));
#169733=CARTESIAN_POINT('Ctrl Pts',(71.8514694646905,9.9765227365849,57.2035482040618));
#169734=CARTESIAN_POINT('Ctrl Pts',(72.4728185408518,9.99685256945185,57.0879616226865));
#169735=CARTESIAN_POINT('Ctrl Pts',(72.5346505210121,9.99828181634118,57.0764431279122));
#169736=CARTESIAN_POINT('Ctrl Pts',(72.6248549170636,9.99950089481505,57.0596117595833));
#169737=CARTESIAN_POINT('Ctrl Pts',(72.6532223781713,9.9997593561708,57.0543146720848));
#169738=CARTESIAN_POINT('Ctrl Pts',(72.7031287002219,9.99999431123556,57.044988182496));
#169739=CARTESIAN_POINT('Ctrl Pts',(72.7246674202334,10.0000237023634,57.0409605807427));
#169740=CARTESIAN_POINT('Ctrl Pts',(72.770701546333,9.99993260503462,57.0323471199713));
#169741=CARTESIAN_POINT('Ctrl Pts',(72.7951964722171,9.99979098279492,57.0277606547346));
#169742=CARTESIAN_POINT('Ctrl Pts',(72.862952647179,9.99914155429355,57.0150654391661));
#169743=CARTESIAN_POINT('Ctrl Pts',(72.9062103478262,9.99843631372799,57.006950877971));
#169744=CARTESIAN_POINT('Ctrl Pts',(73.1581763788988,9.99263517906828,56.9596348577346));
#169745=CARTESIAN_POINT('Ctrl Pts',(73.3666532149147,9.98106536972207,56.9202842055288));
#169746=CARTESIAN_POINT('Ctrl Pts',(73.9664364500754,9.92823246739088,56.8067478861944));
#169747=CARTESIAN_POINT('Ctrl Pts',(74.3558284558308,9.86980459667376,56.7326488791205));
#169748=CARTESIAN_POINT('Ctrl Pts',(75.2413158291936,9.68110915818093,56.5642973908312));
#169749=CARTESIAN_POINT('Ctrl Pts',(75.7329741129178,9.53481733868083,56.4709626815177));
#169750=CARTESIAN_POINT('Ctrl Pts',(76.289398075909,9.32010056864745,56.3660078907599));
#169751=CARTESIAN_POINT('Ctrl Pts',(76.3671075955933,9.28895588853841,56.351364415483));
#169752=CARTESIAN_POINT('Ctrl Pts',(76.4887300842574,9.23838171984617,56.3284689807045));
#169753=CARTESIAN_POINT('Ctrl Pts',(76.5329079298455,9.21962723535497,56.3201573060205));
#169754=CARTESIAN_POINT('Ctrl Pts',(76.6143364945807,9.18434679062292,56.3048460498126));
#169755=CARTESIAN_POINT('Ctrl Pts',(76.6516242935245,9.1679127289542,56.2978381588468));
#169756=CARTESIAN_POINT('Ctrl Pts',(76.7344099097664,9.13080467554706,56.2822869316835));
#169757=CARTESIAN_POINT('Ctrl Pts',(76.7798558479759,9.11001298678257,56.2737550551609));
#169758=CARTESIAN_POINT('Ctrl Pts',(76.9118334746308,9.04840208803876,56.2489924428116));
#169759=CARTESIAN_POINT('Ctrl Pts',(76.9979413263648,9.00665194493683,56.2328545356675));
#169760=CARTESIAN_POINT('Ctrl Pts',(77.3841244304719,8.81234711301676,56.160552686014));
#169761=CARTESIAN_POINT('Ctrl Pts',(77.6770352127363,8.64550191482432,56.105929013356));
#169762=CARTESIAN_POINT('Ctrl Pts',(78.408644020972,8.17723440513523,55.9696435213792));
#169763=CARTESIAN_POINT('Ctrl Pts',(78.8328513716642,7.85444784033037,55.8907981797405));
#169764=CARTESIAN_POINT('Ctrl Pts',(79.3308440876463,7.4073590267506,55.7969444636213));
#169765=CARTESIAN_POINT('Ctrl Pts',(79.4305232913329,7.31405828729849,55.7780829839275));
#169766=CARTESIAN_POINT('Ctrl Pts',(79.5579481356863,7.18972030950491,55.7538366893383));
#169767=CARTESIAN_POINT('Ctrl Pts',(79.5874578565791,7.16055965952134,55.7482118641509));
#169768=CARTESIAN_POINT('Ctrl Pts',(79.6347572932563,7.11322593737397,55.7391791053005));
#169769=CARTESIAN_POINT('Ctrl Pts',(79.6526608714437,7.09517025378022,55.7357560694201));
#169770=CARTESIAN_POINT('Ctrl Pts',(79.6873827345013,7.05988143305583,55.7291093395206));
#169771=CARTESIAN_POINT('Ctrl Pts',(79.70420798506,7.04265570807208,55.7258847200167));
#169772=CARTESIAN_POINT('Ctrl Pts',(79.7454357550802,7.00013629364943,55.7179742160835));
#169773=CARTESIAN_POINT('Ctrl Pts',(79.769767428884,6.97477254054825,55.7132977570772));
#169774=CARTESIAN_POINT('Ctrl Pts',(79.8594096120248,6.88032337847043,55.6960411856496));
#169775=CARTESIAN_POINT('Ctrl Pts',(79.9238673893492,6.81041443214672,55.6835778309452));
#169776=CARTESIAN_POINT('Ctrl Pts',(80.0875772821118,6.62763857621036,55.6518011115764));
#169777=CARTESIAN_POINT('Ctrl Pts',(80.1853035867766,6.51339870097038,55.6327120356469));
#169778=CARTESIAN_POINT('Ctrl Pts',(80.4987040893437,6.12971420976461,55.5711894503913));
#169779=CARTESIAN_POINT('Ctrl Pts',(80.7030701859377,5.85107048554801,55.5305775026007));
#169780=CARTESIAN_POINT('Ctrl Pts',(81.1432751320225,5.18051551057712,55.4425525424328));
#169781=CARTESIAN_POINT('Ctrl Pts',(81.3676554092802,4.78174074339207,55.3972589895638));
#169782=CARTESIAN_POINT('Ctrl Pts',(81.5995376466848,4.2947398871361,55.3502808347035));
#169783=CARTESIAN_POINT('Ctrl Pts',(81.6338333089187,4.22039165055155,55.3433263560345));
#169784=CARTESIAN_POINT('Ctrl Pts',(81.6867568252709,4.10188772790358,55.332584928723));
#169785=CARTESIAN_POINT('Ctrl Pts',(81.7059781403745,4.05801179258908,55.3286816107324));
#169786=CARTESIAN_POINT('Ctrl Pts',(81.741332680708,3.97572000802668,55.3214980692558));
#169787=CARTESIAN_POINT('Ctrl Pts',(81.7575414059008,3.93733903303375,55.3182030361024));
#169788=CARTESIAN_POINT('Ctrl Pts',(81.7932735625761,3.851245334889,55.3109353486928));
#169789=CARTESIAN_POINT('Ctrl Pts',(81.8126709235696,3.80347950775275,55.3069874280684));
#169790=CARTESIAN_POINT('Ctrl Pts',(81.8692303245645,3.6610858909923,55.2954677385405));
#169791=CARTESIAN_POINT('Ctrl Pts',(81.9053367658428,3.56602944462098,55.2881028875509));
#169792=CARTESIAN_POINT('Ctrl Pts',(82.065473195865,3.12449460093883,55.255379535993));
#169793=CARTESIAN_POINT('Ctrl Pts',(82.1720534376146,2.77174544102934,55.2334384729471));
#169794=CARTESIAN_POINT('Ctrl Pts',(82.3758136352477,1.93510532764585,55.1906143018418));
#169795=CARTESIAN_POINT('Ctrl Pts',(82.457417863787,1.44827160084945,55.172657325847));
#169796=CARTESIAN_POINT('Ctrl Pts',(82.5253683923865,0.719948308188185,
55.1546675041677));
#169797=CARTESIAN_POINT('Ctrl Pts',(82.5391241014064,0.481884319809271,
55.1501660288107));
#169798=CARTESIAN_POINT('Ctrl Pts',(82.5454879615095,0.196801508651396,
55.1462630147488));
#169799=CARTESIAN_POINT('Ctrl Pts',(82.546206839377,0.150056984184883,55.1456707560209));
#169800=CARTESIAN_POINT('Ctrl Pts',(82.546818565591,0.0775143892891936,
55.1448240170581));
#169801=CARTESIAN_POINT('Ctrl Pts',(82.5469372335081,0.0517192751872206,
55.1445371285694));
#169802=CARTESIAN_POINT('Ctrl Pts',(82.5469737250037,0.00415092054648192,
55.1440339344148));
#169803=CARTESIAN_POINT('Ctrl Pts',(82.5469199774665,-0.0176219032436765,
55.1438135712789));
#169804=CARTESIAN_POINT('Ctrl Pts',(82.5466360218009,-0.0674037138328463,
55.1433325596077));
#169805=CARTESIAN_POINT('Ctrl Pts',(82.5463596861604,-0.0954122076489487,
55.1430784888024));
#169806=CARTESIAN_POINT('Ctrl Pts',(82.5451378539625,-0.182516811522682,
55.1423405096052));
#169807=CARTESIAN_POINT('Ctrl Pts',(82.5437900812275,-0.241606505921511,
55.1419145693536));
#169808=CARTESIAN_POINT('Ctrl Pts',(82.5282466003325,-0.733675716738335,
55.1390061573088));
#169809=CARTESIAN_POINT('Ctrl Pts',(82.486744801119,-1.16536485403954,55.140592691685));
#169810=CARTESIAN_POINT('Ctrl Pts',(82.3161439861218,-2.22354496998105,
55.1563809273633));
#169811=CARTESIAN_POINT('Ctrl Pts',(82.1552312645009,-2.84289423828583,
55.1762521081694));
#169812=CARTESIAN_POINT('Ctrl Pts',(81.9005478441486,-3.54413120966995,
55.2125774474713));
#169813=CARTESIAN_POINT('Ctrl Pts',(81.8620454506646,-3.64508381083524,
55.2181538028504));
#169814=CARTESIAN_POINT('Ctrl Pts',(81.8023248028915,-3.79445333689554,
55.2269250276648));
#169815=CARTESIAN_POINT('Ctrl Pts',(81.7823247749792,-3.84336265789555,
55.2298812216485));
#169816=CARTESIAN_POINT('Ctrl Pts',(81.7458112214872,-3.93069828419579,
55.2353111728736));
#169817=CARTESIAN_POINT('Ctrl Pts',(81.7294399786342,-3.96918443671297,
55.2377570416467));
#169818=CARTESIAN_POINT('Ctrl Pts',(81.6941074474136,-4.05083720985216,
55.2430592826185));
#169819=CARTESIAN_POINT('Ctrl Pts',(81.6750823900781,-4.09397430902961,
55.2459281832408));
#169820=CARTESIAN_POINT('Ctrl Pts',(81.6228218298127,-4.21026123399974,
55.2538454315186));
#169821=CARTESIAN_POINT('Ctrl Pts',(81.5890181752935,-4.28314420858446,
55.2590052344547));
#169822=CARTESIAN_POINT('Ctrl Pts',(81.3863203953756,-4.70686969538077,
55.2901599628658));
#169823=CARTESIAN_POINT('Ctrl Pts',(81.1982511699067,-5.04788308417159,
55.3199254042824));
#169824=CARTESIAN_POINT('Ctrl Pts',(80.7954080428616,-5.68761772188648,
55.3847075617269));
#169825=CARTESIAN_POINT('Ctrl Pts',(80.5830110594757,-5.98714289113689,
55.4192868711626));
#169826=CARTESIAN_POINT('Ctrl Pts',(80.2202137598613,-6.44331288287155,
55.478389073045));
#169827=CARTESIAN_POINT('Ctrl Pts',(80.0802347356817,-6.60803030250808,
55.5011971696345));
#169828=CARTESIAN_POINT('Ctrl Pts',(79.8784750202396,-6.83033916260853,
55.5339436495727));
#169829=CARTESIAN_POINT('Ctrl Pts',(79.8211125931903,-6.89195185312143,
55.543240172835));
#169830=CARTESIAN_POINT('Ctrl Pts',(79.7391358283428,-6.97778655058047,
55.5564980926484));
#169831=CARTESIAN_POINT('Ctrl Pts',(79.7151615050614,-7.00262820513807,
55.5603721350819));
#169832=CARTESIAN_POINT('Ctrl Pts',(79.6744629507664,-7.04436076701493,
55.5669424288867));
#169833=CARTESIAN_POINT('Ctrl Pts',(79.6578060748199,-7.06131839815295,
55.56962973432));
#169834=CARTESIAN_POINT('Ctrl Pts',(79.6230409417495,-7.09645750039703,
55.5752346088084));
#169835=CARTESIAN_POINT('Ctrl Pts',(79.604922928228,-7.11462871140889,55.5781534762829));
#169836=CARTESIAN_POINT('Ctrl Pts',(79.5567096977773,-7.16260941086454,
55.5859155760166));
#169837=CARTESIAN_POINT('Ctrl Pts',(79.5264948622572,-7.19229538279288,
55.590774695932));
#169838=CARTESIAN_POINT('Ctrl Pts',(79.3803538031251,-7.3340489100916,55.6142551348318));
#169839=CARTESIAN_POINT('Ctrl Pts',(79.2619225699825,-7.44344246608252,
55.6332183622152));
#169840=CARTESIAN_POINT('Ctrl Pts',(78.8816511477967,-7.77787932078961,
55.6940305091882));
#169841=CARTESIAN_POINT('Ctrl Pts',(78.6108053589414,-7.99204271404234,
55.7372408746047));
#169842=CARTESIAN_POINT('Ctrl Pts',(78.3039481208405,-8.20962589212828,
55.7864299336672));
#169843=CARTESIAN_POINT('Ctrl Pts',(78.2782804915427,-8.22764307286505,
55.7905460701455));
#169844=CARTESIAN_POINT('Ctrl Pts',(77.880172692812,-8.50427274301525,55.8544158078225));
#169845=CARTESIAN_POINT('Ctrl Pts',(77.4907942677911,-8.73684180465576,
55.9172955087661));
#169846=CARTESIAN_POINT('Ctrl Pts',(76.9925077600569,-8.98964335241288,
55.9986907256555));
#169847=CARTESIAN_POINT('Ctrl Pts',(76.8970699652099,-9.03613519547111,
56.014318683139));
#169848=CARTESIAN_POINT('Ctrl Pts',(76.753673447537,-9.10313756497479,56.0378584112176));
#169849=CARTESIAN_POINT('Ctrl Pts',(76.7062581816379,-9.12483413679376,
56.0456514046435));
#169850=CARTESIAN_POINT('Ctrl Pts',(76.6208858085757,-9.16307994958528,
56.0596997494516));
#169851=CARTESIAN_POINT('Ctrl Pts',(76.5829906678094,-9.17976942835726,
56.0659414448347));
#169852=CARTESIAN_POINT('Ctrl Pts',(76.5020194818393,-9.21481997950538,
56.0792907157792));
#169853=CARTESIAN_POINT('Ctrl Pts',(76.4589161739331,-9.23311312783332,
56.0864044248266));
#169854=CARTESIAN_POINT('Ctrl Pts',(76.3417111113945,-9.28186781259756,
56.1057679107776));
#169855=CARTESIAN_POINT('Ctrl Pts',(76.2673719603771,-9.31172780239573,
56.1180712060214));
#169856=CARTESIAN_POINT('Ctrl Pts',(75.8403759152482,-9.47718978747199,
56.1888598731825));
#169857=CARTESIAN_POINT('Ctrl Pts',(75.4807137943323,-9.59312044409277,
56.2489661600192));
#169858=CARTESIAN_POINT('Ctrl Pts',(74.5865826797033,-9.8250983877885,56.3990809817534));
#169859=CARTESIAN_POINT('Ctrl Pts',(74.047523912526,-9.91754541389785,56.4901918750426));
#169860=CARTESIAN_POINT('Ctrl Pts',(73.3031321300179,-9.98150847637653,
56.6150972981622));
#169861=CARTESIAN_POINT('Ctrl Pts',(73.102186028597,-9.99251000826106,56.6487182522762));
#169862=CARTESIAN_POINT('Ctrl Pts',(72.8567856408011,-9.99832056019788,
56.6895550734642));
#169863=CARTESIAN_POINT('Ctrl Pts',(72.8125438096882,-9.99906623277688,
56.6969084890224));
#169864=CARTESIAN_POINT('Ctrl Pts',(72.743271029061,-9.99976125388288,56.7084069744269));
#169865=CARTESIAN_POINT('Ctrl Pts',(72.7182437511166,-9.99991581248507,
56.7125580859481));
#169866=CARTESIAN_POINT('Ctrl Pts',(72.6718867547311,-10.0000232896589,
56.720240897245));
#169867=CARTESIAN_POINT('Ctrl Pts',(72.6505575666984,-10.0000026347173,
56.7237733825021));
#169868=CARTESIAN_POINT('Ctrl Pts',(72.6011101604298,-9.99979223162048,
56.7319571946038));
#169869=CARTESIAN_POINT('Ctrl Pts',(72.5729921321942,-9.99955075840802,
56.7366067565296));
#169870=CARTESIAN_POINT('Ctrl Pts',(72.4839986005901,-9.9984009009029,56.7513102993948));
#169871=CARTESIAN_POINT('Ctrl Pts',(72.4231278486966,-9.99704331373609,
56.7613491502423));
#169872=CARTESIAN_POINT('Ctrl Pts',(72.1056434015103,-9.98698291980609,
56.8136258094129));
#169873=CARTESIAN_POINT('Ctrl Pts',(71.8493801283175,-9.96870393054267,
56.8555406635842));
#169874=CARTESIAN_POINT('Ctrl Pts',(71.0099468825211,-9.87537234423317,
56.9924295681601));
#169875=CARTESIAN_POINT('Ctrl Pts',(70.4325720674018,-9.7576990451472,57.0860028999719));
#169876=CARTESIAN_POINT('Ctrl Pts',(69.6163526445126,-9.51290734268113,
57.2191566602303));
#169877=CARTESIAN_POINT('Ctrl Pts',(69.3667475312224,-9.42688894167878,
57.2599856399268));
#169878=CARTESIAN_POINT('Ctrl Pts',(69.0506988897274,-9.30344679008716,
57.311868061212));
#169879=CARTESIAN_POINT('Ctrl Pts',(68.9808489382277,-9.27523072093014,
57.3233461932567));
#169880=CARTESIAN_POINT('Ctrl Pts',(68.8690716619505,-9.22856941639705,
57.3417328252203));
#169881=CARTESIAN_POINT('Ctrl Pts',(68.8269395603865,-9.21063318741089,
57.3486676069018));
#169882=CARTESIAN_POINT('Ctrl Pts',(68.7467644712484,-9.17583496517369,
57.3618722991207));
#169883=CARTESIAN_POINT('Ctrl Pts',(68.7087004656476,-9.15902494469959,
57.3681449208736));
#169884=CARTESIAN_POINT('Ctrl Pts',(68.6215222449076,-9.11985887408198,
57.3825191540077));
#169885=CARTESIAN_POINT('Ctrl Pts',(68.5724820082497,-9.09733789313285,
57.3906109538339));
#169886=CARTESIAN_POINT('Ctrl Pts',(68.418729997444,-9.02518523672881,57.4159983973812));
#169887=CARTESIAN_POINT('Ctrl Pts',(68.3146989662436,-8.97409471314912,
57.4332023172028));
#169888=CARTESIAN_POINT('Ctrl Pts',(68.0716026032028,-8.84931051705981,
57.4734580635512));
#169889=CARTESIAN_POINT('Ctrl Pts',(67.9333420559465,-8.77408341770417,
57.4963963839914));
#169890=CARTESIAN_POINT('Ctrl Pts',(67.3908779586117,-8.4618010403139,57.5865107307297));
#169891=CARTESIAN_POINT('Ctrl Pts',(67.0017752889355,-8.19912903618128,
57.6514419458594));
#169892=CARTESIAN_POINT('Ctrl Pts',(66.4873295702514,-7.7957371799568,57.7367781668038));
#169893=CARTESIAN_POINT('Ctrl Pts',(66.3453773571203,-7.67787966963978,
57.7602608272079));
#169894=CARTESIAN_POINT('Ctrl Pts',(66.0855607086834,-7.44963538898656,
57.8030108968417));
#169895=CARTESIAN_POINT('Ctrl Pts',(65.9669543169776,-7.34021392474407,
57.8224299541468));
#169896=CARTESIAN_POINT('Ctrl Pts',(65.8194810921125,-7.19737679803652,
57.8463957810109));
#169897=CARTESIAN_POINT('Ctrl Pts',(65.7881517100808,-7.1666288793118,57.8514764132685));
#169898=CARTESIAN_POINT('Ctrl Pts',(65.7385891572439,-7.11734004022096,
57.8594953144461));
#169899=CARTESIAN_POINT('Ctrl Pts',(65.7202261268116,-7.09893519843986,
57.862462217087));
#169900=CARTESIAN_POINT('Ctrl Pts',(65.6851318310884,-7.06348522795356,
57.8681240855368));
#169901=CARTESIAN_POINT('Ctrl Pts',(65.668389702301,-7.04645168386884,57.8708214471548));
#169902=CARTESIAN_POINT('Ctrl Pts',(65.6280839667193,-7.00514915834031,
57.8773065011249));
#169903=CARTESIAN_POINT('Ctrl Pts',(65.6045811208325,-6.98081914027601,
57.8810808029697));
#169904=CARTESIAN_POINT('Ctrl Pts',(65.521961844959,-6.8944183850771,57.8943242595585));
#169905=CARTESIAN_POINT('Ctrl Pts',(65.463509824559,-6.83169549597652,57.9036494685014));
#169906=CARTESIAN_POINT('Ctrl Pts',(65.0759533240894,-6.40494408738154,
57.9652173088012));
#169907=CARTESIAN_POINT('Ctrl Pts',(64.7728440328764,-6.01744829571551,
58.0121126516977));
#169908=CARTESIAN_POINT('Ctrl Pts',(64.2340391880073,-5.21310548434183,
58.0945659873071));
#169909=CARTESIAN_POINT('Ctrl Pts',(63.9972270022942,-4.79858339243606,
58.1303310412948));
#169910=CARTESIAN_POINT('Ctrl Pts',(63.7551287009896,-4.29463608264552,
58.1667166652259));
#169911=CARTESIAN_POINT('Ctrl Pts',(63.7205342260945,-4.22031053671581,
58.1719096723079));
#169912=CARTESIAN_POINT('Ctrl Pts',(63.6671421450482,-4.10183465636789,
58.1799149056046));
#169913=CARTESIAN_POINT('Ctrl Pts',(63.6477475544268,-4.0579638398674,58.1828206796472));
#169914=CARTESIAN_POINT('Ctrl Pts',(63.6120706817561,-3.97567664707459,
58.1881619551793));
#169915=CARTESIAN_POINT('Ctrl Pts',(63.5957124681839,-3.93729510868763,
58.190609350044));
#169916=CARTESIAN_POINT('Ctrl Pts',(63.5596467454594,-3.85119360855982,
58.196001488352));
#169917=CARTESIAN_POINT('Ctrl Pts',(63.540066267015,-3.80342049946292,58.1989263388992));
#169918=CARTESIAN_POINT('Ctrl Pts',(63.4829614504212,-3.66098305369202,
58.20744826568));
#169919=CARTESIAN_POINT('Ctrl Pts',(63.4465008112283,-3.56588967069123,
58.2128785897505));
#169920=CARTESIAN_POINT('Ctrl Pts',(63.284725431708,-3.12404434226735,58.2369140044108));
#169921=CARTESIAN_POINT('Ctrl Pts',(63.1770057764588,-2.7710119260063,58.2527577501688));
#169922=CARTESIAN_POINT('Ctrl Pts',(62.9715179067535,-1.93655821366227,
58.2821140804204));
#169923=CARTESIAN_POINT('Ctrl Pts',(62.8889917412337,-1.45228515243556,
58.2931139426145));
#169924=CARTESIAN_POINT('Ctrl Pts',(62.8185609419714,-0.724513613636625,
58.2995354572268));
#169925=CARTESIAN_POINT('Ctrl Pts',(62.8038869612924,-0.484400027867834,
58.3000313765559));
#169926=CARTESIAN_POINT('Ctrl Pts',(62.796504011387,-0.197173501351806,
58.2985317688595));
#169927=CARTESIAN_POINT('Ctrl Pts',(62.7956227610553,-0.150340766037461,
58.2982208256383));
#169928=CARTESIAN_POINT('Ctrl Pts',(62.7947556468869,-0.077690223885297,
58.2976337926366));
#169929=CARTESIAN_POINT('Ctrl Pts',(62.7945454341098,-0.0518753922316298,
58.2974047057229));
#169930=CARTESIAN_POINT('Ctrl Pts',(62.7943952737771,-0.0173734758123369,
58.297070893174));
#169931=CARTESIAN_POINT('Ctrl Pts',(62.7943685479087,-0.00868672916154148,
58.2969845060308));
#169932=CARTESIAN_POINT('Ctrl Pts',(62.7943529015217,6.10048743283802E-11,
58.2968957709606));
#169933=CARTESIAN_POINT('Ctrl Pts',(62.7896316916575,-5.79826049313321E-11,
58.2701204592907));
#169934=CARTESIAN_POINT('Ctrl Pts',(62.7896560368138,-0.0135162054405685,
58.2702585275327));
#169935=CARTESIAN_POINT('Ctrl Pts',(62.7897075319756,-0.0270323637277315,
58.2703927630781));
#169936=CARTESIAN_POINT('Ctrl Pts',(62.7899503939444,-0.068773338415487,
58.2707954032247));
#169937=CARTESIAN_POINT('Ctrl Pts',(62.7902329888609,-0.0969975643424201,
58.2710508411162));
#169938=CARTESIAN_POINT('Ctrl Pts',(62.7914895794682,-0.185455098057772,
58.2717980112957));
#169939=CARTESIAN_POINT('Ctrl Pts',(62.7928842060982,-0.245681608635885,
58.27222911253));
#169940=CARTESIAN_POINT('Ctrl Pts',(62.8027670692509,-0.553516669642862,
58.2740250870666));
#169941=CARTESIAN_POINT('Ctrl Pts',(62.8198196832118,-0.800772308294341,
58.27411742739));
#169942=CARTESIAN_POINT('Ctrl Pts',(62.9161211585352,-1.7099521352087,58.2689787452707));
#169943=CARTESIAN_POINT('Ctrl Pts',(63.051523057112,-2.36415209218552,58.2543781182925));
#169944=CARTESIAN_POINT('Ctrl Pts',(63.3153768788678,-3.21011419768726,
58.2187127907996));
#169945=CARTESIAN_POINT('Ctrl Pts',(63.387727563575,-3.41803155528467,58.2085425026169));
#169946=CARTESIAN_POINT('Ctrl Pts',(63.4923558529088,-3.68986808904647,
58.1933466223143));
#169947=CARTESIAN_POINT('Ctrl Pts',(63.5186488455654,-3.75608876051431,
58.1894926708313));
#169948=CARTESIAN_POINT('Ctrl Pts',(63.562754995827,-3.86384528002755,58.1829716491946));
#169949=CARTESIAN_POINT('Ctrl Pts',(63.5801533094643,-3.90555303718801,
58.1803858908014));
#169950=CARTESIAN_POINT('Ctrl Pts',(63.6143958323984,-3.9861182813017,58.1752711946906));
#169951=CARTESIAN_POINT('Ctrl Pts',(63.6312059858349,-4.02498961629921,
58.1727489205827));
#169952=CARTESIAN_POINT('Ctrl Pts',(63.6711531772115,-4.11579397581618,
58.1667289253965));
#169953=CARTESIAN_POINT('Ctrl Pts',(63.6944839343718,-4.16763762685056,
58.1631931816089));
#169954=CARTESIAN_POINT('Ctrl Pts',(63.7728269862209,-4.33787576642266,
58.1512571571044));
#169955=CARTESIAN_POINT('Ctrl Pts',(63.8296847425617,-4.45538035961212,
58.1424950101607));
#169956=CARTESIAN_POINT('Ctrl Pts',(63.9721197247251,-4.73575072890804,
58.1203273884186));
#169957=CARTESIAN_POINT('Ctrl Pts',(64.0598888902517,-4.89741464014061,
58.1064945944065));
#169958=CARTESIAN_POINT('Ctrl Pts',(64.3181870159524,-5.34360087564587,
58.0653929460286));
#169959=CARTESIAN_POINT('Ctrl Pts',(64.498346247756,-5.62209543137918,58.0362848249265));
#169960=CARTESIAN_POINT('Ctrl Pts',(64.9253738032989,-6.2154764448889,57.9668946164429));
#169961=CARTESIAN_POINT('Ctrl Pts',(65.177942228068,-6.52543110269897,57.9256078756775));
#169962=CARTESIAN_POINT('Ctrl Pts',(65.4953116409186,-6.87025982320277,
57.8741417670288));
#169963=CARTESIAN_POINT('Ctrl Pts',(65.5428770849662,-6.92086489077495,
57.8664386989642));
#169964=CARTESIAN_POINT('Ctrl Pts',(65.6122928724757,-6.99318002316199,
57.8552169205603));
#169965=CARTESIAN_POINT('Ctrl Pts',(65.6337236303911,-7.01529876158576,
57.8517550988664));
#169966=CARTESIAN_POINT('Ctrl Pts',(65.6717032212638,-7.05413388840991,
57.8456253189166));
#169967=CARTESIAN_POINT('Ctrl Pts',(65.6882095547363,-7.07089230610177,
57.8429630033498));
#169968=CARTESIAN_POINT('Ctrl Pts',(65.7239608618288,-7.10693207814124,
57.8372005780922));
#169969=CARTESIAN_POINT('Ctrl Pts',(65.7432256460699,-7.12619281617151,
57.83409783931));
#169970=CARTESIAN_POINT('Ctrl Pts',(65.7978140033004,-7.18032156117973,
57.8253120762596));
#169971=CARTESIAN_POINT('Ctrl Pts',(65.8333185047889,-7.21500203850099,
57.8196049279966));
#169972=CARTESIAN_POINT('Ctrl Pts',(66.0884019481187,-7.46044856141768,
57.778643750801));
#169973=CARTESIAN_POINT('Ctrl Pts',(66.3172220096294,-7.66116574850118,
57.742115642975));
#169974=CARTESIAN_POINT('Ctrl Pts',(66.6741355235429,-7.94627937940034,
57.6850776785341));
#169975=CARTESIAN_POINT('Ctrl Pts',(66.795656771984,-8.0388274737182,57.6656484067713));
#169976=CARTESIAN_POINT('Ctrl Pts',(67.3416239536575,-8.43499482220052,
57.5782050164547));
#169977=CARTESIAN_POINT('Ctrl Pts',(67.7871769411349,-8.707259616821,57.5063956464762));
#169978=CARTESIAN_POINT('Ctrl Pts',(68.3458602876401,-8.99052198928067,
57.4151310169165));
#169979=CARTESIAN_POINT('Ctrl Pts',(68.4408221271113,-9.03676133096291,
57.3995805752955));
#169980=CARTESIAN_POINT('Ctrl Pts',(68.5836435478361,-9.1034786918692,57.3761349207657));
#169981=CARTESIAN_POINT('Ctrl Pts',(68.6309663536374,-9.12512849953856,
57.3683570320917));
#169982=CARTESIAN_POINT('Ctrl Pts',(68.7162379291058,-9.16332280182636,
57.3543251432075));
#169983=CARTESIAN_POINT('Ctrl Pts',(68.7541253512455,-9.18000613894365,
57.3480846627265));
#169984=CARTESIAN_POINT('Ctrl Pts',(68.835151048409,-9.21507459321868,57.3347262879021));
#169985=CARTESIAN_POINT('Ctrl Pts',(68.8783169946911,-9.23339079067513,
57.327602168644));
#169986=CARTESIAN_POINT('Ctrl Pts',(68.9958732099315,-9.28228056989534,
57.3081804450102));
#169987=CARTESIAN_POINT('Ctrl Pts',(69.0705032674212,-9.31224640300566,
57.2958287808511));
#169988=CARTESIAN_POINT('Ctrl Pts',(69.5039131815365,-9.48010684238259,
57.2239750843428));
#169989=CARTESIAN_POINT('Ctrl Pts',(69.8699434368651,-9.59761507769309,
57.1627944174484));
#169990=CARTESIAN_POINT('Ctrl Pts',(70.7046977800549,-9.81224566180213,
57.0226261791118));
#169991=CARTESIAN_POINT('Ctrl Pts',(71.1754823451742,-9.89702135037369,
56.943127860477));
#169992=CARTESIAN_POINT('Ctrl Pts',(71.9065629451082,-9.97374118967351,
56.8202660712687));
#169993=CARTESIAN_POINT('Ctrl Pts',(72.1635544045455,-9.99043491188369,
56.7771960619146));
#169994=CARTESIAN_POINT('Ctrl Pts',(72.4638390016225,-9.99799638053454,
56.7272129036606));
#169995=CARTESIAN_POINT('Ctrl Pts',(72.5067434441473,-9.99879282025211,
56.7200795451036));
#169996=CARTESIAN_POINT('Ctrl Pts',(72.5766435179477,-9.99962793240755,
56.7084726298045));
#169997=CARTESIAN_POINT('Ctrl Pts',(72.6036356969778,-9.99983810934053,
56.7039941645786));
#169998=CARTESIAN_POINT('Ctrl Pts',(72.6520740561749,-10.0000137668606,
56.6959642467719));
#169999=CARTESIAN_POINT('Ctrl Pts',(72.6735194957356,-10.0000206630978,
56.6924115360003));
#170000=CARTESIAN_POINT('Ctrl Pts',(72.7209331498144,-9.99987922188316,
56.6845622711482));
#170001=CARTESIAN_POINT('Ctrl Pts',(72.7469010484595,-9.99969784750455,
56.6802668674492));
#170002=CARTESIAN_POINT('Ctrl Pts',(72.8227959306771,-9.99886406543161,
56.6677227668892));
#170003=CARTESIAN_POINT('Ctrl Pts',(72.8727205695597,-9.99793146535694,
56.6594835245592));
#170004=CARTESIAN_POINT('Ctrl Pts',(73.3758435726986,-9.98466117497393,
56.576563725556));
#170005=CARTESIAN_POINT('Ctrl Pts',(73.8278499941925,-9.94106877638808,
56.5029639906997));
#170006=CARTESIAN_POINT('Ctrl Pts',(74.8830774561407,-9.76438491859643,
56.3313547789217));
#170007=CARTESIAN_POINT('Ctrl Pts',(75.4801487879644,-9.60520653377018,
56.2343562112766));
#170008=CARTESIAN_POINT('Ctrl Pts',(76.1599006764834,-9.35309385969277,
56.1229326415212));
#170009=CARTESIAN_POINT('Ctrl Pts',(76.2606488274134,-9.31381502937074,
56.1063948971864));
#170010=CARTESIAN_POINT('Ctrl Pts',(76.4093722967137,-9.25297269280181,
56.0819462958496));
#170011=CARTESIAN_POINT('Ctrl Pts',(76.4578493448498,-9.23268351977169,
56.0739714743553));
#170012=CARTESIAN_POINT('Ctrl Pts',(76.5442655521862,-9.19569490465986,
56.0597452573067));
#170013=CARTESIAN_POINT('Ctrl Pts',(76.582265400249,-9.17914354506159,56.0534860212888));
#170014=CARTESIAN_POINT('Ctrl Pts',(76.662733897872,-9.14348473599334,56.0402240603206));
#170015=CARTESIAN_POINT('Ctrl Pts',(76.7051741766732,-9.12431440210388,
56.0332250944577));
#170016=CARTESIAN_POINT('Ctrl Pts',(76.8192088606804,-9.07182229533657,
56.0144076765153));
#170017=CARTESIAN_POINT('Ctrl Pts',(76.8905443574619,-9.03793411881336,
56.0026238439549));
#170018=CARTESIAN_POINT('Ctrl Pts',(77.294379380416,-8.8400726263574,55.9358490144783));
#170019=CARTESIAN_POINT('Ctrl Pts',(77.6179324326154,-8.65812295719163,
55.8820784201954));
#170020=CARTESIAN_POINT('Ctrl Pts',(78.3568205450506,-8.18570995922695,
55.7591205998082));
#170021=CARTESIAN_POINT('Ctrl Pts',(78.7617517939312,-7.88053094833642,
55.691587052926));
#170022=CARTESIAN_POINT('Ctrl Pts',(79.2595628825674,-7.44176684154383,
55.6097044574082));
#170023=CARTESIAN_POINT('Ctrl Pts',(79.3746489419549,-7.33539418497803,
55.5908668217293));
#170024=CARTESIAN_POINT('Ctrl Pts',(79.5184516421845,-7.19604766322438,
55.5674992029213));
#170025=CARTESIAN_POINT('Ctrl Pts',(79.5494841927515,-7.16558071303746,
55.5624669976062));
#170026=CARTESIAN_POINT('Ctrl Pts',(79.5986880010373,-7.11663802463973,
55.5545064441688));
#170027=CARTESIAN_POINT('Ctrl Pts',(79.6169859080969,-7.09829497280259,
55.5515501662155));
#170028=CARTESIAN_POINT('Ctrl Pts',(79.6520420155991,-7.06287781121129,
55.5458946322542));
#170029=CARTESIAN_POINT('Ctrl Pts',(79.6688103981895,-7.0458145758536,55.5431931310169));
#170030=CARTESIAN_POINT('Ctrl Pts',(79.7092992155928,-7.00431669816306,
55.5366788472391));
#170031=CARTESIAN_POINT('Ctrl Pts',(79.7329574480326,-6.97981957529539,
55.5328797719419));
#170032=CARTESIAN_POINT('Ctrl Pts',(79.8167546461673,-6.89215860614009,
55.5194482893337));
#170033=CARTESIAN_POINT('Ctrl Pts',(79.8762029944654,-6.82831717449719,
55.5099654624862));
#170034=CARTESIAN_POINT('Ctrl Pts',(80.2654567943855,-6.39917042824931,
55.4481406223644));
#170035=CARTESIAN_POINT('Ctrl Pts',(80.5691244801292,-6.01030280750111,
55.4011696219501));
#170036=CARTESIAN_POINT('Ctrl Pts',(81.1059286353248,-5.20715384881265,
55.3190374995395));
#170037=CARTESIAN_POINT('Ctrl Pts',(81.3407739365141,-4.79559158778963,
55.2835699601268));
#170038=CARTESIAN_POINT('Ctrl Pts',(81.5813692407573,-4.29480132520669,
55.2474101480165));
#170039=CARTESIAN_POINT('Ctrl Pts',(81.6159819879548,-4.22043965619088,
55.2422143900577));
#170040=CARTESIAN_POINT('Ctrl Pts',(81.6693956263758,-4.10191913313227,
55.2342059164948));
#170041=CARTESIAN_POINT('Ctrl Pts',(81.6887942776036,-4.05804016770877,
55.2312995314776));
#170042=CARTESIAN_POINT('Ctrl Pts',(81.7244750411608,-3.9757456640287,55.2259576692539));
#170043=CARTESIAN_POINT('Ctrl Pts',(81.7408332130592,-3.9373650215457,55.2235102786188));
#170044=CARTESIAN_POINT('Ctrl Pts',(81.776894506749,-3.85127593701282,55.2181187978181));
#170045=CARTESIAN_POINT('Ctrl Pts',(81.7964707630272,-3.80351441661973,
55.2151945746701));
#170046=CARTESIAN_POINT('Ctrl Pts',(81.8535494830644,-3.66114671806651,
55.2066765301363));
#170047=CARTESIAN_POINT('Ctrl Pts',(81.8899898239298,-3.56611211345595,
55.2012492136946));
#170048=CARTESIAN_POINT('Ctrl Pts',(82.0515992273742,-3.12476080096068,
55.1772383375035));
#170049=CARTESIAN_POINT('Ctrl Pts',(82.1592191029732,-2.77217906562558,
55.1614089315373));
#170050=CARTESIAN_POINT('Ctrl Pts',(82.36570613699,-1.93426587403167,55.1319065367559));
#170051=CARTESIAN_POINT('Ctrl Pts',(82.4487044914181,-1.44593827026146,
55.1208490837898));
#170052=CARTESIAN_POINT('Ctrl Pts',(82.5184624369535,-0.717290300203294,
55.1145636378729));
#170053=CARTESIAN_POINT('Ctrl Pts',(82.5328076145551,-0.480419027492485,
55.1141011166423));
#170054=CARTESIAN_POINT('Ctrl Pts',(82.5400830901692,-0.196583885451342,
55.1155871992899));
#170055=CARTESIAN_POINT('Ctrl Pts',(82.5409593326823,-0.149890911920435,
55.1158977099975));
#170056=CARTESIAN_POINT('Ctrl Pts',(82.5418222043871,-0.0774114079091971,
55.1164838218244));
#170057=CARTESIAN_POINT('Ctrl Pts',(82.542031498269,-0.0516278227723996,
55.1167127713156));
#170058=CARTESIAN_POINT('Ctrl Pts',(82.5422374743968,-0.00406986241077593,
55.117173116348));
#170059=CARTESIAN_POINT('Ctrl Pts',(82.5422621641968,0.0177040968224466,
55.1173986213876));
#170060=CARTESIAN_POINT('Ctrl Pts',(82.5421594085252,0.067502478009366,
55.1179480115738));
#170061=CARTESIAN_POINT('Ctrl Pts',(82.5419862478804,0.0955264069625877,
55.1182815174849));
#170062=CARTESIAN_POINT('Ctrl Pts',(82.5410884065857,0.182727385267187,
55.1193943434771));
#170063=CARTESIAN_POINT('Ctrl Pts',(82.5399646040612,0.24189799222242,55.1202570439598));
#170064=CARTESIAN_POINT('Ctrl Pts',(82.5284537721331,0.657481339120658,
55.127058210742));
#170065=CARTESIAN_POINT('Ctrl Pts',(82.4999028638073,1.01307791450742,55.1367050025745));
#170066=CARTESIAN_POINT('Ctrl Pts',(82.3693581444211,1.99061937926038,55.1727907434886));
#170067=CARTESIAN_POINT('Ctrl Pts',(82.2280915529031,2.60540559057014,55.2062710267115));
#170068=CARTESIAN_POINT('Ctrl Pts',(81.9790179784828,3.35843425536561,55.2596607528521));
#170069=CARTESIAN_POINT('Ctrl Pts',(81.9236286927221,3.51308753212645,55.2713228690378));
#170070=CARTESIAN_POINT('Ctrl Pts',(81.8414556958688,3.72594593875938,55.2883452535917));
#170071=CARTESIAN_POINT('Ctrl Pts',(81.8178529871186,3.7853900947735,55.2932061671777));
#170072=CARTESIAN_POINT('Ctrl Pts',(81.7788519556088,3.88094466827754,55.3011935461263));
#170073=CARTESIAN_POINT('Ctrl Pts',(81.7638051168413,3.91720114435001,55.3042649178868));
#170074=CARTESIAN_POINT('Ctrl Pts',(81.7320016400795,3.9925823682761,55.3107357674994));
#170075=CARTESIAN_POINT('Ctrl Pts',(81.7152081887932,4.03169022845718,55.3141409961434));
#170076=CARTESIAN_POINT('Ctrl Pts',(81.6747815137863,4.12420665607056,55.3223113736718));
#170077=CARTESIAN_POINT('Ctrl Pts',(81.6509308844624,4.17751547634108,55.3271105516552));
#170078=CARTESIAN_POINT('Ctrl Pts',(81.5682003551724,4.35817921792623,55.3436879950985));
#170079=CARTESIAN_POINT('Ctrl Pts',(81.5071263502993,4.48447901614293,55.355810095591));
#170080=CARTESIAN_POINT('Ctrl Pts',(81.3511528490271,4.79046998160984,55.3865136163936));
#170081=CARTESIAN_POINT('Ctrl Pts',(81.2534157799658,4.96859735987704,55.4055433672032));
#170082=CARTESIAN_POINT('Ctrl Pts',(80.9851819307598,5.42402265031676,55.4573442314821));
#170083=CARTESIAN_POINT('Ctrl Pts',(80.8065134062264,5.69606906909182,55.4914455289004));
#170084=CARTESIAN_POINT('Ctrl Pts',(80.3967337304052,6.25818605272208,55.5693431935936));
#170085=CARTESIAN_POINT('Ctrl Pts',(80.1621039954986,6.5449929738467,55.6137668227995));
#170086=CARTESIAN_POINT('Ctrl Pts',(79.8652577993506,6.86921362961989,55.6703321294969));
#170087=CARTESIAN_POINT('Ctrl Pts',(79.8176462414156,6.9201306466871,55.6794152288931));
#170088=CARTESIAN_POINT('Ctrl Pts',(79.7482426718977,6.99280623729642,55.692675888029));
#170089=CARTESIAN_POINT('Ctrl Pts',(79.7268701895026,7.01497914300828,55.6967621478398));
#170090=CARTESIAN_POINT('Ctrl Pts',(79.689028522474,7.05387474754867,55.7040024995843));
#170091=CARTESIAN_POINT('Ctrl Pts',(79.6726016416218,7.07063992037553,55.7071472615729));
#170092=CARTESIAN_POINT('Ctrl Pts',(79.6370636557936,7.10665370053121,55.7139545963237));
#170093=CARTESIAN_POINT('Ctrl Pts',(79.6179333442399,7.12588201297431,55.717621405733));
#170094=CARTESIAN_POINT('Ctrl Pts',(79.5638236424908,7.17982516049554,55.7279990097966));
#170095=CARTESIAN_POINT('Ctrl Pts',(79.5286679709258,7.21435457459367,55.7347485820397));
#170096=CARTESIAN_POINT('Ctrl Pts',(79.2806318909866,7.45436781747725,55.7824104906476));
#170097=CARTESIAN_POINT('Ctrl Pts',(79.0590916404481,7.65031679717258,55.8251877210789));
#170098=CARTESIAN_POINT('Ctrl Pts',(78.6855425032289,7.95191588266032,55.8972625421681));
#170099=CARTESIAN_POINT('Ctrl Pts',(78.5386494144109,8.06383570001938,55.9255934010245));
#170100=CARTESIAN_POINT('Ctrl Pts',(77.9857252992693,8.46098497094117,56.0320252309737));
#170101=CARTESIAN_POINT('Ctrl Pts',(77.5617691642608,8.71914883231862,56.1131883450019));
#170102=CARTESIAN_POINT('Ctrl Pts',(77.0270211150753,8.99132431623913,56.214442476174));
#170103=CARTESIAN_POINT('Ctrl Pts',(76.9328991340914,9.03733379015971,56.232226779589));
#170104=CARTESIAN_POINT('Ctrl Pts',(76.7911937366267,9.10379148725305,56.2589442000974));
#170105=CARTESIAN_POINT('Ctrl Pts',(76.744148715745,9.12539858463339,56.2678048108245));
#170106=CARTESIAN_POINT('Ctrl Pts',(76.6593118972396,9.16354591623723,56.2837664202998));
#170107=CARTESIAN_POINT('Ctrl Pts',(76.6215817979544,9.18022371872653,56.2908592176795));
#170108=CARTESIAN_POINT('Ctrl Pts',(76.5408231107731,9.21530890529264,56.306028269109));
#170109=CARTESIAN_POINT('Ctrl Pts',(76.4977660082422,9.23364645062245,56.3141081874362));
#170110=CARTESIAN_POINT('Ctrl Pts',(76.3803325595405,9.28266137018431,56.3361248906341));
#170111=CARTESIAN_POINT('Ctrl Pts',(76.3057101334162,9.31272522592874,56.3500931761443));
#170112=CARTESIAN_POINT('Ctrl Pts',(75.8677429585852,9.48288271822146,56.4319498893773));
#170113=CARTESIAN_POINT('Ctrl Pts',(75.4967672066577,9.60189231068149,56.5007695016574));
#170114=CARTESIAN_POINT('Ctrl Pts',(74.6190035087891,9.82627414220338,56.6629255858309));
#170115=CARTESIAN_POINT('Ctrl Pts',(74.1090010404577,9.9139791814594,56.7566193574042));
#170116=CARTESIAN_POINT('Ctrl Pts',(73.3821043927746,9.97982027830171,56.8909620903642));
#170117=CARTESIAN_POINT('Ctrl Pts',(73.1689767994582,9.99203300209417,56.9304551465251));
#170118=CARTESIAN_POINT('Ctrl Pts',(72.9108781725562,9.99826499384839,56.9785305129153));
#170119=CARTESIAN_POINT('Ctrl Pts',(72.8660864449013,9.9990350127156,56.9868828604909));
#170120=CARTESIAN_POINT('Ctrl Pts',(72.7961966441963,9.9997505189866,56.9999310520931));
#170121=CARTESIAN_POINT('Ctrl Pts',(72.7711000501385,9.99990968278211,57.0046196784292));
#170122=CARTESIAN_POINT('Ctrl Pts',(72.7245706896034,10.000023516907,57.0133186662311));
#170123=CARTESIAN_POINT('Ctrl Pts',(72.7031381657225,10.0000046453583,57.017328106088));
#170124=CARTESIAN_POINT('Ctrl Pts',(72.6538099972462,9.99979709104262,57.0265616795334));
#170125=CARTESIAN_POINT('Ctrl Pts',(72.6259151227576,9.99955890718432,57.031787332499));
#170126=CARTESIAN_POINT('Ctrl Pts',(72.5380082847686,9.99842753651006,57.0482674696931));
#170127=CARTESIAN_POINT('Ctrl Pts',(72.4780056813453,9.99709594715378,57.0595342623081));
#170128=CARTESIAN_POINT('Ctrl Pts',(72.1678310260054,9.9873196631852,57.1178574717189));
#170129=CARTESIAN_POINT('Ctrl Pts',(71.9180754197389,9.96971219509977,57.1650910686456));
#170130=CARTESIAN_POINT('Ctrl Pts',(71.0949147371838,9.87942124999785,57.3211753669735));
#170131=CARTESIAN_POINT('Ctrl Pts',(70.5272285833151,9.76499279507884,57.4294072747857));
#170132=CARTESIAN_POINT('Ctrl Pts',(69.709555302367,9.52242286805878,57.5844563228087));
#170133=CARTESIAN_POINT('Ctrl Pts',(69.449809219873,9.43322358138652,57.6335928422547));
#170134=CARTESIAN_POINT('Ctrl Pts',(69.123153735291,9.30534335455554,57.6951851272823));
#170135=CARTESIAN_POINT('Ctrl Pts',(69.0525869852108,9.27675857013407,57.708478823019));
#170136=CARTESIAN_POINT('Ctrl Pts',(68.9400487320975,9.22962860307571,57.7296599863014));
#170137=CARTESIAN_POINT('Ctrl Pts',(68.8978680044398,9.21161260570685,57.737594559924));
#170138=CARTESIAN_POINT('Ctrl Pts',(68.8178424315244,9.17676250994397,57.7526398146157));
#170139=CARTESIAN_POINT('Ctrl Pts',(68.7799753955317,9.159984054687,57.7597554747274));
#170140=CARTESIAN_POINT('Ctrl Pts',(68.6935870036067,9.12104602755132,57.7759808751572));
#170141=CARTESIAN_POINT('Ctrl Pts',(68.6451358145953,9.09872760615646,57.7850751287797));
#170142=CARTESIAN_POINT('Ctrl Pts',(68.4945579049635,9.02786332643967,57.8133210033127));
#170143=CARTESIAN_POINT('Ctrl Pts',(68.3930688989171,8.97792949421522,57.8323332394945));
#170144=CARTESIAN_POINT('Ctrl Pts',(68.156792612989,8.85653796600411,57.8765433841998));
#170145=CARTESIAN_POINT('Ctrl Pts',(68.0227424250005,8.7836544029474,57.9015848552352));
#170146=CARTESIAN_POINT('Ctrl Pts',(67.5529805814227,8.5138251428777,57.9892385214302));
#170147=CARTESIAN_POINT('Ctrl Pts',(67.2270851262614,8.2998876278944,58.0498458996509));
#170148=CARTESIAN_POINT('Ctrl Pts',(66.6024224090205,7.83440640497587,58.166329045405));
#170149=CARTESIAN_POINT('Ctrl Pts',(66.3041566991107,7.58333536755529,58.2221142573581));
#170150=CARTESIAN_POINT('Ctrl Pts',(65.9709412225519,7.26723809998258,58.2852877854289));
#170151=CARTESIAN_POINT('Ctrl Pts',(65.9210449741039,7.21889309525724,58.2947720915488));
#170152=CARTESIAN_POINT('Ctrl Pts',(65.8497981041605,7.14838578179475,58.3083557289708));
#170153=CARTESIAN_POINT('Ctrl Pts',(65.8280388590372,7.12664997538445,58.3125098834334));
#170154=CARTESIAN_POINT('Ctrl Pts',(65.7898563794477,7.08815002738781,58.3198099923265));
#170155=CARTESIAN_POINT('Ctrl Pts',(65.7733911826969,7.07142897802047,58.3229614834389));
#170156=CARTESIAN_POINT('Ctrl Pts',(65.7380063528217,7.03523680009847,58.3297420081264));
#170157=CARTESIAN_POINT('Ctrl Pts',(65.7191069858698,7.01574588818218,58.3333683241492));
#170158=CARTESIAN_POINT('Ctrl Pts',(65.6660498163799,6.96057423594438,58.3435616133775));
#170159=CARTESIAN_POINT('Ctrl Pts',(65.6320768112236,6.92471230592477,58.3501037315673));
#170160=CARTESIAN_POINT('Ctrl Pts',(65.3941801561929,6.66978454220652,58.3960151122375));
#170161=CARTESIAN_POINT('Ctrl Pts',(65.1999126399328,6.44167428638077,58.4340268129339));
#170162=CARTESIAN_POINT('Ctrl Pts',(64.8953545935545,6.0494185559447,58.494129225884));
#170163=CARTESIAN_POINT('Ctrl Pts',(64.7791764599942,5.89024522052992,58.5171977332535));
#170164=CARTESIAN_POINT('Ctrl Pts',(64.3949240343878,5.32963174731759,58.5938173902111));
#170165=CARTESIAN_POINT('Ctrl Pts',(64.1510011920082,4.91187413749828,58.6430027651904));
#170166=CARTESIAN_POINT('Ctrl Pts',(63.8907038042634,4.38171435947856,58.6956908542953));
#170167=CARTESIAN_POINT('Ctrl Pts',(63.8450986501178,4.28496424950862,58.7049332183592));
#170168=CARTESIAN_POINT('Ctrl Pts',(63.7793845204544,4.13960006292655,58.7182660761189));
#170169=CARTESIAN_POINT('Ctrl Pts',(63.7581100322123,4.09154250133929,58.722585059913));
#170170=CARTESIAN_POINT('Ctrl Pts',(63.7206120703256,4.00501739563649,58.7302022026168));
#170171=CARTESIAN_POINT('Ctrl Pts',(63.7042508187716,3.96661331139702,58.7335273878648));
#170172=CARTESIAN_POINT('Ctrl Pts',(63.6698932217707,3.8845596669075,58.7405136426863));
#170173=CARTESIAN_POINT('Ctrl Pts',(63.651963444165,3.84088223479076,58.7441616501512));
#170174=CARTESIAN_POINT('Ctrl Pts',(63.6041854470681,3.72213077575406,58.7538887626634));
#170175=CARTESIAN_POINT('Ctrl Pts',(63.5749270371223,3.64681390896773,58.7598522213024));
#170176=CARTESIAN_POINT('Ctrl Pts',(63.4129784474172,3.21464798949199,58.7929039423211));
#170177=CARTESIAN_POINT('Ctrl Pts',(63.2995269445804,2.85064300111895,58.8162156015133));
#170178=CARTESIAN_POINT('Ctrl Pts',(63.0919972856453,2.02311697307081,58.8596972888563));
#170179=CARTESIAN_POINT('Ctrl Pts',(63.0092314806177,1.55759522967024,58.8777327922444));
#170180=CARTESIAN_POINT('Ctrl Pts',(62.9302613801214,0.815305549533786,
58.8976634002474));
#170181=CARTESIAN_POINT('Ctrl Pts',(62.9123390074276,0.541662011403782,
58.903155357785));
#170182=CARTESIAN_POINT('Ctrl Pts',(62.9043127956501,0.216805783682938,
58.9077169601091));
#170183=CARTESIAN_POINT('Ctrl Pts',(62.9034409778222,0.165998276538289,
58.9083738091881));
#170184=CARTESIAN_POINT('Ctrl Pts',(62.902750607283,0.0941525551497413,
58.9092245670084));
#170185=CARTESIAN_POINT('Ctrl Pts',(62.9026142197142,0.0731187293514479,
58.9094641778581));
#170186=CARTESIAN_POINT('Ctrl Pts',(62.9024852494696,0.0347198170549746,
58.9098845147619));
#170187=CARTESIAN_POINT('Ctrl Pts',(62.9024717297551,0.0173649150417452,
58.9100681158787));
#170188=CARTESIAN_POINT('Ctrl Pts',(62.9025030071408,2.40572005160039E-14,
58.910245498748));
#170189=CARTESIAN_POINT('Origin',(72.2537026314029,-4.33680868994202E-16,
54.3558290880045));
#170190=CARTESIAN_POINT('',(63.0200955324887,3.15100886788204E-11,59.5771458498765));
#170191=CARTESIAN_POINT('',(63.0153743226244,-1.95014612637774E-11,59.5503705382064));
#170192=CARTESIAN_POINT('',(62.4056251012807,-1.65832766814156E-15,56.0923108646735));
#170193=CARTESIAN_POINT('Ctrl Pts',(63.0200955324887,6.3021835685309E-11,
59.5771458498765));
#170194=CARTESIAN_POINT('Ctrl Pts',(63.0200725474665,0.0127610715955115,
59.5770154953381));
#170195=CARTESIAN_POINT('Ctrl Pts',(63.0200734724794,0.0255221090800886,
59.576880073832));
#170196=CARTESIAN_POINT('Ctrl Pts',(63.0201524332212,0.066088450096215,
59.5764335355938));
#170197=CARTESIAN_POINT('Ctrl Pts',(63.0203200911363,0.0938931878456895,
59.5761035105159));
#170198=CARTESIAN_POINT('Ctrl Pts',(63.0210563120057,0.166679807240136,
59.5751773968722));
#170199=CARTESIAN_POINT('Ctrl Pts',(63.0218085748546,0.211658719543653,
59.5745429231689));
#170200=CARTESIAN_POINT('Ctrl Pts',(63.0318781755434,0.643092600572684,
59.567868938244));
#170201=CARTESIAN_POINT('Ctrl Pts',(63.0628517303118,1.02865278076536,59.5573874701675));
#170202=CARTESIAN_POINT('Ctrl Pts',(63.1244481546801,1.47466085631702,59.5405490389491));
#170203=CARTESIAN_POINT('Ctrl Pts',(63.1337863823996,1.53786632840428,59.5380510306884));
#170204=CARTESIAN_POINT('Ctrl Pts',(63.2020388676492,1.97144933253191,59.5201581944454));
#170205=CARTESIAN_POINT('Ctrl Pts',(63.2808465391425,2.33825051061519,59.501233195767));
#170206=CARTESIAN_POINT('Ctrl Pts',(63.4345194487925,2.89938029904544,59.4667508594033));
#170207=CARTESIAN_POINT('Ctrl Pts',(63.4953438866782,3.09733408131394,59.4534788043003));
#170208=CARTESIAN_POINT('Ctrl Pts',(63.60869344673,3.42939836644478,59.4293569762587));
#170209=CARTESIAN_POINT('Ctrl Pts',(63.6580860047928,3.5645425751919,59.4190040033843));
#170210=CARTESIAN_POINT('Ctrl Pts',(63.731804417628,3.75355983427328,59.4037655723795));
#170211=CARTESIAN_POINT('Ctrl Pts',(63.7537414668091,3.8083751020046,59.3992549797151));
#170212=CARTESIAN_POINT('Ctrl Pts',(63.7923640705684,3.90246997818028,59.3913540242616));
#170213=CARTESIAN_POINT('Ctrl Pts',(63.8088201902371,3.94184501349841,59.3879996285045));
#170214=CARTESIAN_POINT('Ctrl Pts',(63.8408413783315,4.01711071388268,59.3814950190118));
#170215=CARTESIAN_POINT('Ctrl Pts',(63.8563664103702,4.05301809162716,59.3783510896961));
#170216=CARTESIAN_POINT('Ctrl Pts',(63.8934289989786,4.13738156008773,59.3708681323689));
#170217=CARTESIAN_POINT('Ctrl Pts',(63.9151406080702,4.18575744968697,59.3665018551243));
#170218=CARTESIAN_POINT('Ctrl Pts',(63.9927705024863,4.35511838983164,59.3509491532393));
#170219=CARTESIAN_POINT('Ctrl Pts',(64.0507046718079,4.47513439168626,59.3394467526492));
#170220=CARTESIAN_POINT('Ctrl Pts',(64.4036239622151,5.17047517097404,59.2699285699411));
#170221=CARTESIAN_POINT('Ctrl Pts',(64.7510267557267,5.71661901636454,59.2037523954328));
#170222=CARTESIAN_POINT('Ctrl Pts',(65.2702382611678,6.38104844216386,59.105195547197));
#170223=CARTESIAN_POINT('Ctrl Pts',(65.3970616580142,6.53371361209762,59.0811330238426));
#170224=CARTESIAN_POINT('Ctrl Pts',(65.6043998917974,6.76865856833162,59.0416941892472));
#170225=CARTESIAN_POINT('Ctrl Pts',(65.6819806544808,6.85355585452661,59.0269163799176));
#170226=CARTESIAN_POINT('Ctrl Pts',(65.786912671263,6.96446143353585,59.0068804632743));
#170227=CARTESIAN_POINT('Ctrl Pts',(65.8129905191862,6.99171158349314,59.0018972686762));
#170228=CARTESIAN_POINT('Ctrl Pts',(65.8563328032513,7.03648948561407,58.9936077571816));
#170229=CARTESIAN_POINT('Ctrl Pts',(65.8735101909773,7.05410449957666,58.9903206007854));
#170230=CARTESIAN_POINT('Ctrl Pts',(65.9060294875375,7.0872055493029,58.9840937279618));
#170231=CARTESIAN_POINT('Ctrl Pts',(65.9213575821644,7.10270551488825,58.981157091306));
#170232=CARTESIAN_POINT('Ctrl Pts',(65.9578844696464,7.1393996360552,58.9741555977358));
#170233=CARTESIAN_POINT('Ctrl Pts',(65.9791275021735,7.16054758509237,58.9700809589307));
#170234=CARTESIAN_POINT('Ctrl Pts',(66.054620891919,7.2350253742697,58.9555917550626));
#170235=CARTESIAN_POINT('Ctrl Pts',(66.1093774784722,7.28781675062998,58.9450666102771));
#170236=CARTESIAN_POINT('Ctrl Pts',(66.5271055983632,7.68137623445971,58.8646861741246));
#170237=CARTESIAN_POINT('Ctrl Pts',(66.9141798820333,7.99448239303505,58.7897578417173));
#170238=CARTESIAN_POINT('Ctrl Pts',(67.6560476066799,8.50668288704805,58.6471537347899));
#170239=CARTESIAN_POINT('Ctrl Pts',(68.0029144129277,8.71567093317399,58.5808209125774));
#170240=CARTESIAN_POINT('Ctrl Pts',(68.4721288828255,8.96000116052806,58.4918673758555));
#170241=CARTESIAN_POINT('Ctrl Pts',(68.5838254793688,9.01546452084471,58.4707447128195));
#170242=CARTESIAN_POINT('Ctrl Pts',(68.746635960045,9.09244628268166,58.4400352861272));
#170243=CARTESIAN_POINT('Ctrl Pts',(68.7969337125674,9.11570503057861,58.4305587995762));
#170244=CARTESIAN_POINT('Ctrl Pts',(68.8854225510539,9.15571012431528,58.4139056431212));
#170245=CARTESIAN_POINT('Ctrl Pts',(68.9235294953462,9.17264369028485,58.4067401664302));
#170246=CARTESIAN_POINT('Ctrl Pts',(69.0028875627831,9.20729858224362,58.391830532333));
#170247=CARTESIAN_POINT('Ctrl Pts',(69.0441545719024,9.22498019748003,58.3840843505093));
#170248=CARTESIAN_POINT('Ctrl Pts',(69.1515952660724,9.27013693690292,58.3639347322885));
#170249=CARTESIAN_POINT('Ctrl Pts',(69.2179491666316,9.29716580507235,58.3515081798939));
#170250=CARTESIAN_POINT('Ctrl Pts',(69.4977224032043,9.40753849723099,58.2991848456211));
#170251=CARTESIAN_POINT('Ctrl Pts',(69.7137035787971,9.48403241842706,58.2589680535346));
#170252=CARTESIAN_POINT('Ctrl Pts',(70.4659955958567,9.72086709788736,58.1193759273193));
#170253=CARTESIAN_POINT('Ctrl Pts',(71.0131274055265,9.84233992992407,58.0187520952213));
#170254=CARTESIAN_POINT('Ctrl Pts',(71.9076142730117,9.96105120379876,57.853835515361));
#170255=CARTESIAN_POINT('Ctrl Pts',(72.2499154079977,9.98806845090927,57.7906110908165));
#170256=CARTESIAN_POINT('Ctrl Pts',(72.6408216794739,9.99806751111475,57.717814278986));
#170257=CARTESIAN_POINT('Ctrl Pts',(72.6888405749281,9.99893776090644,57.7088615752299));
#170258=CARTESIAN_POINT('Ctrl Pts',(72.7623751522576,9.99972226265001,57.6951339437845));
#170259=CARTESIAN_POINT('Ctrl Pts',(72.7878889425738,9.99989341218551,57.6903676886638));
#170260=CARTESIAN_POINT('Ctrl Pts',(72.834791906369,10.0000222929586,57.6815993378657));
#170261=CARTESIAN_POINT('Ctrl Pts',(72.8561808303874,10.0000100498126,57.6775982866506));
#170262=CARTESIAN_POINT('Ctrl Pts',(72.9048981475929,9.99982040624204,57.668479578266));
#170263=CARTESIAN_POINT('Ctrl Pts',(72.9322257985338,9.99959807913916,57.6633605519435));
#170264=CARTESIAN_POINT('Ctrl Pts',(73.0037561063897,9.99871261001218,57.6499516970127));
#170265=CARTESIAN_POINT('Ctrl Pts',(73.0479548171807,9.99786201729911,57.6416565741571));
#170266=CARTESIAN_POINT('Ctrl Pts',(73.4099763817827,9.98840867005868,57.5736404734468));
#170267=CARTESIAN_POINT('Ctrl Pts',(73.7271459028565,9.96442351984042,57.5135977983781));
#170268=CARTESIAN_POINT('Ctrl Pts',(74.4504101346565,9.87365868581348,57.3763235104288));
#170269=CARTESIAN_POINT('Ctrl Pts',(74.8546426124419,9.79649047268983,57.2993521284652));
#170270=CARTESIAN_POINT('Ctrl Pts',(75.624078641156,9.59810386722078,57.1532135676406));
#170271=CARTESIAN_POINT('Ctrl Pts',(75.9894061101993,9.48042539736496,57.0839962767843));
#170272=CARTESIAN_POINT('Ctrl Pts',(76.421830377561,9.31230178869978,57.0024463705009));
#170273=CARTESIAN_POINT('Ctrl Pts',(76.4961996639025,9.28232466602108,56.9884344754596));
#170274=CARTESIAN_POINT('Ctrl Pts',(76.6133316644212,9.2334203758568,56.9663868419319));
#170275=CARTESIAN_POINT('Ctrl Pts',(76.6563342218514,9.21510171964711,56.9582970731907));
#170276=CARTESIAN_POINT('Ctrl Pts',(76.7370456058939,9.18003133349796,56.9431219147273));
#170277=CARTESIAN_POINT('Ctrl Pts',(76.7747821271544,9.16334864282998,56.9360303150169));
#170278=CARTESIAN_POINT('Ctrl Pts',(76.8597042814401,9.12515981145408,56.9200792332432));
#170279=CARTESIAN_POINT('Ctrl Pts',(76.9068286858055,9.10351495763508,56.9112332694498));
#170280=CARTESIAN_POINT('Ctrl Pts',(77.0490177255479,9.03682791653516,56.8845583340145));
#170281=CARTESIAN_POINT('Ctrl Pts',(77.1435467068324,8.99061527782845,56.866846542855));
#170282=CARTESIAN_POINT('Ctrl Pts',(77.6834509451405,8.71577609037926,56.7657979866849));
#170283=CARTESIAN_POINT('Ctrl Pts',(78.112011588744,8.4544617415982,56.6860828841022));
#170284=CARTESIAN_POINT('Ctrl Pts',(78.6646071992033,8.05645938193661,56.5831095517263));
#170285=CARTESIAN_POINT('Ctrl Pts',(78.8071940338766,7.94772210851001,56.5565151880089));
#170286=CARTESIAN_POINT('Ctrl Pts',(79.1765177655816,7.64975983644815,56.4874419441431));
#170287=CARTESIAN_POINT('Ctrl Pts',(79.3979494635795,7.45405364147757,56.4458325825213));
#170288=CARTESIAN_POINT('Ctrl Pts',(79.6457820614942,7.21432026774304,56.3987302495511));
#170289=CARTESIAN_POINT('Ctrl Pts',(79.6809386501648,7.17979880808279,56.3920351807516));
#170290=CARTESIAN_POINT('Ctrl Pts',(79.7350467617612,7.12586553635874,56.381708283254));
#170291=CARTESIAN_POINT('Ctrl Pts',(79.7541771939084,7.10663893262867,56.378052626661));
#170292=CARTESIAN_POINT('Ctrl Pts',(79.7897149771513,7.07062652718713,56.3712528637551));
#170293=CARTESIAN_POINT('Ctrl Pts',(79.8061418208554,7.05386099147639,56.3681061779679));
#170294=CARTESIAN_POINT('Ctrl Pts',(79.8439836437523,7.01496214691912,56.3608491094447));
#170295=CARTESIAN_POINT('Ctrl Pts',(79.8653556327152,6.99278636367774,56.3567444428635));
#170296=CARTESIAN_POINT('Ctrl Pts',(79.9347623082586,6.92009136902349,56.3433953463245));
#170297=CARTESIAN_POINT('Ctrl Pts',(79.982371018843,6.86915774106412,56.3342087701811));
#170298=CARTESIAN_POINT('Ctrl Pts',(80.2831316796237,6.54048824753826,56.2760020315854));
#170299=CARTESIAN_POINT('Ctrl Pts',(80.5210075049209,6.24879826543211,56.2291860027564));
#170300=CARTESIAN_POINT('Ctrl Pts',(80.98578074023,5.60788510940501,56.1369044189581));
#170301=CARTESIAN_POINT('Ctrl Pts',(81.208562615949,5.25645545567287,56.0921734593324));
#170302=CARTESIAN_POINT('Ctrl Pts',(81.4807659378698,4.7615137759443,56.0372790041854));
#170303=CARTESIAN_POINT('Ctrl Pts',(81.5495638146891,4.62956491761264,56.0233770716545));
#170304=CARTESIAN_POINT('Ctrl Pts',(81.6647007485787,4.39626213774363,56.000075169186));
#170305=CARTESIAN_POINT('Ctrl Pts',(81.7123217058328,4.29559588105244,55.9904252154799));
#170306=CARTESIAN_POINT('Ctrl Pts',(81.7803023764543,4.14550752139422,55.976633242519));
#170307=CARTESIAN_POINT('Ctrl Pts',(81.8019443117779,4.09669899714031,55.9722398626085));
#170308=CARTESIAN_POINT('Ctrl Pts',(81.8398498885169,4.00934711780903,55.9645402070295));
#170309=CARTESIAN_POINT('Ctrl Pts',(81.8562622940335,3.97087230805014,55.9612047501161));
#170310=CARTESIAN_POINT('Ctrl Pts',(81.890494070927,3.88922221549536,55.9542443416167));
#170311=CARTESIAN_POINT('Ctrl Pts',(81.908254331894,3.84602225758879,55.9506309892101));
#170312=CARTESIAN_POINT('Ctrl Pts',(81.9550388206692,3.72994120115857,55.9411066696293));
#170313=CARTESIAN_POINT('Ctrl Pts',(81.9835180311332,3.65683531215262,55.935302570212));
#170314=CARTESIAN_POINT('Ctrl Pts',(82.1162483636415,3.30402955169802,55.9082178837333));
#170315=CARTESIAN_POINT('Ctrl Pts',(82.2089887140146,3.01999254132958,55.8891936318053));
#170316=CARTESIAN_POINT('Ctrl Pts',(82.4410812536873,2.1857865052157,55.8410243035325));
#170317=CARTESIAN_POINT('Ctrl Pts',(82.5470843234707,1.62722091554012,55.8182696649173));
#170318=CARTESIAN_POINT('Ctrl Pts',(82.631757366863,0.811817315023689,55.7967190249472));
#170319=CARTESIAN_POINT('Ctrl Pts',(82.6484237067625,0.560224074816844,
55.7916328816616));
#170320=CARTESIAN_POINT('Ctrl Pts',(82.6574089882071,0.247521183882508,
55.7870555173154));
#170321=CARTESIAN_POINT('Ctrl Pts',(82.6586062479302,0.186777458460161,
55.7862477569346));
#170322=CARTESIAN_POINT('Ctrl Pts',(82.6595577826136,0.0977054394520253,
55.7851792375336));
#170323=CARTESIAN_POINT('Ctrl Pts',(82.6597411744399,0.0693838653862917,
55.7848566701605));
#170324=CARTESIAN_POINT('Ctrl Pts',(82.6598547850039,0.0192637541456681,
55.7843158126665));
#170325=CARTESIAN_POINT('Ctrl Pts',(82.6598335891773,-0.00253431925762405,
55.7840906022901));
#170326=CARTESIAN_POINT('Ctrl Pts',(82.6596340842985,-0.0499017624191425,
55.783622892004));
#170327=CARTESIAN_POINT('Ctrl Pts',(82.6594292367648,-0.0754707138692689,
55.7833841888325));
#170328=CARTESIAN_POINT('Ctrl Pts',(82.6585870595155,-0.146779261889534,
55.7827573272739));
#170329=CARTESIAN_POINT('Ctrl Pts',(82.6577360359873,-0.192515982101173,
55.7823998490237));
#170330=CARTESIAN_POINT('Ctrl Pts',(82.6509775435299,-0.458580943742663,
55.7805850650758));
#170331=CARTESIAN_POINT('Ctrl Pts',(82.638172332812,-0.678681116301826,
55.7801415042764));
#170332=CARTESIAN_POINT('Ctrl Pts',(82.5707444230845,-1.41962827553383,
55.7825446168574));
#170333=CARTESIAN_POINT('Ctrl Pts',(82.4829396886288,-1.93657489927633,
55.7907945584611));
#170334=CARTESIAN_POINT('Ctrl Pts',(82.2602112022678,-2.82560554272926,
55.8181788564529));
#170335=CARTESIAN_POINT('Ctrl Pts',(82.1426446438464,-3.20094752095467,
55.8340593003786));
#170336=CARTESIAN_POINT('Ctrl Pts',(81.974866658571,-3.64452544456632,55.858297746295));
#170337=CARTESIAN_POINT('Ctrl Pts',(81.9451355384252,-3.72035487614268,
55.8626396257654));
#170338=CARTESIAN_POINT('Ctrl Pts',(81.8966646676697,-3.83972519316476,
55.8697899598124));
#170339=CARTESIAN_POINT('Ctrl Pts',(81.8785254264841,-3.88351296676275,
55.8724807253108));
#170340=CARTESIAN_POINT('Ctrl Pts',(81.8438169628446,-3.9656628343147,55.8776568236605));
#170341=CARTESIAN_POINT('Ctrl Pts',(81.8273160220162,-4.0040535019679,55.8801287796844));
#170342=CARTESIAN_POINT('Ctrl Pts',(81.7895669762948,-4.09040186860476,
55.8858085047255));
#170343=CARTESIAN_POINT('Ctrl Pts',(81.7681834501694,-4.13829725373535,
55.8890428598873));
#170344=CARTESIAN_POINT('Ctrl Pts',(81.7023829678875,-4.28265291114649,
55.8990453721285));
#170345=CARTESIAN_POINT('Ctrl Pts',(81.6568245220118,-4.3785688757584,55.9060373910911));
#170346=CARTESIAN_POINT('Ctrl Pts',(81.3835434119711,-4.93127178930689,
55.9483376159127));
#170347=CARTESIAN_POINT('Ctrl Pts',(81.1231888358869,-5.37057415499867,
55.9900688843047));
#170348=CARTESIAN_POINT('Ctrl Pts',(80.7292983129638,-5.93276455048374,
56.0539816715363));
#170349=CARTESIAN_POINT('Ctrl Pts',(80.6239193981101,-6.07498988223039,
56.0711371189249));
#170350=CARTESIAN_POINT('Ctrl Pts',(80.3320179476734,-6.44782483159188,
56.1186854656449));
#170351=CARTESIAN_POINT('Ctrl Pts',(80.1389714699411,-6.67295649371278,
56.1501612972022));
#170352=CARTESIAN_POINT('Ctrl Pts',(79.9024408413115,-6.92504963604771,
56.1884673012694));
#170353=CARTESIAN_POINT('Ctrl Pts',(79.8683631238069,-6.96083022844835,
56.193980166324));
#170354=CARTESIAN_POINT('Ctrl Pts',(79.8151198219738,-7.01590419345922,
56.2025822919177));
#170355=CARTESIAN_POINT('Ctrl Pts',(79.7961378948207,-7.0353778390989,56.2056468850472));
#170356=CARTESIAN_POINT('Ctrl Pts',(79.7605820696068,-7.0715557042717,56.2113828529844));
#170357=CARTESIAN_POINT('Ctrl Pts',(79.744028267514,-7.08827955947311,56.2140515415401));
#170358=CARTESIAN_POINT('Ctrl Pts',(79.7056187609149,-7.12680824350938,
56.2202396132705));
#170359=CARTESIAN_POINT('Ctrl Pts',(79.6837208962468,-7.14856973018169,
56.2237645656928));
#170360=CARTESIAN_POINT('Ctrl Pts',(79.6119304288914,-7.21924953091756,
56.235312178609));
#170361=CARTESIAN_POINT('Ctrl Pts',(79.5616265976128,-7.26773812871635,
56.2433900861627));
#170362=CARTESIAN_POINT('Ctrl Pts',(79.2355482633924,-7.57546565443415,
56.2956877548929));
#170363=CARTESIAN_POINT('Ctrl Pts',(78.9457912405974,-7.81910045546643,
56.3418781368217));
#170364=CARTESIAN_POINT('Ctrl Pts',(78.3672991887962,-8.25151230180316,
56.4344443943366));
#170365=CARTESIAN_POINT('Ctrl Pts',(78.0811664485325,-8.44295338347043,
56.4803742384066));
#170366=CARTESIAN_POINT('Ctrl Pts',(77.5457400236712,-8.76202861299789,
56.5669744605854));
#170367=CARTESIAN_POINT('Ctrl Pts',(77.2997999197313,-8.89475760749457,
56.6069819412294));
#170368=CARTESIAN_POINT('Ctrl Pts',(76.9825100957221,-9.04893325464078,
56.6589472236596));
#170369=CARTESIAN_POINT('Ctrl Pts',(76.9159770924969,-9.08034395136983,
56.669862493727));
#170370=CARTESIAN_POINT('Ctrl Pts',(76.8078320754716,-9.12992211309388,
56.687634927693));
#170371=CARTESIAN_POINT('Ctrl Pts',(76.7664296728167,-9.14855628087697,
56.694446068824));
#170372=CARTESIAN_POINT('Ctrl Pts',(76.6867387936664,-9.18376037520967,
56.7075697147214));
#170373=CARTESIAN_POINT('Ctrl Pts',(76.648470388933,-9.20037492912495,56.7138778127472));
#170374=CARTESIAN_POINT('Ctrl Pts',(76.560570212029,-9.23787310215429,56.7283807479796));
#170375=CARTESIAN_POINT('Ctrl Pts',(76.5108722087848,-9.25859223283021,
56.73659046701));
#170376=CARTESIAN_POINT('Ctrl Pts',(76.3774642447571,-9.31292474763031,
56.7586544405836));
#170377=CARTESIAN_POINT('Ctrl Pts',(76.2934661056771,-9.34578995117681,
56.7725739189794));
#170378=CARTESIAN_POINT('Ctrl Pts',(75.5598594453791,-9.62120188052528,
56.8943670593408));
#170379=CARTESIAN_POINT('Ctrl Pts',(74.8874651900091,-9.7949782855156,57.0077064878314));
#170380=CARTESIAN_POINT('Ctrl Pts',(73.8159504270238,-9.95296389788093,
57.1881339633459));
#170381=CARTESIAN_POINT('Ctrl Pts',(73.4262027288345,-9.98662173994688,
57.2536810591757));
#170382=CARTESIAN_POINT('Ctrl Pts',(72.9864642559843,-9.99800712030206,
57.3268856743326));
#170383=CARTESIAN_POINT('Ctrl Pts',(72.9375097698522,-9.99890495110155,
57.335024665605));
#170384=CARTESIAN_POINT('Ctrl Pts',(72.8627839308599,-9.99971136128126,
57.3474301279833));
#170385=CARTESIAN_POINT('Ctrl Pts',(72.8370175548178,-9.99988708951038,
57.3517043836381));
#170386=CARTESIAN_POINT('Ctrl Pts',(72.7897945616622,-10.0000216248123,
57.3595315739047));
#170387=CARTESIAN_POINT('Ctrl Pts',(72.768338554275,-10.0000118088889,57.3630854475909));
#170388=CARTESIAN_POINT('Ctrl Pts',(72.7196523502409,-9.9998285654065,57.3711440875481));
#170389=CARTESIAN_POINT('Ctrl Pts',(72.6924223931206,-9.99961182395552,
57.3756473663842));
#170390=CARTESIAN_POINT('Ctrl Pts',(72.6214924366245,-9.99874962547304,
57.387368176853));
#170391=CARTESIAN_POINT('Ctrl Pts',(72.5777942269155,-9.99792415229429,
57.3945796331145));
#170392=CARTESIAN_POINT('Ctrl Pts',(72.2467762095126,-9.9894414168373,57.4491420010951));
#170393=CARTESIAN_POINT('Ctrl Pts',(71.9598441461565,-9.9693595767181,57.4960695289819));
#170394=CARTESIAN_POINT('Ctrl Pts',(71.6635196628818,-9.93539699957304,
57.5443796562413));
#170395=CARTESIAN_POINT('Ctrl Pts',(71.6528759737561,-9.93415931643981,
57.5461146976422));
#170396=CARTESIAN_POINT('Ctrl Pts',(71.2098765387747,-9.88190558132804,
57.6183202116018));
#170397=CARTESIAN_POINT('Ctrl Pts',(70.7812687173686,-9.80198862539112,
57.6878730205509));
#170398=CARTESIAN_POINT('Ctrl Pts',(69.9866093302135,-9.59800776372879,
57.8172338909326));
#170399=CARTESIAN_POINT('Ctrl Pts',(69.6197771053583,-9.4803630262814,57.8771180451826));
#170400=CARTESIAN_POINT('Ctrl Pts',(69.1856772115836,-9.31229090273862,
57.9483614319441));
#170401=CARTESIAN_POINT('Ctrl Pts',(69.1110067137023,-9.28231600601225,
57.9606293486214));
#170402=CARTESIAN_POINT('Ctrl Pts',(68.9934052907492,-9.23341455738645,
57.979971641371));
#170403=CARTESIAN_POINT('Ctrl Pts',(68.9502305585652,-9.21509638594357,
57.9870772703113));
#170404=CARTESIAN_POINT('Ctrl Pts',(68.8691976078222,-9.18002637846326,
58.0004220169187));
#170405=CARTESIAN_POINT('Ctrl Pts',(68.83131124957,-9.16334356079774,58.0066647701045));
#170406=CARTESIAN_POINT('Ctrl Pts',(68.7460528387754,-9.1251536564957,58.0207210911115));
#170407=CARTESIAN_POINT('Ctrl Pts',(68.6987429589574,-9.10350782765388,
58.028526418776));
#170408=CARTESIAN_POINT('Ctrl Pts',(68.5559936329689,-9.03681485324046,
58.0520936745828));
#170409=CARTESIAN_POINT('Ctrl Pts',(68.4610977555133,-8.99059696045416,
58.0677824928345));
#170410=CARTESIAN_POINT('Ctrl Pts',(67.9212161944057,-8.7167801821928,58.1571511796786));
#170411=CARTESIAN_POINT('Ctrl Pts',(67.4931056969342,-8.45680223914048,
58.2285056107748));
#170412=CARTESIAN_POINT('Ctrl Pts',(66.9384837795892,-8.05928162019742,
58.3207656067462));
#170413=CARTESIAN_POINT('Ctrl Pts',(66.7936749935322,-7.94931667603692,
58.3448302420551));
#170414=CARTESIAN_POINT('Ctrl Pts',(66.4212284288528,-7.64995766362703,
58.4065325495347));
#170415=CARTESIAN_POINT('Ctrl Pts',(66.1988104994536,-7.45416468378645,
58.4431848207273));
#170416=CARTESIAN_POINT('Ctrl Pts',(65.9497103543362,-7.2143324758635,58.483703747417));
#170417=CARTESIAN_POINT('Ctrl Pts',(65.9143811001581,-7.17980817286902,
58.4894371950452));
#170418=CARTESIAN_POINT('Ctrl Pts',(65.8600004773793,-7.12587140748161,
58.4982397389804));
#170419=CARTESIAN_POINT('Ctrl Pts',(65.840772802175,-7.10664419298143,58.5013476431137));
#170420=CARTESIAN_POINT('Ctrl Pts',(65.8050520235847,-7.07063130034372,
58.5071126807602));
#170421=CARTESIAN_POINT('Ctrl Pts',(65.7885397150802,-7.05386589427028,
58.5097740585185));
#170422=CARTESIAN_POINT('Ctrl Pts',(65.7504990403371,-7.01496819926987,
58.5158971397634));
#170423=CARTESIAN_POINT('Ctrl Pts',(65.7290130184311,-6.9927934443895,58.5193495129907));
#170424=CARTESIAN_POINT('Ctrl Pts',(65.659232842176,-6.92010530581626,58.5305429206518));
#170425=CARTESIAN_POINT('Ctrl Pts',(65.6113586508592,-6.86917761357063,
58.5381926513893));
#170426=CARTESIAN_POINT('Ctrl Pts',(65.3100123645777,-6.54179691289175,
58.5861739248146));
#170427=CARTESIAN_POINT('Ctrl Pts',(65.0715038219831,-6.25152202094488,
58.6233820631894));
#170428=CARTESIAN_POINT('Ctrl Pts',(64.6031266231701,-5.611218264681,58.6956468107223));
#170429=CARTESIAN_POINT('Ctrl Pts',(64.3776621958961,-5.25876457416573,
58.7299350072359));
#170430=CARTESIAN_POINT('Ctrl Pts',(64.1022822245504,-4.76250883216498,
58.7715743728875));
#170431=CARTESIAN_POINT('Ctrl Pts',(64.0327518383694,-4.6303510035834,58.7820603105359));
#170432=CARTESIAN_POINT('Ctrl Pts',(63.9164034921777,-4.39671328034927,
58.7995708322651));
#170433=CARTESIAN_POINT('Ctrl Pts',(63.8682899648765,-4.29592408523252,
58.8067998110784));
#170434=CARTESIAN_POINT('Ctrl Pts',(63.7996201879395,-4.14568765497114,
58.8171011345529));
#170435=CARTESIAN_POINT('Ctrl Pts',(63.7777692979185,-4.09685583444628,
58.8203764152899));
#170436=CARTESIAN_POINT('Ctrl Pts',(63.7395034391521,-4.00947809550287,
58.8261075068487));
#170437=CARTESIAN_POINT('Ctrl Pts',(63.7229383537878,-3.97100088051133,
58.8285868303989));
#170438=CARTESIAN_POINT('Ctrl Pts',(63.6883939566803,-3.88936227511663,
58.8337536198343));
#170439=CARTESIAN_POINT('Ctrl Pts',(63.6704739346249,-3.84617630472271,
58.8364318033698));
#170440=CARTESIAN_POINT('Ctrl Pts',(63.6232827182517,-3.73017334220863,
58.8434787435992));
#170441=CARTESIAN_POINT('Ctrl Pts',(63.5945589276684,-3.6571320789314,58.8477617194265));
#170442=CARTESIAN_POINT('Ctrl Pts',(63.4609496468839,-3.30536745325955,
58.8676504444353));
#170443=CARTESIAN_POINT('Ctrl Pts',(63.3675671683697,-3.02233787327736,
58.8814528823321));
#170444=CARTESIAN_POINT('Ctrl Pts',(63.1327154912277,-2.18824256650017,
58.9156148795403));
#170445=CARTESIAN_POINT('Ctrl Pts',(63.0250208122757,-1.62869950712594,
58.9305342332453));
#170446=CARTESIAN_POINT('Ctrl Pts',(62.9379234590289,-0.812159226565499,
58.9392625583131));
#170447=CARTESIAN_POINT('Ctrl Pts',(62.9205065379399,-0.5604315408587,58.9401852381982));
#170448=CARTESIAN_POINT('Ctrl Pts',(62.9104905284351,-0.247577749753939,
58.9389569323095));
#170449=CARTESIAN_POINT('Ctrl Pts',(62.9090885448431,-0.186818084566122,
58.93860734116));
#170450=CARTESIAN_POINT('Ctrl Pts',(62.9078284563691,-0.0977271282440349,
58.937928606089));
#170451=CARTESIAN_POINT('Ctrl Pts',(62.9075457140133,-0.0694025620102268,
58.9376882019774));
#170452=CARTESIAN_POINT('Ctrl Pts',(62.9073010701311,-0.0273849857570098,
58.9372947144178));
#170453=CARTESIAN_POINT('Ctrl Pts',(62.9072488797159,-0.0136925086044199,
58.9371606796013));
#170454=CARTESIAN_POINT('Ctrl Pts',(62.9072242170052,5.40442818497922E-11,
58.9370208104186));
#170455=CARTESIAN_POINT('Ctrl Pts',(62.9025030071408,2.40572005160039E-14,
58.910245498748));
#170456=CARTESIAN_POINT('Ctrl Pts',(62.9025342912689,-0.0173686582679938,
58.9104229198545));
#170457=CARTESIAN_POINT('Ctrl Pts',(62.9026103556841,-0.0347272718981202,
58.9105939150937));
#170458=CARTESIAN_POINT('Ctrl Pts',(62.9028777641638,-0.0731358798131149,
58.9109581633259));
#170459=CARTESIAN_POINT('Ctrl Pts',(62.9030900274107,-0.0941756765552429,
58.9111483321575));
#170460=CARTESIAN_POINT('Ctrl Pts',(62.9040397921087,-0.166048601348156,
58.9117656646191));
#170461=CARTESIAN_POINT('Ctrl Pts',(62.9050954046548,-0.216877140292341,
58.9121470526904));
#170462=CARTESIAN_POINT('Ctrl Pts',(62.9143026604179,-0.5419980837562,58.9142254053892));
#170463=CARTESIAN_POINT('Ctrl Pts',(62.9332410441641,-0.815880099105862,
58.9143284989985));
#170464=CARTESIAN_POINT('Ctrl Pts',(63.014969794944,-1.55827244014797,58.9096275643017));
#170465=CARTESIAN_POINT('Ctrl Pts',(63.09943809618,-2.02366545558728,58.9012098442081));
#170466=CARTESIAN_POINT('Ctrl Pts',(63.3100048167335,-2.85092599920466,
58.8751221496162));
#170467=CARTESIAN_POINT('Ctrl Pts',(63.4247916158072,-3.21480069270942,
58.8595719467266));
#170468=CARTESIAN_POINT('Ctrl Pts',(63.5883534277162,-3.64684082200208,
58.8359360258491));
#170469=CARTESIAN_POINT('Ctrl Pts',(63.6179001438503,-3.72215160646429,
58.8316202608708));
#170470=CARTESIAN_POINT('Ctrl Pts',(63.6661357363112,-3.84089593402397,
58.824503850265));
#170471=CARTESIAN_POINT('Ctrl Pts',(63.6842348233695,-3.8845720558084,58.8218187935395));
#170472=CARTESIAN_POINT('Ctrl Pts',(63.7189119915818,-3.96662458840719,
58.81664697183));
#170473=CARTESIAN_POINT('Ctrl Pts',(63.7354235084024,-4.00502883876494,
58.8141732468591));
#170474=CARTESIAN_POINT('Ctrl Pts',(63.7732617179863,-4.09155602479526,
58.8084796869005));
#170475=CARTESIAN_POINT('Ctrl Pts',(63.7947262317453,-4.13961553848542,
58.8052327949778));
#170476=CARTESIAN_POINT('Ctrl Pts',(63.8610200350821,-4.28499147354866,
58.7951542700602));
#170477=CARTESIAN_POINT('Ctrl Pts',(63.9070152812988,-4.38175165236982,
58.7880939786866));
#170478=CARTESIAN_POINT('Ctrl Pts',(64.1692392423258,-4.91150078674183,
58.7474959071995));
#170479=CARTESIAN_POINT('Ctrl Pts',(64.4146406270562,-5.32887623782263,
58.7082214426276));
#170480=CARTESIAN_POINT('Ctrl Pts',(64.8018013773615,-5.89030287614121,
58.6454642095547));
#170481=CARTESIAN_POINT('Ctrl Pts',(64.9195192906061,-6.05057757157698,
58.6263030524046));
#170482=CARTESIAN_POINT('Ctrl Pts',(65.2262870571687,-6.44313245235599,
58.5763340352565));
#170483=CARTESIAN_POINT('Ctrl Pts',(65.4210945266854,-6.67053695085696,
58.5445688959729));
#170484=CARTESIAN_POINT('Ctrl Pts',(65.6596317011368,-6.92479128899727,
58.5059376810256));
#170485=CARTESIAN_POINT('Ctrl Pts',(65.6937665975725,-6.96063418930786,
58.5004155368764));
#170486=CARTESIAN_POINT('Ctrl Pts',(65.747080158213,-7.01578291223961,58.4918020319176));
#170487=CARTESIAN_POINT('Ctrl Pts',(65.7660743654856,-7.03526978587571,
58.4887354471778));
#170488=CARTESIAN_POINT('Ctrl Pts',(65.8016399989601,-7.07145860285653,
58.4829978824889));
#170489=CARTESIAN_POINT('Ctrl Pts',(65.8181912067245,-7.08818030322966,
58.4803296049725));
#170490=CARTESIAN_POINT('Ctrl Pts',(65.8565776532105,-7.12668696804056,
58.4741452322619));
#170491=CARTESIAN_POINT('Ctrl Pts',(65.8784548819281,-7.1484287631162,58.4706235902747));
#170492=CARTESIAN_POINT('Ctrl Pts',(65.95010784568,-7.21897644402316,58.4590980524618));
#170493=CARTESIAN_POINT('Ctrl Pts',(66.0002926365253,-7.26735490810976,
58.4510392041551));
#170494=CARTESIAN_POINT('Ctrl Pts',(66.3264422016386,-7.5751941552042,58.3987296727815));
#170495=CARTESIAN_POINT('Ctrl Pts',(66.6164150449733,-7.81902438452433,
58.3525050495425));
#170496=CARTESIAN_POINT('Ctrl Pts',(67.2394907643446,-8.28474647656219,
58.2528047338209));
#170497=CARTESIAN_POINT('Ctrl Pts',(67.5735397682636,-8.5041999340286,58.1991521789296));
#170498=CARTESIAN_POINT('Ctrl Pts',(68.0540499006501,-8.77970114605355,
58.121252280052));
#170499=CARTESIAN_POINT('Ctrl Pts',(68.1901935791239,-8.85354907957623,
58.0991073914919));
#170500=CARTESIAN_POINT('Ctrl Pts',(68.4298920273864,-8.97633916261201,
58.0599758389674));
#170501=CARTESIAN_POINT('Ctrl Pts',(68.5326856563159,-9.02675085809725,
58.0431502382624));
#170502=CARTESIAN_POINT('Ctrl Pts',(68.6849427005484,-9.09814817447399,
58.0181611935353));
#170503=CARTESIAN_POINT('Ctrl Pts',(68.7337542152503,-9.12055066262303,
58.0101400960207));
#170504=CARTESIAN_POINT('Ctrl Pts',(68.8206739087486,-9.15958321890219,
57.9958390581626));
#170505=CARTESIAN_POINT('Ctrl Pts',(68.8587107372246,-9.17637463661734,
57.9895748390962));
#170506=CARTESIAN_POINT('Ctrl Pts',(68.9389814253069,-9.21120246816204,
57.9763427089367));
#170507=CARTESIAN_POINT('Ctrl Pts',(68.9812368555633,-9.22918479117664,
57.9693699374593));
#170508=CARTESIAN_POINT('Ctrl Pts',(69.0937049371064,-9.2761169259097,57.9507920647203));
#170509=CARTESIAN_POINT('Ctrl Pts',(69.1641236765312,-9.30454619076747,
57.939140528811));
#170510=CARTESIAN_POINT('Ctrl Pts',(69.4862920862339,-9.4302768968974,57.8857481274107));
#170511=CARTESIAN_POINT('Ctrl Pts',(69.7415477202365,-9.51792282889497,
57.843202957748));
#170512=CARTESIAN_POINT('Ctrl Pts',(70.5578155419666,-9.76094538690896,
57.7065771209657));
#170513=CARTESIAN_POINT('Ctrl Pts',(71.128860984443,-9.87668951302964,57.6100967183394));
#170514=CARTESIAN_POINT('Ctrl Pts',(71.960673633025,-9.96891279633525,57.4702511870423));
#170515=CARTESIAN_POINT('Ctrl Pts',(72.2156418465909,-9.98705241367056,
57.4274908907429));
#170516=CARTESIAN_POINT('Ctrl Pts',(72.5317680219692,-9.99705410672111,
57.3748134266249));
#170517=CARTESIAN_POINT('Ctrl Pts',(72.5924940441712,-9.9984063538746,57.3647099715857));
#170518=CARTESIAN_POINT('Ctrl Pts',(72.6813205044352,-9.99955242324994,
57.3499576255916));
#170519=CARTESIAN_POINT('Ctrl Pts',(72.7094116097431,-9.99979322436574,
57.3452961000567));
#170520=CARTESIAN_POINT('Ctrl Pts',(72.7588299662828,-10.0000028811811,
57.3371026915096));
#170521=CARTESIAN_POINT('Ctrl Pts',(72.7801564671796,-10.0000232682167,
57.3335692093946));
#170522=CARTESIAN_POINT('Ctrl Pts',(72.8265282793482,-9.99991520040572,
57.3258913849486));
#170523=CARTESIAN_POINT('Ctrl Pts',(72.8515733429144,-9.99976017905586,
57.3217479627198));
#170524=CARTESIAN_POINT('Ctrl Pts',(72.9209407289911,-9.99906311135047,
57.3102806329203));
#170525=CARTESIAN_POINT('Ctrl Pts',(72.9652615313968,-9.99831501398692,
57.3029636869536));
#170526=CARTESIAN_POINT('Ctrl Pts',(73.2120407645548,-9.99246377887463,
57.2622726676503));
#170527=CARTESIAN_POINT('Ctrl Pts',(73.4143411697187,-9.98134760084399,
57.2291019584791));
#170528=CARTESIAN_POINT('Ctrl Pts',(74.1590739731057,-9.91708696058708,
57.1073832542155));
#170529=CARTESIAN_POINT('Ctrl Pts',(74.6973353667004,-9.82477421979976,
57.0201282859161));
#170530=CARTESIAN_POINT('Ctrl Pts',(75.5909101085944,-9.5931600653227,56.8746506189172));
#170531=CARTESIAN_POINT('Ctrl Pts',(75.9508635486133,-9.47721678910531,
56.8158822677019));
#170532=CARTESIAN_POINT('Ctrl Pts',(76.3780410405796,-9.31173238424783,
56.7457738262313));
#170533=CARTESIAN_POINT('Ctrl Pts',(76.4523980563466,-9.28187149455451,
56.7335572648992));
#170534=CARTESIAN_POINT('Ctrl Pts',(76.5696211207097,-9.23311556292462,
56.7142770553058));
#170535=CARTESIAN_POINT('Ctrl Pts',(76.6127283574853,-9.21482221852788,
56.7071824875156));
#170536=CARTESIAN_POINT('Ctrl Pts',(76.6937025395623,-9.17977150395332,
56.6938473437002));
#170537=CARTESIAN_POINT('Ctrl Pts',(76.73159717781,-9.1630820797026,56.687603190084));
#170538=CARTESIAN_POINT('Ctrl Pts',(76.816964030267,-9.12483673414464,56.6735289078984));
#170539=CARTESIAN_POINT('Ctrl Pts',(76.8643733963188,-9.10314056843571,
56.6657071093106));
#170540=CARTESIAN_POINT('Ctrl Pts',(77.0077414827794,-9.03614085080102,
56.6420374941345));
#170541=CARTESIAN_POINT('Ctrl Pts',(77.1031493495533,-8.98965120953712,
56.6262637751262));
#170542=CARTESIAN_POINT('Ctrl Pts',(77.5995124876066,-8.73773245868233,
56.5440970859348));
#170543=CARTESIAN_POINT('Ctrl Pts',(77.9869522615415,-8.50627838538123,
56.4795728407288));
#170544=CARTESIAN_POINT('Ctrl Pts',(78.7331529385745,-7.98789563464108,
56.3553938402558));
#170545=CARTESIAN_POINT('Ctrl Pts',(79.0905424923617,-7.70087001339288,
56.2959741793573));
#170546=CARTESIAN_POINT('Ctrl Pts',(79.497765681327,-7.3247033024308,56.2293483485337));
#170547=CARTESIAN_POINT('Ctrl Pts',(79.5673634584594,-7.25852205814219,
56.2180040886079));
#170548=CARTESIAN_POINT('Ctrl Pts',(79.661262058269,-7.16661355164451,56.2027705859959));
#170549=CARTESIAN_POINT('Ctrl Pts',(79.6863834015439,-7.14176196039425,
56.1987022587048));
#170550=CARTESIAN_POINT('Ctrl Pts',(79.7284587820362,-7.09969401349658,
56.1919012511977));
#170551=CARTESIAN_POINT('Ctrl Pts',(79.745482044774,-7.08254977254455,56.1891532579657));
#170552=CARTESIAN_POINT('Ctrl Pts',(79.7803160489608,-7.04721272956597,
56.1835379142265));
#170553=CARTESIAN_POINT('Ctrl Pts',(79.7981198422834,-7.02901321619789,
56.1806720728125));
#170554=CARTESIAN_POINT('Ctrl Pts',(79.8447223321716,-6.98100920131469,
56.1731811584525));
#170555=CARTESIAN_POINT('Ctrl Pts',(79.8734074602198,-6.95109124997033,
56.1685810166465));
#170556=CARTESIAN_POINT('Ctrl Pts',(79.9950222400842,-6.82265977258022,
56.1491210942092));
#170557=CARTESIAN_POINT('Ctrl Pts',(80.0861598640805,-6.72241096163732,
56.1346461392179));
#170558=CARTESIAN_POINT('Ctrl Pts',(80.2544239170646,-6.52959413168857,
56.108086301528));
#170559=CARTESIAN_POINT('Ctrl Pts',(80.3319657344929,-6.4374320396065,56.0959170707031));
#170560=CARTESIAN_POINT('Ctrl Pts',(80.6939541038447,-5.99107850162928,
56.0393791190158));
#170561=CARTESIAN_POINT('Ctrl Pts',(80.9559994147831,-5.61888201167553,
55.9992509737802));
#170562=CARTESIAN_POINT('Ctrl Pts',(81.3664075105566,-4.94253295842123,
55.9368895665563));
#170563=CARTESIAN_POINT('Ctrl Pts',(81.5263213812908,-4.64644750119736,
55.9127664942475));
#170564=CARTESIAN_POINT('Ctrl Pts',(81.7046442838395,-4.2725370286962,55.8859732357997));
#170565=CARTESIAN_POINT('Ctrl Pts',(81.7373219096174,-4.20192092644069,
55.8810690142608));
#170566=CARTESIAN_POINT('Ctrl Pts',(81.7882576277528,-4.08841272845341,
55.8734332952313));
#170567=CARTESIAN_POINT('Ctrl Pts',(81.8070405218673,-4.04576526252089,
55.8706195698855));
#170568=CARTESIAN_POINT('Ctrl Pts',(81.842157498107,-3.96450525574626,55.8653627814097));
#170569=CARTESIAN_POINT('Ctrl Pts',(81.858547666924,-3.92591861480768,55.8629109327281));
#170570=CARTESIAN_POINT('Ctrl Pts',(81.895408490312,-3.83761013362202,55.8574007039593));
#170571=CARTESIAN_POINT('Ctrl Pts',(81.9157233945547,-3.7878231849306,55.854366716022));
#170572=CARTESIAN_POINT('Ctrl Pts',(81.9774692159133,-3.63296552248592,
55.8451544209256));
#170573=CARTESIAN_POINT('Ctrl Pts',(82.0175368826061,-3.52734839105768,
55.8391898560533));
#170574=CARTESIAN_POINT('Ctrl Pts',(82.24592031167,-2.89341059449705,55.8052889603103));
#170575=CARTESIAN_POINT('Ctrl Pts',(82.3917567001461,-2.35051118530748,
55.7839872145028));
#170576=CARTESIAN_POINT('Ctrl Pts',(82.525349966207,-1.613847614769,55.7661776652224));
#170577=CARTESIAN_POINT('Ctrl Pts',(82.5536618620599,-1.42865788028523,
55.7626177888971));
#170578=CARTESIAN_POINT('Ctrl Pts',(82.6179492638532,-0.913142139990253,
55.7553792079458));
#170579=CARTESIAN_POINT('Ctrl Pts',(82.6428772281945,-0.581656744058186,
55.7537386626833));
#170580=CARTESIAN_POINT('Ctrl Pts',(82.6528669907766,-0.201084493584069,
55.7556829203826));
#170581=CARTESIAN_POINT('Ctrl Pts',(82.6537938996066,-0.152604633247536,
55.7560017346494));
#170582=CARTESIAN_POINT('Ctrl Pts',(82.6546859107789,-0.0782442591020743,
55.7566016435419));
#170583=CARTESIAN_POINT('Ctrl Pts',(82.6548979563943,-0.0523670315677803,
55.7568310053257));
#170584=CARTESIAN_POINT('Ctrl Pts',(82.6551073110461,-0.0047241958240891,
55.7572915357648));
#170585=CARTESIAN_POINT('Ctrl Pts',(82.6551333942184,0.0170409902828053,
55.7575166520411));
#170586=CARTESIAN_POINT('Ctrl Pts',(82.6550341790086,0.0667067804927853,
55.758063890045));
#170587=CARTESIAN_POINT('Ctrl Pts',(82.6548641264406,0.0946068915860172,
55.7583954297706));
#170588=CARTESIAN_POINT('Ctrl Pts',(82.6541178920338,0.167809949977412,
55.7593280552602));
#170589=CARTESIAN_POINT('Ctrl Pts',(82.6533545310646,0.213109855960252,
55.7599682495316));
#170590=CARTESIAN_POINT('Ctrl Pts',(82.6442066695507,0.602154718065384,
55.7660004390248));
#170591=CARTESIAN_POINT('Ctrl Pts',(82.6187540126702,0.945218316972891,
55.7748949510362));
#170592=CARTESIAN_POINT('Ctrl Pts',(82.5265690674369,1.68002181989931,55.8009209666152));
#170593=CARTESIAN_POINT('Ctrl Pts',(82.4541356262684,2.07043194606314,55.8190848664116));
#170594=CARTESIAN_POINT('Ctrl Pts',(82.2656140061652,2.8331892824714,55.8625205332722));
#170595=CARTESIAN_POINT('Ctrl Pts',(82.1505203141465,3.20508695669689,55.8876162658754));
#170596=CARTESIAN_POINT('Ctrl Pts',(81.9858209027212,3.64520415645675,55.9219602953549));
#170597=CARTESIAN_POINT('Ctrl Pts',(81.9564512836613,3.72088125281246,55.9280375905523));
#170598=CARTESIAN_POINT('Ctrl Pts',(81.9085263432233,3.84006772535572,55.9378822178392));
#170599=CARTESIAN_POINT('Ctrl Pts',(81.8905723899394,3.8838227207945,55.9415552537532));
#170600=CARTESIAN_POINT('Ctrl Pts',(81.8561958915566,3.96594390355726,55.9485603325315));
#170601=CARTESIAN_POINT('Ctrl Pts',(81.8398415787454,4.00433844950523,55.951881671172));
#170602=CARTESIAN_POINT('Ctrl Pts',(81.8024007654925,4.09073877751059,55.9594604951477));
#170603=CARTESIAN_POINT('Ctrl Pts',(81.7811772146922,4.13868192326703,55.9637394245656));
#170604=CARTESIAN_POINT('Ctrl Pts',(81.7157816854263,4.28333403556716,55.9768734974031));
#170605=CARTESIAN_POINT('Ctrl Pts',(81.6704533624586,4.37949524045373,55.9859098094996));
#170606=CARTESIAN_POINT('Ctrl Pts',(81.392405257031,4.94582714483263,56.0409680083436));
#170607=CARTESIAN_POINT('Ctrl Pts',(81.1247994764948,5.39740610865565,56.0924276399303));
#170608=CARTESIAN_POINT('Ctrl Pts',(80.6404665156884,6.08525149804973,56.1846295327195));
#170609=CARTESIAN_POINT('Ctrl Pts',(80.4453478688704,6.33600141878482,56.2215985093296));
#170610=CARTESIAN_POINT('Ctrl Pts',(80.1714611855094,6.65529223623627,56.2736431613594));
#170611=CARTESIAN_POINT('Ctrl Pts',(80.102938218998,6.73270132713967,56.2866761225027));
#170612=CARTESIAN_POINT('Ctrl Pts',(79.9843873274947,6.862496079063,56.3092635089353));
#170613=CARTESIAN_POINT('Ctrl Pts',(79.934958889108,6.91543947332063,56.3186922082157));
#170614=CARTESIAN_POINT('Ctrl Pts',(79.863145954515,6.99069466959353,56.3324124766871));
#170615=CARTESIAN_POINT('Ctrl Pts',(79.8412172630735,7.01345618253948,56.3366049154377));
#170616=CARTESIAN_POINT('Ctrl Pts',(79.8027936208427,7.05296039309222,56.3439564659895));
#170617=CARTESIAN_POINT('Ctrl Pts',(79.7863461709483,7.06975082341103,56.3471050992447));
#170618=CARTESIAN_POINT('Ctrl Pts',(79.750903870796,7.10567641210136,56.353893973126));
#170619=CARTESIAN_POINT('Ctrl Pts',(79.7318908918214,7.12479239867154,56.3575382113221));
#170620=CARTESIAN_POINT('Ctrl Pts',(79.6793508285267,7.17718868482272,56.3676145299479));
#170621=CARTESIAN_POINT('Ctrl Pts',(79.645667040466,7.21030420375505,56.3740810894789));
#170622=CARTESIAN_POINT('Ctrl Pts',(79.4548278975932,7.39526226663255,56.4107488422979));
#170623=CARTESIAN_POINT('Ctrl Pts',(79.2930236368102,7.54202220522219,56.4419529715292));
#170624=CARTESIAN_POINT('Ctrl Pts',(78.7665629883177,7.98863151605013,56.5435304744943));
#170625=CARTESIAN_POINT('Ctrl Pts',(78.3855367794655,8.26741933616086,56.6170888762217));
#170626=CARTESIAN_POINT('Ctrl Pts',(77.7968388750445,8.63609731930965,56.7297712509923));
#170627=CARTESIAN_POINT('Ctrl Pts',(77.6034414638665,8.74816817762196,56.7666543607519));
#170628=CARTESIAN_POINT('Ctrl Pts',(77.2745049814969,8.92397698378391,56.8291011340283));
#170629=CARTESIAN_POINT('Ctrl Pts',(77.1409947007258,8.99143070836977,56.8543726086862));
#170630=CARTESIAN_POINT('Ctrl Pts',(76.952371607933,9.08133667158602,56.8899655143526));
#170631=CARTESIAN_POINT('Ctrl Pts',(76.8985005769538,9.10641111998939,56.9001185940377));
#170632=CARTESIAN_POINT('Ctrl Pts',(76.805823573605,9.14851946610285,56.9175642600107));
#170633=CARTESIAN_POINT('Ctrl Pts',(76.7671274819039,9.16579709438249,56.9248422123066));
#170634=CARTESIAN_POINT('Ctrl Pts',(76.6884239565763,9.20032273338006,56.9396320930603));
#170635=CARTESIAN_POINT('Ctrl Pts',(76.6484111517669,9.21755583147009,56.9471446752639));
#170636=CARTESIAN_POINT('Ctrl Pts',(76.5480441732338,9.25998543610024,56.9659727030585));
#170637=CARTESIAN_POINT('Ctrl Pts',(76.487551860372,9.2848416693542,56.9773058947809));
#170638=CARTESIAN_POINT('Ctrl Pts',(76.2623402264916,9.37473478142222,57.0194460009106));
#170639=CARTESIAN_POINT('Ctrl Pts',(76.0961338266892,9.43586305753576,57.0504400432094));
#170640=CARTESIAN_POINT('Ctrl Pts',(75.3537733601903,9.68606621061228,57.1884688740469));
#170641=CARTESIAN_POINT('Ctrl Pts',(74.7626083962399,9.8253428950092,57.2972227740556));
#170642=CARTESIAN_POINT('Ctrl Pts',(73.8202296514385,9.95589747587143,57.4709356885238));
#170643=CARTESIAN_POINT('Ctrl Pts',(73.4755939287353,9.98495018454923,57.534560246781));
#170644=CARTESIAN_POINT('Ctrl Pts',(73.0723052086547,9.99726578219294,57.6096063145284));
#170645=CARTESIAN_POINT('Ctrl Pts',(73.0143360141412,9.99851414849793,57.6204080133131));
#170646=CARTESIAN_POINT('Ctrl Pts',(72.928852687366,9.99958566903191,57.6363611368264));
#170647=CARTESIAN_POINT('Ctrl Pts',(72.9013423823041,9.99981302850819,57.6414989355973));
#170648=CARTESIAN_POINT('Ctrl Pts',(72.8524306804665,10.0000083972134,57.6506407332592));
#170649=CARTESIAN_POINT('Ctrl Pts',(72.831029474739,10.0000227845603,57.6546431420296));
#170650=CARTESIAN_POINT('Ctrl Pts',(72.7842542195342,9.99989883465852,57.663396355502));
#170651=CARTESIAN_POINT('Ctrl Pts',(72.7588807622356,9.99973164448181,57.6681480084801));
#170652=CARTESIAN_POINT('Ctrl Pts',(72.6874783543683,9.99897986318256,57.681528608682));
#170653=CARTESIAN_POINT('Ctrl Pts',(72.6414537367366,9.99816626338632,57.6901642078766));
#170654=CARTESIAN_POINT('Ctrl Pts',(72.3593295425278,9.99116158729582,57.7431586657038));
#170655=CARTESIAN_POINT('Ctrl Pts',(72.1235500244626,9.97664267091837,57.78770167283));
#170656=CARTESIAN_POINT('Ctrl Pts',(71.40840498152,9.90620628550892,57.9231933128778));
#170657=CARTESIAN_POINT('Ctrl Pts',(70.9324299634483,9.82299931367809,58.0138736950315));
#170658=CARTESIAN_POINT('Ctrl Pts',(70.1123819100195,9.61548347920324,58.1696493579154));
#170659=CARTESIAN_POINT('Ctrl Pts',(69.7655146378595,9.50665367784475,58.2353987178575));
#170660=CARTESIAN_POINT('Ctrl Pts',(69.3313178194179,9.34316708616744,58.3173486902701));
#170661=CARTESIAN_POINT('Ctrl Pts',(69.2378662466272,9.30631822157649,58.3349661940586));
#170662=CARTESIAN_POINT('Ctrl Pts',(69.0978815446895,9.2486020191161,58.3613244872542));
#170663=CARTESIAN_POINT('Ctrl Pts',(69.0509298242328,9.2288112867636,58.3701598043824));
#170664=CARTESIAN_POINT('Ctrl Pts',(68.9663066816261,9.19235730439304,58.3860743533869));
#170665=CARTESIAN_POINT('Ctrl Pts',(68.9285833913971,9.17582262596013,58.3931652134119));
#170666=CARTESIAN_POINT('Ctrl Pts',(68.8477058310117,9.1397601199923,58.4083603275334));
#170667=CARTESIAN_POINT('Ctrl Pts',(68.8045855847042,9.12015543506491,58.4164570663256));
#170668=CARTESIAN_POINT('Ctrl Pts',(68.6881339287258,9.06618364624091,58.4383111863728));
#170669=CARTESIAN_POINT('Ctrl Pts',(68.6150755822808,9.03121226622456,58.4520086564608));
#170670=CARTESIAN_POINT('Ctrl Pts',(68.1381466699981,8.7955792971828,58.5413464457309));
#170671=CARTESIAN_POINT('Ctrl Pts',(67.74771901752,8.56785444753638,58.6140683772073));
#170672=CARTESIAN_POINT('Ctrl Pts',(67.0970598350584,8.12548011414788,58.7352523955257));
#170673=CARTESIAN_POINT('Ctrl Pts',(66.829725500545,7.92301211440147,58.7850494681557));
#170674=CARTESIAN_POINT('Ctrl Pts',(66.3951885895302,7.55752403764773,58.8665169981539));
#170675=CARTESIAN_POINT('Ctrl Pts',(66.222574790196,7.40158626085029,58.8990365033695));
#170676=CARTESIAN_POINT('Ctrl Pts',(66.0219453491944,7.20700544304562,58.9371807612201));
#170677=CARTESIAN_POINT('Ctrl Pts',(65.988554097954,7.17415594591082,58.9435413493771));
#170678=CARTESIAN_POINT('Ctrl Pts',(65.9365678098929,7.12227888855382,58.9534649532022));
#170679=CARTESIAN_POINT('Ctrl Pts',(65.9178155000774,7.10341394175211,58.9570488906134));
#170680=CARTESIAN_POINT('Ctrl Pts',(65.8825753950237,7.06767407712765,58.9637925633479));
#170681=CARTESIAN_POINT('Ctrl Pts',(65.8660716930858,7.05081574958995,58.9669544065797));
#170682=CARTESIAN_POINT('Ctrl Pts',(65.8271370088832,7.01075796502635,58.97442210123));
#170683=CARTESIAN_POINT('Ctrl Pts',(65.8047584130837,6.98750667247541,58.9787209915102));
#170684=CARTESIAN_POINT('Ctrl Pts',(65.7298378535979,6.90889642073338,58.9931344948668));
#170685=CARTESIAN_POINT('Ctrl Pts',(65.6778174513365,6.85303114838828,59.0031780994776));
#170686=CARTESIAN_POINT('Ctrl Pts',(65.5518046664728,6.71452149583707,59.0275854351167));
#170687=CARTESIAN_POINT('Ctrl Pts',(65.478536450389,6.63121385909819,59.0418446087248));
#170688=CARTESIAN_POINT('Ctrl Pts',(65.1725478769838,6.27128075288447,59.1016355963843));
#170689=CARTESIAN_POINT('Ctrl Pts',(64.9534804948299,5.98306163370636,59.1450434458933));
#170690=CARTESIAN_POINT('Ctrl Pts',(64.489757352552,5.29864141497704,59.2375827581187));
#170691=CARTESIAN_POINT('Ctrl Pts',(64.2559932066147,4.89581537161776,59.2847227242312));
#170692=CARTESIAN_POINT('Ctrl Pts',(64.0036093063675,4.38178642825061,59.3358089667328));
#170693=CARTESIAN_POINT('Ctrl Pts',(63.9579943076422,4.28501715074904,59.3450533214539));
#170694=CARTESIAN_POINT('Ctrl Pts',(63.8922690722984,4.13962980658163,59.3583884288315));
#170695=CARTESIAN_POINT('Ctrl Pts',(63.8709927647128,4.09156852755386,59.3627077809818));
#170696=CARTESIAN_POINT('Ctrl Pts',(63.8334927967838,4.00503936356984,59.370325329739));
#170697=CARTESIAN_POINT('Ctrl Pts',(63.8171313041858,3.96663496362141,59.373650563344));
#170698=CARTESIAN_POINT('Ctrl Pts',(63.7827743929955,3.88458348448609,59.3806366773712));
#170699=CARTESIAN_POINT('Ctrl Pts',(63.7648455037303,3.84090854991692,59.3842845032402));
#170700=CARTESIAN_POINT('Ctrl Pts',(63.7170727132223,3.72217108621557,59.3940105529897));
#170701=CARTESIAN_POINT('Ctrl Pts',(63.687818382829,3.64686581329855,59.3999731772421));
#170702=CARTESIAN_POINT('Ctrl Pts',(63.5259603331888,3.21495033141412,59.4330063950098));
#170703=CARTESIAN_POINT('Ctrl Pts',(63.4125685846242,2.85119376599921,59.4563056449456));
#170704=CARTESIAN_POINT('Ctrl Pts',(63.180119070049,1.92462129514176,59.50500681965));
#170705=CARTESIAN_POINT('Ctrl Pts',(63.0878540298603,1.35626728101101,59.525342480917));
#170706=CARTESIAN_POINT('Ctrl Pts',(63.0303100530313,0.597995224837442,
59.5419459594712));
#170707=CARTESIAN_POINT('Ctrl Pts',(63.0213609437474,0.41265721398558,59.5451892306214));
#170708=CARTESIAN_POINT('Ctrl Pts',(63.0166172310532,0.18350400315967,59.5482719701468));
#170709=CARTESIAN_POINT('Ctrl Pts',(63.0159965172689,0.139834677949024,
59.5488179121082));
#170710=CARTESIAN_POINT('Ctrl Pts',(63.0154652684897,0.0710627943937142,
59.5496136497237));
#170711=CARTESIAN_POINT('Ctrl Pts',(63.0153649747804,0.0459625763126578,
59.5498906471691));
#170712=CARTESIAN_POINT('Ctrl Pts',(63.0153564584608,0.0139080571565023,
59.5502274527843));
#170713=CARTESIAN_POINT('Ctrl Pts',(63.0153617971604,0.0069540216278127,
59.55029950277));
#170714=CARTESIAN_POINT('Ctrl Pts',(63.0153743226244,-3.90012641998867E-11,
59.5503705382064));
#170715=CARTESIAN_POINT('Origin',(69.7358040552328,0.,40.0761166693274));
#170716=CARTESIAN_POINT('',(59.9621915011161,6.55335890299524E-10,43.6746029314002));
#170717=CARTESIAN_POINT('',(59.9459911121981,-3.64320804018464E-10,43.5827259602593));
#170718=CARTESIAN_POINT('',(59.6415245868576,-1.25526296912604E-15,41.8560104904131));
#170719=CARTESIAN_POINT('',(72.9974833261205,-9.75859007406187,40.5164212233382));
#170720=CARTESIAN_POINT('Ctrl Pts',(59.9621915011161,1.31067303586202E-9,
43.6746029314002));
#170721=CARTESIAN_POINT('Ctrl Pts',(59.9621173489605,0.0228571466064858,
43.6741823936118));
#170722=CARTESIAN_POINT('Ctrl Pts',(59.9621180799651,0.0457142985922821,
43.6737462492041));
#170723=CARTESIAN_POINT('Ctrl Pts',(59.9624078920643,0.133296489368093,
43.6720156346674));
#170724=CARTESIAN_POINT('Ctrl Pts',(59.9632226967352,0.198015867431952,
43.6706124157896));
#170725=CARTESIAN_POINT('Ctrl Pts',(59.9678600120166,0.409967523361952,
43.6656166008375));
#170726=CARTESIAN_POINT('Ctrl Pts',(59.9741929074607,0.557114709600572,
43.6615153088182));
#170727=CARTESIAN_POINT('Ctrl Pts',(59.998364587665,0.933224609434551,43.6494724853576));
#170728=CARTESIAN_POINT('Ctrl Pts',(60.0206520657771,1.16179318812559,43.6406704381945));
#170729=CARTESIAN_POINT('Ctrl Pts',(60.1378106502567,2.05585624406351,43.6007067186337));
#170730=CARTESIAN_POINT('Ctrl Pts',(60.289511129006,2.71176638524539,43.5593668052642));
#170731=CARTESIAN_POINT('Ctrl Pts',(60.5523720615392,3.49255424417903,43.4964316546202));
#170732=CARTESIAN_POINT('Ctrl Pts',(60.604378853226,3.63636565434677,43.4842343271781));
#170733=CARTESIAN_POINT('Ctrl Pts',(60.6958366926319,3.87267630363641,43.4631817307161));
#170734=CARTESIAN_POINT('Ctrl Pts',(60.7334847405298,3.96587194680139,43.4546131709443));
#170735=CARTESIAN_POINT('Ctrl Pts',(60.8113679101905,4.15081525954715,43.4370735516841));
#170736=CARTESIAN_POINT('Ctrl Pts',(60.8515905937239,4.24255632784152,43.4281047483983));
#170737=CARTESIAN_POINT('Ctrl Pts',(60.9560112778985,4.47155784408085,43.4050345898634));
#170738=CARTESIAN_POINT('Ctrl Pts',(61.0219073827158,4.60798972713239,43.3906642933388));
#170739=CARTESIAN_POINT('Ctrl Pts',(61.1741302317573,4.90611503719396,43.3578454249194));
#170740=CARTESIAN_POINT('Ctrl Pts',(61.2618115080646,5.06703334461495,43.3391809161984));
#170741=CARTESIAN_POINT('Ctrl Pts',(61.5805617291279,5.61643215419288,43.2720333696092));
#170742=CARTESIAN_POINT('Ctrl Pts',(61.8328107441819,5.99156763586135,43.2200948034707));
#170743=CARTESIAN_POINT('Ctrl Pts',(62.2780025896807,6.56733504541906,43.1292253869409));
#170744=CARTESIAN_POINT('Ctrl Pts',(62.4560175662718,6.77914880064797,43.0930538146435));
#170745=CARTESIAN_POINT('Ctrl Pts',(62.6974675926512,7.04378963482971,43.0439565774247));
#170746=CARTESIAN_POINT('Ctrl Pts',(62.7533793669096,7.10360488459081,43.0325847604572));
#170747=CARTESIAN_POINT('Ctrl Pts',(62.8481893238609,7.20261070306342,43.0132885449785));
#170748=CARTESIAN_POINT('Ctrl Pts',(62.8867037413048,7.24217909369355,43.0054462307965));
#170749=CARTESIAN_POINT('Ctrl Pts',(62.9716333422471,7.32802212488346,42.9881426304937));
#170750=CARTESIAN_POINT('Ctrl Pts',(63.0181746133971,7.37416200354657,42.9786543938634));
#170751=CARTESIAN_POINT('Ctrl Pts',(63.1646921582297,7.51662816108502,42.9487733654001));
#170752=CARTESIAN_POINT('Ctrl Pts',(63.2661683042383,7.6113220524863,42.9280627144475));
#170753=CARTESIAN_POINT('Ctrl Pts',(63.683676641712,7.98515581457783,42.842875281147));
#170754=CARTESIAN_POINT('Ctrl Pts',(64.0147467484473,8.2461738564164,42.7753930960578));
#170755=CARTESIAN_POINT('Ctrl Pts',(64.7129166745861,8.72869804795411,42.6341409547654));
#170756=CARTESIAN_POINT('Ctrl Pts',(65.0798374146058,8.94897057827151,42.560428361568));
#170757=CARTESIAN_POINT('Ctrl Pts',(65.5759815949015,9.20500908177388,42.4617082015838));
#170758=CARTESIAN_POINT('Ctrl Pts',(65.6936460591498,9.26281810691175,42.4383603462147));
#170759=CARTESIAN_POINT('Ctrl Pts',(65.8993561053364,9.35888780248268,42.3976544996312));
#170760=CARTESIAN_POINT('Ctrl Pts',(65.9868888909456,9.39823419833073,42.3803680453632));
#170761=CARTESIAN_POINT('Ctrl Pts',(66.1707762926584,9.47771320147651,42.3441237481254));
#170762=CARTESIAN_POINT('Ctrl Pts',(66.2672193832234,9.5176065801842,42.3251546585356));
#170763=CARTESIAN_POINT('Ctrl Pts',(66.5303000012563,9.62160599451012,42.2735135941002));
#170764=CARTESIAN_POINT('Ctrl Pts',(66.6980417425985,9.6827402026475,42.2406984428086));
#170765=CARTESIAN_POINT('Ctrl Pts',(67.2057678737193,9.85241545738296,42.1416605022513));
#170766=CARTESIAN_POINT('Ctrl Pts',(67.5499555697635,9.94713706253093,42.0749112681763));
#170767=CARTESIAN_POINT('Ctrl Pts',(68.3729831188539,10.1265021802317,41.9156916451335));
#170768=CARTESIAN_POINT('Ctrl Pts',(68.8543582772232,10.1948356872893,41.8228819554522));
#170769=CARTESIAN_POINT('Ctrl Pts',(69.4770026780229,10.2368873557742,41.7020779247071));
#170770=CARTESIAN_POINT('Ctrl Pts',(69.6155866148857,10.2433197476081,41.6751401055884));
#170771=CARTESIAN_POINT('Ctrl Pts',(69.8168134430169,10.2484171668224,41.635915800564));
#170772=CARTESIAN_POINT('Ctrl Pts',(69.879394580317,10.2494074474648,41.6237016685943));
#170773=CARTESIAN_POINT('Ctrl Pts',(69.9868439031305,10.2500863515925,41.6026997239521));
#170774=CARTESIAN_POINT('Ctrl Pts',(70.031709362798,10.2500640897533,41.5939209213597));
#170775=CARTESIAN_POINT('Ctrl Pts',(70.1410862974038,10.249264419133,41.5724962519277));
#170776=CARTESIAN_POINT('Ctrl Pts',(70.2055911165958,10.2481605107784,41.559842056356));
#170777=CARTESIAN_POINT('Ctrl Pts',(70.4209209722125,10.242363872947,41.5175440429169));
#170778=CARTESIAN_POINT('Ctrl Pts',(70.571638512008,10.2348455628059,41.4878467799212));
#170779=CARTESIAN_POINT('Ctrl Pts',(70.9625450467684,10.2063487386924,41.4106583962023));
#170780=CARTESIAN_POINT('Ctrl Pts',(71.2022447629782,10.1800199987766,41.3631666522352));
#170781=CARTESIAN_POINT('Ctrl Pts',(72.0951777882295,10.0486995648725,41.1860129444652));
#170782=CARTESIAN_POINT('Ctrl Pts',(72.7386402484642,9.88690701672744,41.0579901983043));
#170783=CARTESIAN_POINT('Ctrl Pts',(73.4925478435304,9.6147721265457,40.9087845182055));
#170784=CARTESIAN_POINT('Ctrl Pts',(73.6221561785561,9.56489518654855,40.8831577982836));
#170785=CARTESIAN_POINT('Ctrl Pts',(73.839744805898,9.47588736436761,40.8401767898018));
#170786=CARTESIAN_POINT('Ctrl Pts',(73.9282588973938,9.43817299578687,40.8227041079641));
#170787=CARTESIAN_POINT('Ctrl Pts',(74.1089292205463,9.35808061597936,40.7870625206487));
#170788=CARTESIAN_POINT('Ctrl Pts',(74.2010154417043,9.31556553328432,40.7689086618338));
#170789=CARTESIAN_POINT('Ctrl Pts',(74.4396917085287,9.20092390472612,40.7218838042689));
#170790=CARTESIAN_POINT('Ctrl Pts',(74.5852233809284,9.12657320745118,40.6932386751481));
#170791=CARTESIAN_POINT('Ctrl Pts',(74.8250778081425,8.99651990887481,40.6460542819881));
#170792=CARTESIAN_POINT('Ctrl Pts',(74.9203958179086,8.94279552140334,40.6273102682133));
#170793=CARTESIAN_POINT('Ctrl Pts',(75.3158959460101,8.71125304821846,40.5495440028411));
#170794=CARTESIAN_POINT('Ctrl Pts',(75.6078006929296,8.51923709816489,40.492174775107));
#170795=CARTESIAN_POINT('Ctrl Pts',(76.2045070451203,8.08049044573636,40.3744386786407));
#170796=CARTESIAN_POINT('Ctrl Pts',(76.5061781490616,7.83033589013045,40.3146322624727));
#170797=CARTESIAN_POINT('Ctrl Pts',(76.8632764293588,7.49723871979224,40.2428515583412));
#170798=CARTESIAN_POINT('Ctrl Pts',(76.9328689371494,7.43043143693812,40.228811623474));
#170799=CARTESIAN_POINT('Ctrl Pts',(77.0425255134659,7.32209786669668,40.2065927027049));
#170800=CARTESIAN_POINT('Ctrl Pts',(77.0832019609948,7.28121728359858,40.1983288871604));
#170801=CARTESIAN_POINT('Ctrl Pts',(77.1655949510218,7.19697848608749,40.1815412153398));
#170802=CARTESIAN_POINT('Ctrl Pts',(77.2072791305238,7.15359121425286,40.1730220518778));
#170803=CARTESIAN_POINT('Ctrl Pts',(77.3235043901774,7.03043367865424,40.1492000300661));
#170804=CARTESIAN_POINT('Ctrl Pts',(77.3971561861542,6.94981120634495,40.1340231108469));
#170805=CARTESIAN_POINT('Ctrl Pts',(77.5671917963301,6.75752477627966,40.0988159294102));
#170806=CARTESIAN_POINT('Ctrl Pts',(77.6624851149221,6.64489896507505,40.0789512984824));
#170807=CARTESIAN_POINT('Ctrl Pts',(78.0451683691847,6.17208490725915,39.9987104549053));
#170808=CARTESIAN_POINT('Ctrl Pts',(78.3106477829238,5.79426324545742,39.9419343747953));
#170809=CARTESIAN_POINT('Ctrl Pts',(78.709895369505,5.13555485717968,39.85538209849));
#170810=CARTESIAN_POINT('Ctrl Pts',(78.8579202449703,4.86447867345772,39.8229392144116));
#170811=CARTESIAN_POINT('Ctrl Pts',(79.0485049951672,4.47475917324987,39.7807255571288));
#170812=CARTESIAN_POINT('Ctrl Pts',(79.1013419507587,4.36154850676487,39.7689653621557));
#170813=CARTESIAN_POINT('Ctrl Pts',(79.1913152696655,4.15926374257341,39.7488361141225));
#170814=CARTESIAN_POINT('Ctrl Pts',(79.2292776224757,4.0705900938065,39.7403067915342));
#170815=CARTESIAN_POINT('Ctrl Pts',(79.3071811106906,3.88134112494089,39.7227233478217));
#170816=CARTESIAN_POINT('Ctrl Pts',(79.3467983331995,3.78063946443114,39.7137322934617));
#170817=CARTESIAN_POINT('Ctrl Pts',(79.4532281947511,3.49713415511864,39.6894306405052));
#170818=CARTESIAN_POINT('Ctrl Pts',(79.5164959258718,3.31299144033201,39.6748074869594));
#170819=CARTESIAN_POINT('Ctrl Pts',(79.6515049216347,2.88078099934798,39.6431138485946));
#170820=CARTESIAN_POINT('Ctrl Pts',(79.7192630951612,2.6315539187254,39.6268063790029));
#170821=CARTESIAN_POINT('Ctrl Pts',(79.8553469381881,2.04542344578551,39.5928183428281));
#170822=CARTESIAN_POINT('Ctrl Pts',(79.9164083023191,1.70707918399919,39.5764822130061));
#170823=CARTESIAN_POINT('Ctrl Pts',(80.0029096504755,1.0396177494775,39.5501129407671));
#170824=CARTESIAN_POINT('Ctrl Pts',(80.0296829682864,0.711099854667932,
39.5398580952606));
#170825=CARTESIAN_POINT('Ctrl Pts',(80.0435161808942,0.299867631964759,
39.5300357774177));
#170826=CARTESIAN_POINT('Ctrl Pts',(80.0453000397251,0.217898369552569,
39.5282267562018));
#170827=CARTESIAN_POINT('Ctrl Pts',(80.046624549247,0.0838834065347642,
39.5255040730306));
#170828=CARTESIAN_POINT('Ctrl Pts',(80.0467466390509,0.0318487197293709,
39.5245047644598));
#170829=CARTESIAN_POINT('Ctrl Pts',(80.0461810446212,-0.0770421743425323,
39.5225320751962));
#170830=CARTESIAN_POINT('Ctrl Pts',(80.0454173465967,-0.133896045883498,
39.5215700085654));
#170831=CARTESIAN_POINT('Ctrl Pts',(80.0419445200657,-0.294171634927588,
39.5190534947571));
#170832=CARTESIAN_POINT('Ctrl Pts',(80.0381542087308,-0.397565684268229,
39.5176598488733));
#170833=CARTESIAN_POINT('Ctrl Pts',(80.0257175206212,-0.638351979015838,
39.5149697493917));
#170834=CARTESIAN_POINT('Ctrl Pts',(80.015881642578,-0.775665347584725,
39.5138579199797));
#170835=CARTESIAN_POINT('Ctrl Pts',(79.9681294730664,-1.29673392045101,
39.5113161000226));
#170836=CARTESIAN_POINT('Ctrl Pts',(79.9115848938906,-1.67847948944964,
39.5129326313413));
#170837=CARTESIAN_POINT('Ctrl Pts',(79.7453491137976,-2.4878330276729,39.5245408991904));
#170838=CARTESIAN_POINT('Ctrl Pts',(79.6293893604218,-2.91336111157483,
39.5356926267131));
#170839=CARTESIAN_POINT('Ctrl Pts',(79.436317815401,-3.47799802302839,39.5577336475775));
#170840=CARTESIAN_POINT('Ctrl Pts',(79.3824275799282,-3.62471565578979,
39.564145826349));
#170841=CARTESIAN_POINT('Ctrl Pts',(79.2881949465286,-3.86442988438599,
39.5757625243229));
#170842=CARTESIAN_POINT('Ctrl Pts',(79.2497561460365,-3.95816437331337,
39.5805982594267));
#170843=CARTESIAN_POINT('Ctrl Pts',(79.1706894388021,-4.14321512524139,
39.5907297015011));
#170844=CARTESIAN_POINT('Ctrl Pts',(79.1301017712287,-4.2345369342463,39.5960178770899));
#170845=CARTESIAN_POINT('Ctrl Pts',(79.0256927379774,-4.46060257360602,
39.6098281622912));
#170846=CARTESIAN_POINT('Ctrl Pts',(78.9602813570908,-4.59456726527603,
39.6186593835295));
#170847=CARTESIAN_POINT('Ctrl Pts',(78.6993617524911,-5.10093193980778,
39.6545086894478));
#170848=CARTESIAN_POINT('Ctrl Pts',(78.4842466923207,-5.46248288743085,
39.6853245395268));
#170849=CARTESIAN_POINT('Ctrl Pts',(77.9759743733251,-6.20885361409864,
39.7598038940904));
#170850=CARTESIAN_POINT('Ctrl Pts',(77.6765978230205,-6.58808349054391,
39.8046077311431));
#170851=CARTESIAN_POINT('Ctrl Pts',(77.290641866474,-7.01159944329429,39.8623364442698));
#170852=CARTESIAN_POINT('Ctrl Pts',(77.2285883757945,-7.07789256832334,
39.8716162406021));
#170853=CARTESIAN_POINT('Ctrl Pts',(77.130166503438,-7.1802627397015,39.8863211949434));
#170854=CARTESIAN_POINT('Ctrl Pts',(77.0943915823113,-7.21691568138124,
39.891663501156));
#170855=CARTESIAN_POINT('Ctrl Pts',(77.0161053098073,-7.29592220348143,
39.9033454419194));
#170856=CARTESIAN_POINT('Ctrl Pts',(76.9734940530889,-7.33817187992911,
39.9096986641105));
#170857=CARTESIAN_POINT('Ctrl Pts',(76.8535436084434,-7.45502044706939,
39.9275733209952));
#170858=CARTESIAN_POINT('Ctrl Pts',(76.7754017126208,-7.52876698255031,
39.9392068607575));
#170859=CARTESIAN_POINT('Ctrl Pts',(76.4817043189845,-7.79728526459952,
39.9829276972726));
#170860=CARTESIAN_POINT('Ctrl Pts',(76.2590915117683,-7.98396200446055,
40.0160619804401));
#170861=CARTESIAN_POINT('Ctrl Pts',(75.5494288559673,-8.52909754940981,
40.1221845041652));
#170862=CARTESIAN_POINT('Ctrl Pts',(75.0385395243456,-8.8535292413592,40.1993245473084));
#170863=CARTESIAN_POINT('Ctrl Pts',(74.3812162984507,-9.19277637038211,
40.3003980655456));
#170864=CARTESIAN_POINT('Ctrl Pts',(74.2587588269137,-9.25286941293378,
40.319296020266));
#170865=CARTESIAN_POINT('Ctrl Pts',(74.0470333520821,-9.35149847965907,
40.3520884572869));
#170866=CARTESIAN_POINT('Ctrl Pts',(73.9583410299252,-9.39126526229129,
40.3658600374334));
#170867=CARTESIAN_POINT('Ctrl Pts',(73.7874146030616,-9.46495489953998,
40.3924658912069));
#170868=CARTESIAN_POINT('Ctrl Pts',(73.7052763221112,-9.49908431976494,
40.4052797349676));
#170869=CARTESIAN_POINT('Ctrl Pts',(73.5306247219921,-9.56895706967644,
40.4325841311828));
#170870=CARTESIAN_POINT('Ctrl Pts',(73.4380164429053,-9.60442909177834,
40.4470962130776));
#170871=CARTESIAN_POINT('Ctrl Pts',(73.2298227428336,-9.68066566216209,
40.4797924347375));
#170872=CARTESIAN_POINT('Ctrl Pts',(73.1139937762474,-9.7206951460624,40.4980316609364));
#170873=CARTESIAN_POINT('Ctrl Pts',(72.9974833261205,-9.75859007406187,
40.5164212233382));
#170874=CARTESIAN_POINT('',(76.8678595013252,-7.42547303891629,39.8339694781585));
#170875=CARTESIAN_POINT('Origin',(69.9094522328998,0.,41.0609244223396));
#170876=CARTESIAN_POINT('Ctrl Pts',(76.8678595013252,-7.42547303891629,
39.8339694781584));
#170877=CARTESIAN_POINT('Ctrl Pts',(76.8990285746249,-7.39548789751561,
39.8292694255059));
#170878=CARTESIAN_POINT('Ctrl Pts',(76.9300033038781,-7.36530950731916,
39.8246101125015));
#170879=CARTESIAN_POINT('Ctrl Pts',(76.9890950918522,-7.3070029802757,39.8157448866622));
#170880=CARTESIAN_POINT('Ctrl Pts',(77.0172338774585,-7.27891310035191,
39.811533799747));
#170881=CARTESIAN_POINT('Ctrl Pts',(77.0856086872409,-7.20985852939954,
39.8013283125404));
#170882=CARTESIAN_POINT('Ctrl Pts',(77.1256682594321,-7.16871548356406,
39.7953724164883));
#170883=CARTESIAN_POINT('Ctrl Pts',(77.2311477720555,-7.05854733117038,
39.7797484782629));
#170884=CARTESIAN_POINT('Ctrl Pts',(77.295966387408,-6.98893604171636,39.7702080620901));
#170885=CARTESIAN_POINT('Ctrl Pts',(77.6305655574832,-6.61942870337986,
39.7212469538832));
#170886=CARTESIAN_POINT('Ctrl Pts',(77.8836889316479,-6.30448353077214,
39.6851960134421));
#170887=CARTESIAN_POINT('Ctrl Pts',(78.4029737335433,-5.57414804881995,
39.6126427073769));
#170888=CARTESIAN_POINT('Ctrl Pts',(78.6592508879664,-5.15278013234336,
39.57783655874));
#170889=CARTESIAN_POINT('Ctrl Pts',(78.9516653474975,-4.58383576110372,
39.5390626495023));
#170890=CARTESIAN_POINT('Ctrl Pts',(79.0160016307363,-4.45180144374981,
39.530607907952));
#170891=CARTESIAN_POINT('Ctrl Pts',(79.1191926701759,-4.2280246383929,39.5171765521302));
#170892=CARTESIAN_POINT('Ctrl Pts',(79.1595712596385,-4.13702419646794,
39.5119580218592));
#170893=CARTESIAN_POINT('Ctrl Pts',(79.2385572431532,-3.95184115846412,
39.5018279559135));
#170894=CARTESIAN_POINT('Ctrl Pts',(79.2771013330322,-3.85764308504231,
39.4969263200327));
#170895=CARTESIAN_POINT('Ctrl Pts',(79.3722209894594,-3.61501995471575,
39.4849435078869));
#170896=CARTESIAN_POINT('Ctrl Pts',(79.4267846515862,-3.4658199729671,39.4781815291744));
#170897=CARTESIAN_POINT('Ctrl Pts',(79.6393390113098,-2.84033980478241,
39.4523692131195));
#170898=CARTESIAN_POINT('Ctrl Pts',(79.7660895075844,-2.35398540594275,
39.4382963459358));
#170899=CARTESIAN_POINT('Ctrl Pts',(79.918371690702,-1.5290448733026,39.4251794611873));
#170900=CARTESIAN_POINT('Ctrl Pts',(79.963395685683,-1.1950133641786,39.4227322356103));
#170901=CARTESIAN_POINT('Ctrl Pts',(80.0080462612809,-0.674516161978915,
39.4237578630503));
#170902=CARTESIAN_POINT('Ctrl Pts',(80.0189721768199,-0.489257118968895,
39.4250665478881));
#170903=CARTESIAN_POINT('Ctrl Pts',(80.0272276639154,-0.23370677680595,
39.4282457473849));
#170904=CARTESIAN_POINT('Ctrl Pts',(80.0287868895687,-0.163577834301707,
39.4292606182179));
#170905=CARTESIAN_POINT('Ctrl Pts',(80.0302602635132,-0.0425597037715466,
39.4312630645013));
#170906=CARTESIAN_POINT('Ctrl Pts',(80.0305085519828,0.00832354220289945,
39.4321818150966));
#170907=CARTESIAN_POINT('Ctrl Pts',(80.0302337913538,0.122148487738307,
39.4344098758722));
#170908=CARTESIAN_POINT('Ctrl Pts',(80.0295138785973,0.185086082590115,
39.4357595574041));
#170909=CARTESIAN_POINT('Ctrl Pts',(80.0254343796904,0.384367694243806,
39.4403996303459));
#170910=CARTESIAN_POINT('Ctrl Pts',(80.0199751212635,0.520644196063558,
39.4441161654749));
#170911=CARTESIAN_POINT('Ctrl Pts',(79.9820996429936,1.15498961354795,39.4638611414359));
#170912=CARTESIAN_POINT('Ctrl Pts',(79.9166508322399,1.6502162462987,39.4862837367131));
#170913=CARTESIAN_POINT('Ctrl Pts',(79.7371277022152,2.52022778367019,39.5369688694709));
#170914=CARTESIAN_POINT('Ctrl Pts',(79.6369242658023,2.89701110402737,39.5628547848345));
#170915=CARTESIAN_POINT('Ctrl Pts',(79.4636815455327,3.42597023401457,39.6046748539072));
#170916=CARTESIAN_POINT('Ctrl Pts',(79.4077692912873,3.58360973267206,39.6178607972264));
#170917=CARTESIAN_POINT('Ctrl Pts',(79.3112175035052,3.83613493849726,39.6401589588782));
#170918=CARTESIAN_POINT('Ctrl Pts',(79.272933952288,3.93192072117163,39.6488964259421));
#170919=CARTESIAN_POINT('Ctrl Pts',(79.1958155300578,4.11675596164734,39.6663043427833));
#170920=CARTESIAN_POINT('Ctrl Pts',(79.1571451961852,4.20586455879665,39.6749484356336));
#170921=CARTESIAN_POINT('Ctrl Pts',(79.0690856502033,4.40115295012384,39.6944543856953));
#170922=CARTESIAN_POINT('Ctrl Pts',(79.0191353558858,4.50705563096255,39.7054049367983));
#170923=CARTESIAN_POINT('Ctrl Pts',(78.8056406730932,4.94033148362395,39.7517720560935));
#170924=CARTESIAN_POINT('Ctrl Pts',(78.6265591937485,5.25947349456486,39.7896551829451));
#170925=CARTESIAN_POINT('Ctrl Pts',(78.2116804948403,5.91409987506177,39.8759311392482));
#170926=CARTESIAN_POINT('Ctrl Pts',(77.9720229012634,6.24628086098109,39.9249606399178));
#170927=CARTESIAN_POINT('Ctrl Pts',(77.6246178158771,6.67146949341581,39.9956966378726));
#170928=CARTESIAN_POINT('Ctrl Pts',(77.5336591481646,6.77821698227307,40.0141911967846));
#170929=CARTESIAN_POINT('Ctrl Pts',(77.3705838108441,6.96178471729201,40.0473476947724));
#170930=CARTESIAN_POINT('Ctrl Pts',(77.2994058850546,7.0394439411327,40.0618191768485));
#170931=CARTESIAN_POINT('Ctrl Pts',(77.1862350714393,7.15913500881618,40.0848449318188));
#170932=CARTESIAN_POINT('Ctrl Pts',(77.1450411747064,7.20194430764065,40.0932295683592));
#170933=CARTESIAN_POINT('Ctrl Pts',(77.0676782118854,7.28094345440789,40.1089860008795));
#170934=CARTESIAN_POINT('Ctrl Pts',(77.0316043901696,7.31722787839537,40.1163371104082));
#170935=CARTESIAN_POINT('Ctrl Pts',(76.9302526726861,7.41764188748027,40.1369984532148));
#170936=CARTESIAN_POINT('Ctrl Pts',(76.8643922015006,7.48115089376309,40.1504336311935));
#170937=CARTESIAN_POINT('Ctrl Pts',(76.3980520662467,7.91880977020058,40.2455832329278));
#170938=CARTESIAN_POINT('Ctrl Pts',(75.9692665279844,8.26020280735344,40.3331178885577));
#170939=CARTESIAN_POINT('Ctrl Pts',(75.2985069547894,8.70999833087118,40.4686098847352));
#170940=CARTESIAN_POINT('Ctrl Pts',(75.0761544622313,8.84680697144869,40.5133230576833));
#170941=CARTESIAN_POINT('Ctrl Pts',(74.7695648199348,9.01926273357357,40.5746330733728));
#170942=CARTESIAN_POINT('Ctrl Pts',(74.6897242445181,9.06274676450101,40.5905692816809));
#170943=CARTESIAN_POINT('Ctrl Pts',(74.4822279790979,9.17210369399836,40.6319057495574));
#170944=CARTESIAN_POINT('Ctrl Pts',(74.3537413525391,9.23630923447455,40.6574253326405));
#170945=CARTESIAN_POINT('Ctrl Pts',(74.1354185870535,9.3395650965652,40.7006561014693));
#170946=CARTESIAN_POINT('Ctrl Pts',(74.0462972422509,9.38011621502275,40.7182673050036));
#170947=CARTESIAN_POINT('Ctrl Pts',(73.8753841785891,9.45485715834273,40.7519737138198));
#170948=CARTESIAN_POINT('Ctrl Pts',(73.7937028210593,9.4892827629088,40.7680535087685));
#170949=CARTESIAN_POINT('Ctrl Pts',(73.5757808526759,9.57771432433733,40.8108794385776));
#170950=CARTESIAN_POINT('Ctrl Pts',(73.4388036548674,9.62979930375277,40.837721877349));
#170951=CARTESIAN_POINT('Ctrl Pts',(72.674124477842,9.90134916431078,40.9871888510873));
#170952=CARTESIAN_POINT('Ctrl Pts',(72.0271611616332,10.0601723356113,41.1121153475183));
#170953=CARTESIAN_POINT('Ctrl Pts',(71.1425330131848,10.1850166898584,41.2830892933127));
#170954=CARTESIAN_POINT('Ctrl Pts',(70.9144637961712,10.2091524228976,41.3271956911357));
#170955=CARTESIAN_POINT('Ctrl Pts',(70.5400256272296,10.2356556234102,41.3998228763409));
#170956=CARTESIAN_POINT('Ctrl Pts',(70.394049029545,10.2427390308062,41.4281904026554));
#170957=CARTESIAN_POINT('Ctrl Pts',(70.1842294733845,10.2482598716852,41.4690843290307));
#170958=CARTESIAN_POINT('Ctrl Pts',(70.1204592708199,10.2493199595284,41.4815290851168));
#170959=CARTESIAN_POINT('Ctrl Pts',(70.0068811527501,10.2501078748424,41.5037268454323));
#170960=CARTESIAN_POINT('Ctrl Pts',(69.9570765267565,10.2500766201812,41.5134723015878));
#170961=CARTESIAN_POINT('Ctrl Pts',(69.8420581847569,10.2491342981117,41.5360050517938));
#170962=CARTESIAN_POINT('Ctrl Pts',(69.7768509474777,10.2479538840617,41.5487988724902));
#170963=CARTESIAN_POINT('Ctrl Pts',(69.5665371123725,10.2420616783078,41.5901176442255));
#170964=CARTESIAN_POINT('Ctrl Pts',(69.4215302454519,10.234795177056,41.6186899135523));
#170965=CARTESIAN_POINT('Ctrl Pts',(68.4696077886515,10.1660138608211,41.8066451880225));
#170966=CARTESIAN_POINT('Ctrl Pts',(67.6725851893531,10.0086501410841,41.9655895428828));
#170967=CARTESIAN_POINT('Ctrl Pts',(66.7236348913335,9.69686408548901,42.1536230990952));
#170968=CARTESIAN_POINT('Ctrl Pts',(66.5464194445875,9.63300004668673,42.1886978194846));
#170969=CARTESIAN_POINT('Ctrl Pts',(66.2722638634957,9.52530485355145,42.2428876051179));
#170970=CARTESIAN_POINT('Ctrl Pts',(66.1740777165832,9.48490985429102,42.262280687351));
#170971=CARTESIAN_POINT('Ctrl Pts',(65.9888791377432,9.40523036584957,42.2988334914227));
#170972=CARTESIAN_POINT('Ctrl Pts',(65.9017526755059,9.36625267307211,42.3160184288552));
#170973=CARTESIAN_POINT('Ctrl Pts',(65.7020464373638,9.27344606329649,42.3553853881296));
#170974=CARTESIAN_POINT('Ctrl Pts',(65.5898759105557,9.21873771633629,42.3774794533091));
#170975=CARTESIAN_POINT('Ctrl Pts',(65.2014965573261,9.02021804661125,42.4539324068031));
#170976=CARTESIAN_POINT('Ctrl Pts',(64.9308299837578,8.86552166540736,42.5071262200063));
#170977=CARTESIAN_POINT('Ctrl Pts',(64.2866946003729,8.4563710629904,42.6338073921607));
#170978=CARTESIAN_POINT('Ctrl Pts',(63.9221101920738,8.18870661371439,42.7055779139455));
#170979=CARTESIAN_POINT('Ctrl Pts',(63.464653865196,7.80286662160835,42.7965793118998));
#170980=CARTESIAN_POINT('Ctrl Pts',(63.3549227002082,7.70614968893859,42.818489265235));
#170981=CARTESIAN_POINT('Ctrl Pts',(63.1674400891867,7.53350670885597,42.8561159797199));
#170982=CARTESIAN_POINT('Ctrl Pts',(63.0887526019016,7.45866379174902,42.8719701145718));
#170983=CARTESIAN_POINT('Ctrl Pts',(62.9684381653949,7.34046815037003,42.8963277451624));
#170984=CARTESIAN_POINT('Ctrl Pts',(62.9259756637275,7.29800195607488,42.9049475465382));
#170985=CARTESIAN_POINT('Ctrl Pts',(62.8434240876446,7.21395562638395,42.9217555361425));
#170986=CARTESIAN_POINT('Ctrl Pts',(62.8033082706967,7.17240601497427,42.9299474042846));
#170987=CARTESIAN_POINT('Ctrl Pts',(62.696834408525,7.06021662695402,42.9517506682705));
#170988=CARTESIAN_POINT('Ctrl Pts',(62.6311236833974,6.98895283042766,42.9652709750419));
#170989=CARTESIAN_POINT('Ctrl Pts',(62.2192988284285,6.52924229277284,43.0503751758264));
#170990=CARTESIAN_POINT('Ctrl Pts',(61.9021320626343,6.11509303133995,43.1175762416949));
#170991=CARTESIAN_POINT('Ctrl Pts',(61.4684418428818,5.44882528130082,43.210900835275));
#170992=CARTESIAN_POINT('Ctrl Pts',(61.3284373037179,5.21365403011963,43.2413240604058));
#170993=CARTESIAN_POINT('Ctrl Pts',(61.1031071075094,4.7982550081286,43.2907177272806));
#170994=CARTESIAN_POINT('Ctrl Pts',(61.0133551765301,4.62070523803238,43.3105333202156));
#170995=CARTESIAN_POINT('Ctrl Pts',(60.8825753724263,4.34225659141649,43.3396217908423));
#170996=CARTESIAN_POINT('Ctrl Pts',(60.8379382180383,4.24318147026431,43.3495942591852));
#170997=CARTESIAN_POINT('Ctrl Pts',(60.7566758520312,4.05493621894353,43.3678352123577));
#170998=CARTESIAN_POINT('Ctrl Pts',(60.7197204517938,3.96592785976959,43.376167717492));
#170999=CARTESIAN_POINT('Ctrl Pts',(60.6380742271444,3.76124565852801,43.3946662102358));
#171000=CARTESIAN_POINT('Ctrl Pts',(60.5942028810397,3.64524710709357,43.4046729206937));
#171001=CARTESIAN_POINT('Ctrl Pts',(60.4537665704898,3.25275197961635,43.4369514375245));
#171002=CARTESIAN_POINT('Ctrl Pts',(60.3667968015805,2.97282680911703,43.4573653843859));
#171003=CARTESIAN_POINT('Ctrl Pts',(60.2748146619763,2.62545634078586,43.4796507789828));
#171004=CARTESIAN_POINT('Ctrl Pts',(60.2584787769182,2.56128895432738,43.4836423840945));
#171005=CARTESIAN_POINT('Ctrl Pts',(60.1234629266166,2.00888984379493,43.5169456414411));
#171006=CARTESIAN_POINT('Ctrl Pts',(60.0396715483063,1.51245742901374,43.5397563499562));
#171007=CARTESIAN_POINT('Ctrl Pts',(59.9708782351334,0.786683988483576,
43.5641630169089));
#171008=CARTESIAN_POINT('Ctrl Pts',(59.9569046242807,0.561003863913369,
43.570523119053));
#171009=CARTESIAN_POINT('Ctrl Pts',(59.9481523568033,0.260411614599621,
43.5774956935159));
#171010=CARTESIAN_POINT('Ctrl Pts',(59.9467861842967,0.18577909152811,43.5791043272761));
#171011=CARTESIAN_POINT('Ctrl Pts',(59.9459496143772,0.0740918169188201,
43.5813340252946));
#171012=CARTESIAN_POINT('Ctrl Pts',(59.9458709289595,0.0370460643766788,
43.5820443672582));
#171013=CARTESIAN_POINT('Ctrl Pts',(59.9459911121981,-7.28640352773959E-10,
43.5827259602593));
#171014=CARTESIAN_POINT('Origin',(69.7358040552328,0.,40.0761166693274));
#171015=CARTESIAN_POINT('',(60.1705693073443,2.15049072447686E-6,44.8563721954731));
#171016=CARTESIAN_POINT('',(60.1543689253998,-5.77418479642888E-10,44.7644952638818));
#171017=CARTESIAN_POINT('',(59.6415245868576,-1.25526296912604E-15,41.8560104904131));
#171018=CARTESIAN_POINT('Ctrl Pts',(60.1705693073443,2.15049072447686E-6,
44.8563721954731));
#171019=CARTESIAN_POINT('Ctrl Pts',(60.1704255439564,0.044319522617042,
44.8555568192404));
#171020=CARTESIAN_POINT('Ctrl Pts',(60.1705632383758,0.0886262742527372,
44.8546829874787));
#171021=CARTESIAN_POINT('Ctrl Pts',(60.1715249939329,0.190262826338394,
44.8525455399988));
#171022=CARTESIAN_POINT('Ctrl Pts',(60.1725386634808,0.24757857132914,44.851243168513));
#171023=CARTESIAN_POINT('Ctrl Pts',(60.1780873034733,0.461678724818797,
44.846021289225));
#171024=CARTESIAN_POINT('Ctrl Pts',(60.1856796859077,0.618347621851348,
44.8414849048274));
#171025=CARTESIAN_POINT('Ctrl Pts',(60.2352514242262,1.31563187889683,44.8182311328369));
#171026=CARTESIAN_POINT('Ctrl Pts',(60.3158132347216,1.85239267216816,44.7921429505985));
#171027=CARTESIAN_POINT('Ctrl Pts',(60.496083572513,2.63157607779585,44.7433425718599));
#171028=CARTESIAN_POINT('Ctrl Pts',(60.5636603217285,2.88079739688011,44.72601359766));
#171029=CARTESIAN_POINT('Ctrl Pts',(60.6984329542329,3.31300003676053,44.6929898169196));
#171030=CARTESIAN_POINT('Ctrl Pts',(60.7616251099477,3.49713991596297,44.6779436237939));
#171031=CARTESIAN_POINT('Ctrl Pts',(60.867985974017,3.78064376844652,44.6532527619124));
#171032=CARTESIAN_POINT('Ctrl Pts',(60.9075878649764,3.88134492149082,44.6441757815022));
#171033=CARTESIAN_POINT('Ctrl Pts',(60.9854807615025,4.07059365435046,44.6265322693778));
#171034=CARTESIAN_POINT('Ctrl Pts',(61.0234457822407,4.15926739726915,44.618017701498));
#171035=CARTESIAN_POINT('Ctrl Pts',(61.1134425585809,4.3615526780029,44.5980194586427));
#171036=CARTESIAN_POINT('Ctrl Pts',(61.1663055552607,4.47476422131632,44.5864043415833));
#171037=CARTESIAN_POINT('Ctrl Pts',(61.3570238261799,4.86449146664188,44.5449234402758));
#171038=CARTESIAN_POINT('Ctrl Pts',(61.5052200292013,5.1355786498999,44.5134151024511));
#171039=CARTESIAN_POINT('Ctrl Pts',(61.9049887878862,5.79429098218372,44.4297809731763));
#171040=CARTESIAN_POINT('Ctrl Pts',(62.1708670338384,6.17210203586741,44.375301394302));
#171041=CARTESIAN_POINT('Ctrl Pts',(62.5539340471743,6.64490599185717,44.297280985997));
#171042=CARTESIAN_POINT('Ctrl Pts',(62.6493093980692,6.75753047789234,44.2778868575379));
#171043=CARTESIAN_POINT('Ctrl Pts',(62.8194514240044,6.94981479463985,44.2432933370539));
#171044=CARTESIAN_POINT('Ctrl Pts',(62.8931372911015,7.0304365990296,44.228312610868));
#171045=CARTESIAN_POINT('Ctrl Pts',(63.0093911900475,7.1535927499084,44.2046604536838));
#171046=CARTESIAN_POINT('Ctrl Pts',(63.051081244933,7.1969798918094,44.1961751949651));
#171047=CARTESIAN_POINT('Ctrl Pts',(63.133475470328,7.28121862649367,44.1793947693533));
#171048=CARTESIAN_POINT('Ctrl Pts',(63.1741476806585,7.32209928440839,44.1711063476643));
#171049=CARTESIAN_POINT('Ctrl Pts',(63.2837819804715,7.43043383051258,44.1487550811757));
#171050=CARTESIAN_POINT('Ctrl Pts',(63.3533481592734,7.49724151193889,44.1345629000235));
#171051=CARTESIAN_POINT('Ctrl Pts',(63.7102379452026,7.8303157962833,44.0617423766876));
#171052=CARTESIAN_POINT('Ctrl Pts',(64.0115750148459,8.08044522957783,44.0002314552037));
#171053=CARTESIAN_POINT('Ctrl Pts',(64.6076836801177,8.51918299615302,43.8792630898112));
#171054=CARTESIAN_POINT('Ctrl Pts',(64.8993390431828,8.71121564743694,43.8203647594883));
#171055=CARTESIAN_POINT('Ctrl Pts',(65.2946093242197,8.94277663363288,43.7411317988175));
#171056=CARTESIAN_POINT('Ctrl Pts',(65.389876630923,8.99650370569618,43.7220771734533));
#171057=CARTESIAN_POINT('Ctrl Pts',(65.6296224175688,9.12656163676907,43.6742358849136));
#171058=CARTESIAN_POINT('Ctrl Pts',(65.7751076266834,9.20091494725499,43.6453029153465));
#171059=CARTESIAN_POINT('Ctrl Pts',(66.0137429955704,9.31555992474666,43.5980099606362));
#171060=CARTESIAN_POINT('Ctrl Pts',(66.1058202200845,9.35807551534762,43.5798006983418));
#171061=CARTESIAN_POINT('Ctrl Pts',(66.2864886000496,9.43816827008255,43.5441461631412));
#171062=CARTESIAN_POINT('Ctrl Pts',(66.3750087861485,9.47588256072015,43.5267111117354));
#171063=CARTESIAN_POINT('Ctrl Pts',(66.5926281127583,9.56488892941394,43.4839294927927));
#171064=CARTESIAN_POINT('Ctrl Pts',(66.7222701492106,9.61476500451744,43.4585120757762));
#171065=CARTESIAN_POINT('Ctrl Pts',(67.4764781670717,9.88690200561605,43.3110061088934));
#171066=CARTESIAN_POINT('Ctrl Pts',(68.1205943078348,10.0487024228311,43.186575724765));
#171067=CARTESIAN_POINT('Ctrl Pts',(69.0143425374277,10.1800240126983,43.0138548861445));
#171068=CARTESIAN_POINT('Ctrl Pts',(69.2542296819376,10.2063509474823,42.9674745222301));
#171069=CARTESIAN_POINT('Ctrl Pts',(69.6004044869966,10.2315711849265,42.9003410817753));
#171070=CARTESIAN_POINT('Ctrl Pts',(69.7061292514836,10.2375676435575,42.8798105480313));
#171071=CARTESIAN_POINT('Ctrl Pts',(69.8967200090483,10.2453073872475,42.8427303618961));
#171072=CARTESIAN_POINT('Ctrl Pts',(69.9815547331096,10.2476581851155,42.8262005905712));
#171073=CARTESIAN_POINT('Ctrl Pts',(70.1188155339306,10.2496923204523,42.7994057882111));
#171074=CARTESIAN_POINT('Ctrl Pts',(70.1712314968081,10.2500517997528,42.7891618178983));
#171075=CARTESIAN_POINT('Ctrl Pts',(70.2783408274154,10.2499336729321,42.76820175232));
#171076=CARTESIAN_POINT('Ctrl Pts',(70.3330320179782,10.2494189562434,42.7574850875006));
#171077=CARTESIAN_POINT('Ctrl Pts',(70.4837238492593,10.2467484629841,42.7279219820349));
#171078=CARTESIAN_POINT('Ctrl Pts',(70.5796976098612,10.243646539479,42.7090541965003));
#171079=CARTESIAN_POINT('Ctrl Pts',(71.2343127941338,10.2129229516261,42.580143329448));
#171080=CARTESIAN_POINT('Ctrl Pts',(71.7897217646185,10.1392630019662,42.4697373880899));
#171081=CARTESIAN_POINT('Ctrl Pts',(72.6774250788273,9.94381380994694,42.2934205579085));
#171082=CARTESIAN_POINT('Ctrl Pts',(73.0145363486329,9.8506409414843,42.2264858167201));
#171083=CARTESIAN_POINT('Ctrl Pts',(73.5156923673857,9.68315989648576,42.1272022106212));
#171084=CARTESIAN_POINT('Ctrl Pts',(73.6836442204659,9.62194670070529,42.0939665145021));
#171085=CARTESIAN_POINT('Ctrl Pts',(73.9469871844002,9.51784016813432,42.0419191438102));
#171086=CARTESIAN_POINT('Ctrl Pts',(74.0434680579532,9.47793239236348,42.0228645502519));
#171087=CARTESIAN_POINT('Ctrl Pts',(74.2273835720304,9.39844897974591,41.9865676574354));
#171088=CARTESIAN_POINT('Ctrl Pts',(74.314905967817,9.35911469835312,41.9693059225534));
#171089=CARTESIAN_POINT('Ctrl Pts',(74.5205123278379,9.26312021661874,41.9287788807951));
#171090=CARTESIAN_POINT('Ctrl Pts',(74.6380926422076,9.20537831638721,41.9056217376954));
#171091=CARTESIAN_POINT('Ctrl Pts',(75.106018253574,8.96404741834731,41.8135204116345));
#171092=CARTESIAN_POINT('Ctrl Pts',(75.4467689884151,8.76189028604758,41.7465923191755));
#171093=CARTESIAN_POINT('Ctrl Pts',(76.0869348626083,8.32889507682514,41.6205837505826));
#171094=CARTESIAN_POINT('Ctrl Pts',(76.3870566723647,8.10031556226049,41.561374723565));
#171095=CARTESIAN_POINT('Ctrl Pts',(76.7765438108752,7.76749541067642,41.4838081207003));
#171096=CARTESIAN_POINT('Ctrl Pts',(76.8774633495982,7.67768718311102,41.4636368981732));
#171097=CARTESIAN_POINT('Ctrl Pts',(77.0518293647839,7.51612138903478,41.428616315608));
#171098=CARTESIAN_POINT('Ctrl Pts',(77.1260310612677,7.44523216914281,41.4136567295806));
#171099=CARTESIAN_POINT('Ctrl Pts',(77.2410925400592,7.33189808863244,41.3903532688205));
#171100=CARTESIAN_POINT('Ctrl Pts',(77.2826744187369,7.29021725883324,41.3819091198612));
#171101=CARTESIAN_POINT('Ctrl Pts',(77.3599430814493,7.21139676583721,41.3661715975547));
#171102=CARTESIAN_POINT('Ctrl Pts',(77.3957139398822,7.17434443853985,41.3588669591122));
#171103=CARTESIAN_POINT('Ctrl Pts',(77.4956308479103,7.06925111262193,41.3384123581069));
#171104=CARTESIAN_POINT('Ctrl Pts',(77.5591268084516,7.00058144592475,41.325353646242));
#171105=CARTESIAN_POINT('Ctrl Pts',(77.9195724797514,6.599756598571,41.2509104659163));
#171106=CARTESIAN_POINT('Ctrl Pts',(78.1955792805213,6.24883939102378,41.1926748869468));
#171107=CARTESIAN_POINT('Ctrl Pts',(78.7098957651985,5.49845019218121,41.0826207823401));
#171108=CARTESIAN_POINT('Ctrl Pts',(78.9458107585613,5.09851772952473,41.031258550513));
#171109=CARTESIAN_POINT('Ctrl Pts',(79.2174723675086,4.55742509420517,40.9712472424416));
#171110=CARTESIAN_POINT('Ctrl Pts',(79.2782138090284,4.42997847584416,40.9577570927977));
#171111=CARTESIAN_POINT('Ctrl Pts',(79.3768412566637,4.21161040246182,40.9357285122937));
#171112=CARTESIAN_POINT('Ctrl Pts',(79.4160675084637,4.1213432053878,40.9269300458601));
#171113=CARTESIAN_POINT('Ctrl Pts',(79.4936301304731,3.93564231489199,40.9094535020662));
#171114=CARTESIAN_POINT('Ctrl Pts',(79.5318451999104,3.84016787462365,40.900799126533));
#171115=CARTESIAN_POINT('Ctrl Pts',(79.6278364120737,3.58958159601358,40.8789389978898));
#171116=CARTESIAN_POINT('Ctrl Pts',(79.6833396296783,3.43359367398906,40.8661743422649));
#171117=CARTESIAN_POINT('Ctrl Pts',(79.9416392350219,2.64857230428485,40.8060544529767));
#171118=CARTESIAN_POINT('Ctrl Pts',(80.0879373965521,2.00181501077962,40.7696638583571));
#171119=CARTESIAN_POINT('Ctrl Pts',(80.1995400765391,1.12657467356358,40.735399786807));
#171120=CARTESIAN_POINT('Ctrl Pts',(80.2204452889702,0.907197634177053,
40.7280260479068));
#171121=CARTESIAN_POINT('Ctrl Pts',(80.2433907346824,0.544223252651627,
40.7176810132585));
#171122=CARTESIAN_POINT('Ctrl Pts',(80.2494678294453,0.400973136692729,
40.71407258984));
#171123=CARTESIAN_POINT('Ctrl Pts',(80.2539563570033,0.193552747041624,
40.7094954915821));
#171124=CARTESIAN_POINT('Ctrl Pts',(80.2547483208994,0.129459205751225,
40.7081705364979));
#171125=CARTESIAN_POINT('Ctrl Pts',(80.255100920087,0.0145775709653826,
40.7059514906647));
#171126=CARTESIAN_POINT('Ctrl Pts',(80.2548831092962,-0.0362062436283323,
40.7050247949784));
#171127=CARTESIAN_POINT('Ctrl Pts',(80.2535063607505,-0.154416988821826,
40.7029943333017));
#171128=CARTESIAN_POINT('Ctrl Pts',(80.2520624162441,-0.221838426712053,
40.7019326063345));
#171129=CARTESIAN_POINT('Ctrl Pts',(80.2451677638437,-0.442935493740978,
40.6987748722631));
#171130=CARTESIAN_POINT('Ctrl Pts',(80.2369549850655,-0.596510272815278,
40.6970953967244));
#171131=CARTESIAN_POINT('Ctrl Pts',(80.1634693289375,-1.56610449762325,
40.6899144716912));
#171132=CARTESIAN_POINT('Ctrl Pts',(80.0053183119484,-2.37226317618852,
40.6995494146783));
#171133=CARTESIAN_POINT('Ctrl Pts',(79.6963960163447,-3.332170090917,40.7334733134641));
#171134=CARTESIAN_POINT('Ctrl Pts',(79.6331912676002,-3.51155099444106,
40.7408180233016));
#171135=CARTESIAN_POINT('Ctrl Pts',(79.5265981742277,-3.78951510215392,
40.7537952416134));
#171136=CARTESIAN_POINT('Ctrl Pts',(79.4865245648172,-3.88935231860143,
40.7587859707903));
#171137=CARTESIAN_POINT('Ctrl Pts',(79.407419779681,-4.07790713533195,40.7688409796));
#171138=CARTESIAN_POINT('Ctrl Pts',(79.368681742007,-4.1667380292011,40.7738486070063));
#171139=CARTESIAN_POINT('Ctrl Pts',(79.2763176601259,-4.37069828847553,
40.7859726570874));
#171140=CARTESIAN_POINT('Ctrl Pts',(79.2218144948323,-4.48540258671413,
40.7932597806484));
#171141=CARTESIAN_POINT('Ctrl Pts',(79.0189807899978,-4.892797214755,40.8208200787647));
#171142=CARTESIAN_POINT('Ctrl Pts',(78.8589425892462,-5.17927701523856,
40.8433637815059));
#171143=CARTESIAN_POINT('Ctrl Pts',(78.4503012656289,-5.83533564463955,
40.9023110919439));
#171144=CARTESIAN_POINT('Ctrl Pts',(78.1909464253384,-6.19723727250574,
40.940731406425));
#171145=CARTESIAN_POINT('Ctrl Pts',(77.8167151048648,-6.65359690702007,
40.9965870950902));
#171146=CARTESIAN_POINT('Ctrl Pts',(77.721926373189,-6.7642804461397,41.0107638368156));
#171147=CARTESIAN_POINT('Ctrl Pts',(77.5525577052348,-6.95369539142955,
41.0360980070918));
#171148=CARTESIAN_POINT('Ctrl Pts',(77.4790197265573,-7.03334720038034,
41.0470987407664));
#171149=CARTESIAN_POINT('Ctrl Pts',(77.3627047132826,-7.15537022968237,
41.0644818265892));
#171150=CARTESIAN_POINT('Ctrl Pts',(77.3207898736863,-7.19856925942343,
41.0707426482386));
#171151=CARTESIAN_POINT('Ctrl Pts',(77.2376487384254,-7.28275170342843,
41.0831509789572));
#171152=CARTESIAN_POINT('Ctrl Pts',(77.1964493257227,-7.32375875748218,
41.089294665291));
#171153=CARTESIAN_POINT('Ctrl Pts',(77.0849042211385,-7.43289809342019,
41.1059190680632));
#171154=CARTESIAN_POINT('Ctrl Pts',(77.0139293706916,-7.50036556454618,
41.1164872961157));
#171155=CARTESIAN_POINT('Ctrl Pts',(76.6864070774697,-7.8028312059972,41.1652458625602));
#171156=CARTESIAN_POINT('Ctrl Pts',(76.4190165354946,-8.02548914234972,
41.2050323975225));
#171157=CARTESIAN_POINT('Ctrl Pts',(75.8366534024342,-8.46191632817427,
41.2922309507865));
#171158=CARTESIAN_POINT('Ctrl Pts',(75.5200232683736,-8.67253465312376,
41.3399444956717));
#171159=CARTESIAN_POINT('Ctrl Pts',(75.0932027642936,-8.92307973147675,
41.4049407542926));
#171160=CARTESIAN_POINT('Ctrl Pts',(74.992869920202,-8.97969578241385,41.4202646474527));
#171161=CARTESIAN_POINT('Ctrl Pts',(74.7424448216935,-9.11542310643498,
41.4586313394939));
#171162=CARTESIAN_POINT('Ctrl Pts',(74.591312786796,-9.19248002066406,41.4818896101064));
#171163=CARTESIAN_POINT('Ctrl Pts',(74.3454482934272,-9.31013546457496,
41.5198996829357));
#171164=CARTESIAN_POINT('Ctrl Pts',(74.2518781354646,-9.35316518107523,
41.5344045342761));
#171165=CARTESIAN_POINT('Ctrl Pts',(74.0695810462862,-9.43363974854203,
41.562738448414));
#171166=CARTESIAN_POINT('Ctrl Pts',(73.9809416416488,-9.47126169519278,
41.5765490803664));
#171167=CARTESIAN_POINT('Ctrl Pts',(73.7653626751441,-9.55913766853745,
41.6102166631081));
#171168=CARTESIAN_POINT('Ctrl Pts',(73.6379291640151,-9.60808632132263,
41.6301836765182));
#171169=CARTESIAN_POINT('Ctrl Pts',(73.073123924773,-9.81195026239119,41.7189444567463));
#171170=CARTESIAN_POINT('Ctrl Pts',(72.6266323311036,-9.93898254185201,
41.7898282484404));
#171171=CARTESIAN_POINT('Ctrl Pts',(71.7919835398247,-10.1150082328428,
41.9228213438546));
#171172=CARTESIAN_POINT('Ctrl Pts',(71.4065734074098,-10.1730658266453,
41.9844078439595));
#171173=CARTESIAN_POINT('Ctrl Pts',(70.8819130618401,-10.221009383761,42.0678801835785));
#171174=CARTESIAN_POINT('Ctrl Pts',(70.744805929142,-10.2306934508472,42.0896588226559));
#171175=CARTESIAN_POINT('Ctrl Pts',(70.5046670019219,-10.2426865429399,
42.1277015338923));
#171176=CARTESIAN_POINT('Ctrl Pts',(70.4017199527197,-10.2462348543771,
42.1439776443847));
#171177=CARTESIAN_POINT('Ctrl Pts',(70.2424081672662,-10.2492634056236,
42.1690983386118));
#171178=CARTESIAN_POINT('Ctrl Pts',(70.1860758048906,-10.2498583874661,
42.1779680568265));
#171179=CARTESIAN_POINT('Ctrl Pts',(70.0784109730032,-10.2500862104176,
42.1948921933579));
#171180=CARTESIAN_POINT('Ctrl Pts',(70.0270811673423,-10.249799880826,42.202948428152));
#171181=CARTESIAN_POINT('Ctrl Pts',(69.8952185046746,-10.2480497692699,
42.2236150272714));
#171182=CARTESIAN_POINT('Ctrl Pts',(69.8146939112116,-10.2460087084472,
42.2362075318369));
#171183=CARTESIAN_POINT('Ctrl Pts',(69.4311997185964,-10.2316554002495,
42.2960661450067));
#171184=CARTESIAN_POINT('Ctrl Pts',(69.1288032560586,-10.2065539130263,
42.3429353815764));
#171185=CARTESIAN_POINT('Ctrl Pts',(68.3448741127029,-10.1054881116976,
42.4641052211933));
#171186=CARTESIAN_POINT('Ctrl Pts',(67.8667957127787,-10.0080528806127,
42.5376930843337));
#171187=CARTESIAN_POINT('Ctrl Pts',(67.210734278808,-9.82373831792741,42.6389832248867));
#171188=CARTESIAN_POINT('Ctrl Pts',(67.0254614860757,-9.76584396775118,
42.6676183412889));
#171189=CARTESIAN_POINT('Ctrl Pts',(66.6914602635536,-9.65074918116083,
42.7193214625833));
#171190=CARTESIAN_POINT('Ctrl Pts',(66.5422011822621,-9.59531431834851,
42.7424566756313));
#171191=CARTESIAN_POINT('Ctrl Pts',(66.3003003397803,-9.4988739277754,42.780003460665));
#171192=CARTESIAN_POINT('Ctrl Pts',(66.206864161016,-9.45997862245632,42.7945190799848));
#171193=CARTESIAN_POINT('Ctrl Pts',(66.0247675191537,-9.38093144995062,
42.8228323310797));
#171194=CARTESIAN_POINT('Ctrl Pts',(65.9360716464283,-9.34089050952548,
42.8366345313369));
#171195=CARTESIAN_POINT('Ctrl Pts',(65.7183198397622,-9.23876254125689,
42.8705441520899));
#171196=CARTESIAN_POINT('Ctrl Pts',(65.5899689257589,-9.17519101207616,
42.8905536483184));
#171197=CARTESIAN_POINT('Ctrl Pts',(65.0019901980299,-8.86819225514824,
42.982285489555));
#171198=CARTESIAN_POINT('Ctrl Pts',(64.5599807279445,-8.5920108761144,43.0514825197807));
#171199=CARTESIAN_POINT('Ctrl Pts',(63.8385401500208,-8.05988720219786,
43.1636036880936));
#171200=CARTESIAN_POINT('Ctrl Pts',(63.548724571481,-7.82022914357439,43.2083693712019));
#171201=CARTESIAN_POINT('Ctrl Pts',(63.2010465706138,-7.49880992345238,
43.2611688632362));
#171202=CARTESIAN_POINT('Ctrl Pts',(63.1304731108674,-7.4316715860082,43.2718352988815));
#171203=CARTESIAN_POINT('Ctrl Pts',(63.019390249814,-7.32293441139376,43.2885280859276));
#171204=CARTESIAN_POINT('Ctrl Pts',(62.9782678448442,-7.28199058140089,
43.2946859857017));
#171205=CARTESIAN_POINT('Ctrl Pts',(62.8951149025589,-7.197781174401,43.3070894314852));
#171206=CARTESIAN_POINT('Ctrl Pts',(62.8531136598361,-7.15448927420012,
43.3133288946496));
#171207=CARTESIAN_POINT('Ctrl Pts',(62.7362667739382,-7.03190687389094,
43.3306194702127));
#171208=CARTESIAN_POINT('Ctrl Pts',(62.6622864964652,-6.95177688158209,
43.3414875602269));
#171209=CARTESIAN_POINT('Ctrl Pts',(62.4916563702286,-6.76094917609823,
43.3663886209964));
#171210=CARTESIAN_POINT('Ctrl Pts',(62.3960632753648,-6.64931087552116,
43.3802091111123));
#171211=CARTESIAN_POINT('Ctrl Pts',(62.0154123502092,-6.18495979641894,
43.4347904284973));
#171212=CARTESIAN_POINT('Ctrl Pts',(61.7512251719933,-5.81534570084265,
43.4716146726948));
#171213=CARTESIAN_POINT('Ctrl Pts',(61.3448960495976,-5.1591306179987,43.5271123087567));
#171214=CARTESIAN_POINT('Ctrl Pts',(61.1901527276195,-4.88130754176526,
43.547879498298));
#171215=CARTESIAN_POINT('Ctrl Pts',(60.9919903885807,-4.48330927718824,
43.5740179079228));
#171216=CARTESIAN_POINT('Ctrl Pts',(60.9376309207981,-4.36890195438882,
43.5811307878231));
#171217=CARTESIAN_POINT('Ctrl Pts',(60.8454328724955,-4.16527582899965,
43.5930913611281));
#171218=CARTESIAN_POINT('Ctrl Pts',(60.806722155446,-4.07647757889274,43.5980774865959));
#171219=CARTESIAN_POINT('Ctrl Pts',(60.7276048238023,-3.8877922035273,43.6081895033886));
#171220=CARTESIAN_POINT('Ctrl Pts',(60.6874990306224,-3.78778913082878,
43.6132678560022));
#171221=CARTESIAN_POINT('Ctrl Pts',(60.5806290917482,-3.50876749973317,
43.626658658446));
#171222=CARTESIAN_POINT('Ctrl Pts',(60.5172424990888,-3.32847745506082,
43.6344346924671));
#171223=CARTESIAN_POINT('Ctrl Pts',(60.2076167799292,-2.36324238070314,
43.671375970447));
#171224=CARTESIAN_POINT('Ctrl Pts',(60.0504624715391,-1.55243489538217,
43.6864193700675));
#171225=CARTESIAN_POINT('Ctrl Pts',(59.9792450557694,-0.582489999898303,
43.6822138483795));
#171226=CARTESIAN_POINT('Ctrl Pts',(59.9715017252469,-0.433189199583286,
43.6809465333485));
#171227=CARTESIAN_POINT('Ctrl Pts',(59.9649354564718,-0.217092509485996,
43.6781744434392));
#171228=CARTESIAN_POINT('Ctrl Pts',(59.9635474472644,-0.150387540702407,
43.6771896383154));
#171229=CARTESIAN_POINT('Ctrl Pts',(59.9624839812393,-0.0557842688263437,
43.6756060404254));
#171230=CARTESIAN_POINT('Ctrl Pts',(59.9622819875824,-0.0278921387390975,
43.675116105672));
#171231=CARTESIAN_POINT('Ctrl Pts',(59.9621915011161,1.31067303586202E-9,
43.6746029314002));
#171232=CARTESIAN_POINT('Ctrl Pts',(59.9459911121981,-7.28640352773959E-10,
43.5827259602593));
#171233=CARTESIAN_POINT('Ctrl Pts',(59.9460375900799,-0.0143266460599373,
43.5829895494194));
#171234=CARTESIAN_POINT('Ctrl Pts',(59.946113810169,-0.0286533381359354,
43.5832488390263));
#171235=CARTESIAN_POINT('Ctrl Pts',(59.9466646997059,-0.103139137788873,
43.5845744266029));
#171236=CARTESIAN_POINT('Ctrl Pts',(59.9476339701448,-0.163294614590786,
43.585568729974));
#171237=CARTESIAN_POINT('Ctrl Pts',(59.9521211302597,-0.344036513006118,
43.588321807074));
#171238=CARTESIAN_POINT('Ctrl Pts',(59.957221110632,-0.464576916028509,
43.5898441921207));
#171239=CARTESIAN_POINT('Ctrl Pts',(59.9952440979856,-1.10044949754627,
43.5961474971593));
#171240=CARTESIAN_POINT('Ctrl Pts',(60.0644986283257,-1.61293018088451,
43.5951938415123));
#171241=CARTESIAN_POINT('Ctrl Pts',(60.2491038566319,-2.48481286991128,
43.5817148185854));
#171242=CARTESIAN_POINT('Ctrl Pts',(60.3464892490603,-2.84703270485521,
43.5724493086601));
#171243=CARTESIAN_POINT('Ctrl Pts',(60.5191319917585,-3.37397908844107,
43.5532653883163));
#171244=CARTESIAN_POINT('Ctrl Pts',(60.5795257731593,-3.543349290979,43.5461983962768));
#171245=CARTESIAN_POINT('Ctrl Pts',(60.6823277489088,-3.80962222417279,
43.5336394321642));
#171246=CARTESIAN_POINT('Ctrl Pts',(60.7218859029594,-3.90761074021264,
43.5286993712111));
#171247=CARTESIAN_POINT('Ctrl Pts',(60.800796383866,-4.09480154908873,43.5186475891421));
#171248=CARTESIAN_POINT('Ctrl Pts',(60.8399245364853,-4.18408823367254,
43.513579128566));
#171249=CARTESIAN_POINT('Ctrl Pts',(60.9356783573457,-4.3944786241219,43.5009853742053));
#171250=CARTESIAN_POINT('Ctrl Pts',(60.9933931351928,-4.51505409487973,
43.4932481998287));
#171251=CARTESIAN_POINT('Ctrl Pts',(61.3342139881777,-5.19309496507027,
43.4467919855794));
#171252=CARTESIAN_POINT('Ctrl Pts',(61.6646959979008,-5.72460664695023,
43.3988158979195));
#171253=CARTESIAN_POINT('Ctrl Pts',(62.1758565580389,-6.40081490004067,
43.3229576775345));
#171254=CARTESIAN_POINT('Ctrl Pts',(62.3165378614139,-6.57478569882454,
43.3019529901831));
#171255=CARTESIAN_POINT('Ctrl Pts',(62.5574355865755,-6.85348034838193,
43.2659333134321));
#171256=CARTESIAN_POINT('Ctrl Pts',(62.6544107220027,-6.96096753278267,
43.2514209122878));
#171257=CARTESIAN_POINT('Ctrl Pts',(62.799353378053,-7.11490539940208,43.2297523322832));
#171258=CARTESIAN_POINT('Ctrl Pts',(62.8455598722524,-7.16302442308203,
43.2228477554537));
#171259=CARTESIAN_POINT('Ctrl Pts',(62.9309109399163,-7.25017857204365,
43.2101047413057));
#171260=CARTESIAN_POINT('Ctrl Pts',(62.9699081272575,-7.2893563376217,43.2042869120689));
#171261=CARTESIAN_POINT('Ctrl Pts',(63.0665960901053,-7.38492314733817,
43.1898717121464));
#171262=CARTESIAN_POINT('Ctrl Pts',(63.1246379911191,-7.44094407153647,
43.1812257756037));
#171263=CARTESIAN_POINT('Ctrl Pts',(63.3731532484376,-7.675167396915,43.1442206188697));
#171264=CARTESIAN_POINT('Ctrl Pts',(63.5697038420368,-7.84664015300446,
43.114984867416));
#171265=CARTESIAN_POINT('Ctrl Pts',(64.1352126644439,-8.30296019081711,
43.0306020645529));
#171266=CARTESIAN_POINT('Ctrl Pts',(64.5172977653965,-8.57011422427541,
42.9732714676007));
#171267=CARTESIAN_POINT('Ctrl Pts',(65.0745654338905,-8.90522790379286,
42.8885664899947));
#171268=CARTESIAN_POINT('Ctrl Pts',(65.2356545641202,-8.99618558198695,
42.8639666151387));
#171269=CARTESIAN_POINT('Ctrl Pts',(65.5336148410308,-9.15381648743382,
42.8182344431816));
#171270=CARTESIAN_POINT('Ctrl Pts',(65.6696924087366,-9.22191951265763,
42.7972643415207));
#171271=CARTESIAN_POINT('Ctrl Pts',(65.8974898533498,-9.32956159898774,
42.7620168084714));
#171272=CARTESIAN_POINT('Ctrl Pts',(65.9883735920149,-9.3708692046486,42.7479174718631));
#171273=CARTESIAN_POINT('Ctrl Pts',(66.1711273838748,-9.45068162080295,
42.7194933426395));
#171274=CARTESIAN_POINT('Ctrl Pts',(66.2629851798873,-9.48918732474518,
42.705170595965));
#171275=CARTESIAN_POINT('Ctrl Pts',(66.4949577457651,-9.58240888751211,
42.6689138259321));
#171276=CARTESIAN_POINT('Ctrl Pts',(66.6357353503896,-9.63535125544396,
42.6468318910217));
#171277=CARTESIAN_POINT('Ctrl Pts',(67.3100766137265,-9.87183714434973,
42.5407200531307));
#171278=CARTESIAN_POINT('Ctrl Pts',(67.8568336237306,-10.0132608371559,
42.4536330517418));
#171279=CARTESIAN_POINT('Ctrl Pts',(68.8275881304431,-10.1786493093381,
42.2987866733099));
#171280=CARTESIAN_POINT('Ctrl Pts',(69.2467769037161,-10.223093001542,42.2318708571912));
#171281=CARTESIAN_POINT('Ctrl Pts',(69.7566209836434,-10.2447623578791,
42.1511825076571));
#171282=CARTESIAN_POINT('Ctrl Pts',(69.8457224560884,-10.2473567790266,
42.1371075889581));
#171283=CARTESIAN_POINT('Ctrl Pts',(69.9883517930055,-10.2496024647024,
42.1146302327215));
#171284=CARTESIAN_POINT('Ctrl Pts',(70.0418599869951,-10.2500156234435,
42.1062096836316));
#171285=CARTESIAN_POINT('Ctrl Pts',(70.149518156792,-10.2499832824638,42.0892946883698));
#171286=CARTESIAN_POINT('Ctrl Pts',(70.2036663937296,-10.2495275185122,
42.0808007840563));
#171287=CARTESIAN_POINT('Ctrl Pts',(70.3500372849288,-10.2471074464185,
42.0578739302752));
#171288=CARTESIAN_POINT('Ctrl Pts',(70.4422449880518,-10.2443076647194,
42.0434668380879));
#171289=CARTESIAN_POINT('Ctrl Pts',(71.022766247079,-10.2186465656209,41.9529479927956));
#171290=CARTESIAN_POINT('Ctrl Pts',(71.5090751876544,-10.1613175233665,
41.8779170190555));
#171291=CARTESIAN_POINT('Ctrl Pts',(72.4346805892153,-9.98283080432906,
41.7351742488077));
#171292=CARTESIAN_POINT('Ctrl Pts',(72.8737854201792,-9.86683159229917,
41.6674861722385));
#171293=CARTESIAN_POINT('Ctrl Pts',(73.4640988682087,-9.66724560127392,
41.5761341899508));
#171294=CARTESIAN_POINT('Ctrl Pts',(73.6231304500029,-9.60895774775429,
41.5514904435393));
#171295=CARTESIAN_POINT('Ctrl Pts',(73.8764955096983,-9.50876261489964,
41.512170585656));
#171296=CARTESIAN_POINT('Ctrl Pts',(73.971772300336,-9.4693801852802,41.4973711659113));
#171297=CARTESIAN_POINT('Ctrl Pts',(74.1557884221983,-9.38998415419588,
41.4687630291964));
#171298=CARTESIAN_POINT('Ctrl Pts',(74.2445848466483,-9.35013427435378,
41.4549468436074));
#171299=CARTESIAN_POINT('Ctrl Pts',(74.4571581255323,-9.25100800216019,
41.4218473526083));
#171300=CARTESIAN_POINT('Ctrl Pts',(74.580338722039,-9.19047211405968,41.4026467156689));
#171301=CARTESIAN_POINT('Ctrl Pts',(75.2248689893672,-8.85721022430065,
41.3021063109763));
#171302=CARTESIAN_POINT('Ctrl Pts',(75.7232208935052,-8.54154437581208,
41.2240334446168));
#171303=CARTESIAN_POINT('Ctrl Pts',(76.3797857300465,-8.04063741825332,
41.1221956496918));
#171304=CARTESIAN_POINT('Ctrl Pts',(76.5627223540064,-7.89069744434567,
41.0939557778104));
#171305=CARTESIAN_POINT('Ctrl Pts',(76.8529490302931,-7.63543627012667,
41.0495539337904));
#171306=CARTESIAN_POINT('Ctrl Pts',(76.9633673714707,-7.53392065665673,
41.0327627421851));
#171307=CARTESIAN_POINT('Ctrl Pts',(77.1202509238951,-7.38318789238706,
41.0091001727908));
#171308=CARTESIAN_POINT('Ctrl Pts',(77.1684938332366,-7.33590959851867,
41.0018515246761));
#171309=CARTESIAN_POINT('Ctrl Pts',(77.2552570340658,-7.24918325001962,
40.9888712799995));
#171310=CARTESIAN_POINT('Ctrl Pts',(77.2939302737214,-7.20989801632789,
40.9831068009904));
#171311=CARTESIAN_POINT('Ctrl Pts',(77.3874447105696,-7.11335930622603,
40.9692187416404));
#171312=CARTESIAN_POINT('Ctrl Pts',(77.4419476727918,-7.05577317682132,
40.9611673409808));
#171313=CARTESIAN_POINT('Ctrl Pts',(77.6587057174443,-6.82137060509613,
40.9293059857636));
#171314=CARTESIAN_POINT('Ctrl Pts',(77.8154820958198,-6.6394385941867,40.9066261575104));
#171315=CARTESIAN_POINT('Ctrl Pts',(78.1833153722474,-6.18102325609108,
40.8540994115583));
#171316=CARTESIAN_POINT('Ctrl Pts',(78.3870793060089,-5.89891689248128,
40.8256083292068));
#171317=CARTESIAN_POINT('Ctrl Pts',(78.7407995616609,-5.35289045722612,
40.7769456644645));
#171318=CARTESIAN_POINT('Ctrl Pts',(78.8941341991853,-5.09165831176914,
40.7561986658561));
#171319=CARTESIAN_POINT('Ctrl Pts',(79.114079668581,-4.67603162253496,40.726895501663));
#171320=CARTESIAN_POINT('Ctrl Pts',(79.1887622655494,-4.52619813869404,
40.7170439350763));
#171321=CARTESIAN_POINT('Ctrl Pts',(79.3035589219681,-4.28112993192916,
40.7020599920552));
#171322=CARTESIAN_POINT('Ctrl Pts',(79.3459375623717,-4.18701268434998,
40.6965679481115));
#171323=CARTESIAN_POINT('Ctrl Pts',(79.4255869180075,-4.00279687151226,
40.6863253375304));
#171324=CARTESIAN_POINT('Ctrl Pts',(79.4630065666425,-3.912776019988,40.6815510433645));
#171325=CARTESIAN_POINT('Ctrl Pts',(79.5510186649322,-3.69229658560822,
40.6704188464459));
#171326=CARTESIAN_POINT('Ctrl Pts',(79.6002509572031,-3.56130564516457,
40.6642765731327));
#171327=CARTESIAN_POINT('Ctrl Pts',(79.8734219276251,-2.78716581397686,
40.630750261085));
#171328=CARTESIAN_POINT('Ctrl Pts',(80.036199019137,-2.12385049578148,40.6130137092608));
#171329=CARTESIAN_POINT('Ctrl Pts',(80.1674515416969,-1.2091924592492,40.6050775418096));
#171330=CARTESIAN_POINT('Ctrl Pts',(80.1935067487899,-0.967989845444839,
40.6045162377913));
#171331=CARTESIAN_POINT('Ctrl Pts',(80.2189222227205,-0.619335059196382,
40.606063448969));
#171332=CARTESIAN_POINT('Ctrl Pts',(80.2250626423124,-0.512455059801902,
40.6068558946787));
#171333=CARTESIAN_POINT('Ctrl Pts',(80.2331722425514,-0.31960774339719,
40.6088780251448));
#171334=CARTESIAN_POINT('Ctrl Pts',(80.2357243293705,-0.233673779241834,
40.6099908389222));
#171335=CARTESIAN_POINT('Ctrl Pts',(80.2381424332421,-0.0944225953100012,
40.6121463084135));
#171336=CARTESIAN_POINT('Ctrl Pts',(80.2386605338121,-0.0411186812615804,
40.6130549964071));
#171337=CARTESIAN_POINT('Ctrl Pts',(80.2388875538814,0.068039035736405,
40.615089812499));
#171338=CARTESIAN_POINT('Ctrl Pts',(80.2385565526446,0.123890759317233,
40.6162240313559));
#171339=CARTESIAN_POINT('Ctrl Pts',(80.2364058055572,0.278197784409159,
40.6196109858607));
#171340=CARTESIAN_POINT('Ctrl Pts',(80.2336427929077,0.37662978697222,40.6220565484951));
#171341=CARTESIAN_POINT('Ctrl Pts',(80.2103218164168,0.928889356995538,
40.6373367883457));
#171342=CARTESIAN_POINT('Ctrl Pts',(80.1615626044225,1.38087278303248,40.6557394214364));
#171343=CARTESIAN_POINT('Ctrl Pts',(80.0199125654128,2.19143526620157,40.6984158437578));
#171344=CARTESIAN_POINT('Ctrl Pts',(79.9370832874237,2.55108783377926,40.7209201867642));
#171345=CARTESIAN_POINT('Ctrl Pts',(79.7881175342793,3.06943055637364,40.75837518173));
#171346=CARTESIAN_POINT('Ctrl Pts',(79.736912265311,3.23227915737716,40.7708918470471));
#171347=CARTESIAN_POINT('Ctrl Pts',(79.634702643799,3.5311982057483,40.7952517888642));
#171348=CARTESIAN_POINT('Ctrl Pts',(79.5848110211136,3.66761744394733,40.8069160276739));
#171349=CARTESIAN_POINT('Ctrl Pts',(79.496038160898,3.89529874403081,40.8273101327712));
#171350=CARTESIAN_POINT('Ctrl Pts',(79.4586850379013,3.98715464255901,40.8357970317134));
#171351=CARTESIAN_POINT('Ctrl Pts',(79.385012852756,4.16107311123714,40.852364021814));
#171352=CARTESIAN_POINT('Ctrl Pts',(79.3489345058583,4.2432311709102,40.8604057255209));
#171353=CARTESIAN_POINT('Ctrl Pts',(79.2502716536176,4.46014513185474,40.8822163440565));
#171354=CARTESIAN_POINT('Ctrl Pts',(79.1858424905868,4.59400837202528,40.8962775208754));
#171355=CARTESIAN_POINT('Ctrl Pts',(78.9381167390807,5.08134239878733,40.9497345341578));
#171356=CARTESIAN_POINT('Ctrl Pts',(78.7373149201773,5.42519801935659,40.9919164317268));
#171357=CARTESIAN_POINT('Ctrl Pts',(78.3217323578381,6.05019069970159,41.077833175774));
#171358=CARTESIAN_POINT('Ctrl Pts',(78.1113059835995,6.33361571499208,41.1208130307063));
#171359=CARTESIAN_POINT('Ctrl Pts',(77.8034569838703,6.70627120459286,41.1834732485849));
#171360=CARTESIAN_POINT('Ctrl Pts',(77.7181519512505,6.80557187567079,41.2008167853645));
#171361=CARTESIAN_POINT('Ctrl Pts',(77.5641791857886,6.97797051420906,41.232122576725));
#171362=CARTESIAN_POINT('Ctrl Pts',(77.4962853560562,7.05176390492606,41.2459272234256));
#171363=CARTESIAN_POINT('Ctrl Pts',(77.3871513568511,7.166917943456,41.2681328440385));
#171364=CARTESIAN_POINT('Ctrl Pts',(77.3466117927354,7.20896209254216,41.2763848102507));
#171365=CARTESIAN_POINT('Ctrl Pts',(77.2694152287003,7.28765533835146,41.2921083239062));
#171366=CARTESIAN_POINT('Ctrl Pts',(77.2328340306705,7.32437933958338,41.2995632703786));
#171367=CARTESIAN_POINT('Ctrl Pts',(77.1280766959687,7.42794721872118,41.3209200009373));
#171368=CARTESIAN_POINT('Ctrl Pts',(77.0592505971471,7.49409711798191,41.3349609988095));
#171369=CARTESIAN_POINT('Ctrl Pts',(76.6173294068665,7.90698117658797,41.4251309402652));
#171370=CARTESIAN_POINT('Ctrl Pts',(76.2199922768251,8.22560935912857,41.5062352773913));
#171371=CARTESIAN_POINT('Ctrl Pts',(75.4832917644561,8.72959773806129,41.6552044139016));
#171372=CARTESIAN_POINT('Ctrl Pts',(75.1538759892047,8.92812337330524,41.7213883313959));
#171373=CARTESIAN_POINT('Ctrl Pts',(74.6875133322545,9.17366615781197,41.814289648415));
#171374=CARTESIAN_POINT('Ctrl Pts',(74.5595694582691,9.237549914246,41.8397002935372));
#171375=CARTESIAN_POINT('Ctrl Pts',(74.3418879498715,9.34044343571355,41.8828027581011));
#171376=CARTESIAN_POINT('Ctrl Pts',(74.2528545331535,9.38093242200543,41.9003960884452));
#171377=CARTESIAN_POINT('Ctrl Pts',(74.0819289368364,9.45564015737336,41.9341041063845));
#171378=CARTESIAN_POINT('Ctrl Pts',(74.000144760869,9.49008927924609,41.9502037038238));
#171379=CARTESIAN_POINT('Ctrl Pts',(73.781501364439,9.57875718641313,41.9931701847553));
#171380=CARTESIAN_POINT('Ctrl Pts',(73.6438965685247,9.63103035949489,42.0201345343597));
#171381=CARTESIAN_POINT('Ctrl Pts',(72.9410820168122,9.88027937791589,42.1575026697587));
#171382=CARTESIAN_POINT('Ctrl Pts',(72.3603789891852,10.028767605135,42.2697834155235));
#171383=CARTESIAN_POINT('Ctrl Pts',(71.502079616051,10.1671413440725,42.4356364628139));
#171384=CARTESIAN_POINT('Ctrl Pts',(71.2323799028694,10.1993012234798,42.4877518500749));
#171385=CARTESIAN_POINT('Ctrl Pts',(70.8487744119882,10.2290971665373,42.5621153328345));
#171386=CARTESIAN_POINT('Ctrl Pts',(70.7356517164443,10.2359292629871,42.584074144077));
#171387=CARTESIAN_POINT('Ctrl Pts',(70.5332716509214,10.2446623340606,42.6234364358077));
#171388=CARTESIAN_POINT('Ctrl Pts',(70.4440540624603,10.2473017608102,42.640815805587));
#171389=CARTESIAN_POINT('Ctrl Pts',(70.3015238058131,10.2495859655522,42.6686344253381));
#171390=CARTESIAN_POINT('Ctrl Pts',(70.2482238541103,10.2500086536731,42.6790494262501));
#171391=CARTESIAN_POINT('Ctrl Pts',(70.1412820663025,10.2499910209053,42.6999735552205));
#171392=CARTESIAN_POINT('Ctrl Pts',(70.0876419906215,10.2495450902793,42.7104824859471));
#171393=CARTESIAN_POINT('Ctrl Pts',(69.9431202514993,10.2471657637742,42.7388299870026));
#171394=CARTESIAN_POINT('Ctrl Pts',(69.852260865597,10.2444143332145,42.7566873966239));
#171395=CARTESIAN_POINT('Ctrl Pts',(69.2578523779148,10.2181930521271,42.8737033210349));
#171396=CARTESIAN_POINT('Ctrl Pts',(68.7567501112307,10.1574351896112,42.9732171057245));
#171397=CARTESIAN_POINT('Ctrl Pts',(67.7885712796517,9.96402834930255,43.16551229296));
#171398=CARTESIAN_POINT('Ctrl Pts',(67.3221959485919,9.83476678771789,43.2581496903659));
#171399=CARTESIAN_POINT('Ctrl Pts',(66.7318003060275,9.62363010938942,43.3750098951206));
#171400=CARTESIAN_POINT('Ctrl Pts',(66.5979465520151,9.57247178701405,43.4014788638174));
#171401=CARTESIAN_POINT('Ctrl Pts',(66.3745381330922,9.48150719916644,43.4456127821913));
#171402=CARTESIAN_POINT('Ctrl Pts',(66.2844032180224,9.44324792314643,43.4634065243943));
#171403=CARTESIAN_POINT('Ctrl Pts',(66.1137386736809,9.36781801758265,43.4970758814441));
#171404=CARTESIAN_POINT('Ctrl Pts',(66.0331157095046,9.33089108775091,43.5129720104634));
#171405=CARTESIAN_POINT('Ctrl Pts',(65.8202489540236,9.22993809552489,43.5549199188208));
#171406=CARTESIAN_POINT('Ctrl Pts',(65.6888786706006,9.16404454290439,43.5807846723764));
#171407=CARTESIAN_POINT('Ctrl Pts',(65.2085602447716,8.90970766782227,43.675296153065));
#171408=CARTESIAN_POINT('Ctrl Pts',(64.8691603666153,8.70329799202075,43.7419543654796));
#171409=CARTESIAN_POINT('Ctrl Pts',(64.1985032119731,8.23877372854175,43.8740335738653));
#171410=CARTESIAN_POINT('Ctrl Pts',(63.8693083531321,7.97893375500673,43.9390700456032));
#171411=CARTESIAN_POINT('Ctrl Pts',(63.4548230651222,7.60752724362429,44.0219980900755));
#171412=CARTESIAN_POINT('Ctrl Pts',(63.3545087620615,7.51387866073428,44.0421584804766));
#171413=CARTESIAN_POINT('Ctrl Pts',(63.2093224476735,7.37268393367582,44.0715075251689));
#171414=CARTESIAN_POINT('Ctrl Pts',(63.1629719911126,7.32672431201815,44.0809038283794));
#171415=CARTESIAN_POINT('Ctrl Pts',(63.0781916190838,7.24101109611234,44.0981454549373));
#171416=CARTESIAN_POINT('Ctrl Pts',(63.0396383023116,7.2013875802826,44.1060078610015));
#171417=CARTESIAN_POINT('Ctrl Pts',(62.9444561668407,7.10194209022563,44.1254717352569));
#171418=CARTESIAN_POINT('Ctrl Pts',(62.8882245884188,7.04173459229395,44.1370176684737));
#171419=CARTESIAN_POINT('Ctrl Pts',(62.6389037039307,6.76815901836654,44.1884040771738));
#171420=CARTESIAN_POINT('Ctrl Pts',(62.4541192736215,6.5471721156624,44.2270191408352));
#171421=CARTESIAN_POINT('Ctrl Pts',(62.0101297946349,5.96786206652741,44.3207776041163));
#171422=CARTESIAN_POINT('Ctrl Pts',(61.7642248934756,5.59973148773273,44.3736457813584));
#171423=CARTESIAN_POINT('Ctrl Pts',(61.4517708519255,5.05926852203045,44.4417054306874));
#171424=CARTESIAN_POINT('Ctrl Pts',(61.3650571102148,4.89965697625828,44.4607139226006));
#171425=CARTESIAN_POINT('Ctrl Pts',(61.2142568371581,4.6036621360204,44.4939773213363));
#171426=CARTESIAN_POINT('Ctrl Pts',(61.1488601915217,4.46803248006192,44.5084840868057));
#171427=CARTESIAN_POINT('Ctrl Pts',(61.0449929553346,4.23998572462094,44.531661998768));
#171428=CARTESIAN_POINT('Ctrl Pts',(61.004866833588,4.14838192684605,44.5406543052984));
#171429=CARTESIAN_POINT('Ctrl Pts',(60.9270231008684,3.96341078168895,44.5581787743077));
#171430=CARTESIAN_POINT('Ctrl Pts',(60.8893267034365,3.87004614627509,44.5667066831668));
#171431=CARTESIAN_POINT('Ctrl Pts',(60.7974910126167,3.6326660703553,44.5875938759801));
#171432=CARTESIAN_POINT('Ctrl Pts',(60.7451781959886,3.48794028136869,44.599598575301));
#171433=CARTESIAN_POINT('Ctrl Pts',(60.5279615902703,2.84235242295893,44.6499801348749));
#171434=CARTESIAN_POINT('Ctrl Pts',(60.3980370108493,2.33005966651555,44.6815814004138));
#171435=CARTESIAN_POINT('Ctrl Pts',(60.252064560178,1.49022692120604,44.7212881957219));
#171436=CARTESIAN_POINT('Ctrl Pts',(60.2115056883058,1.16814721753628,44.7337442901996));
#171437=CARTESIAN_POINT('Ctrl Pts',(60.1718904704918,0.663491986028091,
44.7493674512558));
#171438=CARTESIAN_POINT('Ctrl Pts',(60.1624315563092,0.48200272453448,44.7542083558063));
#171439=CARTESIAN_POINT('Ctrl Pts',(60.1559568484478,0.230712323472897,
44.7599097471535));
#171440=CARTESIAN_POINT('Ctrl Pts',(60.1548649575305,0.161064386341852,
44.7613837534939));
#171441=CARTESIAN_POINT('Ctrl Pts',(60.1543057576669,0.0609395441185803,
44.763354614216));
#171442=CARTESIAN_POINT('Ctrl Pts',(60.1542700764961,0.0304698290536312,
44.7639346639111));
#171443=CARTESIAN_POINT('Ctrl Pts',(60.1543689253998,-1.15483570402281E-9,
44.7644952638818));
#171444=CARTESIAN_POINT('Origin',(69.7358040552328,0.,40.0761166693274));
#171445=CARTESIAN_POINT('',(60.3789471275204,6.59340593767212E-11,46.0381415386512));
#171446=CARTESIAN_POINT('',(60.3627467385963,-5.75426767521213E-14,45.9462645674752));
#171447=CARTESIAN_POINT('',(59.6415245868576,-1.25526296912604E-15,41.8560104904131));
#171448=CARTESIAN_POINT('Ctrl Pts',(60.3789471275204,1.31869374016412E-10,
46.0381415386512));
#171449=CARTESIAN_POINT('Ctrl Pts',(60.378925330733,0.00671878418599705,
46.0380179229264));
#171450=CARTESIAN_POINT('Ctrl Pts',(60.3789100041966,0.0134375803992449,
46.03789295849));
#171451=CARTESIAN_POINT('Ctrl Pts',(60.3788262141627,0.0770085414268258,
46.0366978518554));
#171452=CARTESIAN_POINT('Ctrl Pts',(60.3792145896087,0.133858539604107,
46.0355327241613));
#171453=CARTESIAN_POINT('Ctrl Pts',(60.3816162978435,0.294110881741993,
46.0319808432064));
#171454=CARTESIAN_POINT('Ctrl Pts',(60.3847000954561,0.397485575382497,
46.0293755110242));
#171455=CARTESIAN_POINT('Ctrl Pts',(60.3954619430938,0.6382170946337,46.0225960466755));
#171456=CARTESIAN_POINT('Ctrl Pts',(60.4043200761219,0.775495110568486,
46.0181887322636));
#171457=CARTESIAN_POINT('Ctrl Pts',(60.448292680914,1.29632651977757,45.9994785111034));
#171458=CARTESIAN_POINT('Ctrl Pts',(60.5019329936339,1.67787306614414,45.9816710352204));
#171459=CARTESIAN_POINT('Ctrl Pts',(60.6620634989202,2.48730663859187,45.9357303979089));
#171460=CARTESIAN_POINT('Ctrl Pts',(60.7748970488261,2.91310231641818,45.90653366641));
#171461=CARTESIAN_POINT('Ctrl Pts',(60.9639494315895,3.47799654954706,45.861190457982));
#171462=CARTESIAN_POINT('Ctrl Pts',(61.0167828669662,3.62471447983636,45.8487843676519));
#171463=CARTESIAN_POINT('Ctrl Pts',(61.1093058311519,3.86442905708134,45.8274710075018));
#171464=CARTESIAN_POINT('Ctrl Pts',(61.1470804203344,3.95816360141092,45.8188682644958));
#171465=CARTESIAN_POINT('Ctrl Pts',(61.2248439682433,4.1432143670693,45.8013463007918));
#171466=CARTESIAN_POINT('Ctrl Pts',(61.2647925358388,4.23453613561547,45.7924337659594));
#171467=CARTESIAN_POINT('Ctrl Pts',(61.3676281751315,4.46060148906893,45.7697012294424));
#171468=CARTESIAN_POINT('Ctrl Pts',(61.432115085293,4.59456594006168,45.7556278819492));
#171469=CARTESIAN_POINT('Ctrl Pts',(61.6895592808755,5.10092843623557,45.7000757073256));
#171470=CARTESIAN_POINT('Ctrl Pts',(61.9022396526794,5.46247757645872,45.6554597151197));
#171471=CARTESIAN_POINT('Ctrl Pts',(62.4053327784477,6.2088495327472,45.5516080363524));
#171472=CARTESIAN_POINT('Ctrl Pts',(62.7019803653381,6.58808203293475,45.4913166879943));
#171473=CARTESIAN_POINT('Ctrl Pts',(63.0844067574181,7.0116001530841,45.4135588062441));
#171474=CARTESIAN_POINT('Ctrl Pts',(63.1458917128634,7.07789312758018,45.4010554448187));
#171475=CARTESIAN_POINT('Ctrl Pts',(63.2434072577435,7.18026312697839,45.3812113500679));
#171476=CARTESIAN_POINT('Ctrl Pts',(63.2788518431567,7.2169160438872,45.3739957362542));
#171477=CARTESIAN_POINT('Ctrl Pts',(63.3564123569383,7.29592258117983,45.3581976830808));
#171478=CARTESIAN_POINT('Ctrl Pts',(63.398626813907,7.33817229649872,45.3495938420671));
#171479=CARTESIAN_POINT('Ctrl Pts',(63.5174571149938,7.4550211050397,45.3253650037492));
#171480=CARTESIAN_POINT('Ctrl Pts',(63.5948656056335,7.5287678368704,45.3095708072905));
#171481=CARTESIAN_POINT('Ctrl Pts',(63.7785695622404,7.69831509588369,45.2720858636952));
#171482=CARTESIAN_POINT('Ctrl Pts',(63.8857392206877,7.79309526280672,45.2502159904983));
#171483=CARTESIAN_POINT('Ctrl Pts',(64.3223182430656,8.16297009745149,45.1612032877917));
#171484=CARTESIAN_POINT('Ctrl Pts',(64.6667790051496,8.41889901779289,45.0911652196799));
#171485=CARTESIAN_POINT('Ctrl Pts',(65.0571008875175,8.67177745263827,45.0124694009763));
#171486=CARTESIAN_POINT('Ctrl Pts',(65.0880919473385,8.69161382469961,45.0062252464144));
#171487=CARTESIAN_POINT('Ctrl Pts',(65.3784028575049,8.87518222957974,44.947773431553));
#171488=CARTESIAN_POINT('Ctrl Pts',(65.64485274034,9.02697212853524,44.8944340943857));
#171489=CARTESIAN_POINT('Ctrl Pts',(66.0278319447423,9.22234577828469,44.8182809434756));
#171490=CARTESIAN_POINT('Ctrl Pts',(66.1389521851639,9.27645011243593,44.7962426803298));
#171491=CARTESIAN_POINT('Ctrl Pts',(66.3374874012046,9.36858307229529,44.7569697563452));
#171492=CARTESIAN_POINT('Ctrl Pts',(66.4245047088404,9.40745464770424,44.7397905606299));
#171493=CARTESIAN_POINT('Ctrl Pts',(66.6101971756299,9.48722343313728,44.7032013747657));
#171494=CARTESIAN_POINT('Ctrl Pts',(66.7089973473114,9.52779175354907,44.6837752751633));
#171495=CARTESIAN_POINT('Ctrl Pts',(66.9870644186293,9.63676335449365,44.629212788059));
#171496=CARTESIAN_POINT('Ctrl Pts',(67.1676578649076,9.70156431617021,44.5939047391021));
#171497=CARTESIAN_POINT('Ctrl Pts',(67.5914784360616,9.83991033498591,44.5112939379681));
#171498=CARTESIAN_POINT('Ctrl Pts',(67.8358538125961,9.90941510406354,44.4638492042291));
#171499=CARTESIAN_POINT('Ctrl Pts',(68.4110612650839,10.0493690707769,44.3524360082622));
#171500=CARTESIAN_POINT('Ctrl Pts',(68.7433312152032,10.1124040850863,44.288277909562));
#171501=CARTESIAN_POINT('Ctrl Pts',(69.3993086443484,10.2023622571703,44.1614856735944));
#171502=CARTESIAN_POINT('Ctrl Pts',(69.7224336102066,10.2305863885849,44.0989673307257));
#171503=CARTESIAN_POINT('Ctrl Pts',(70.1267142570285,10.2459391287521,44.0202884472602));
#171504=CARTESIAN_POINT('Ctrl Pts',(70.2071940450906,10.2480107407359,44.0046030102669));
#171505=CARTESIAN_POINT('Ctrl Pts',(70.3387607935062,10.2497885692975,43.9789148654675));
#171506=CARTESIAN_POINT('Ctrl Pts',(70.3898397882226,10.2500825110509,43.9689304457918));
#171507=CARTESIAN_POINT('Ctrl Pts',(70.4967202203022,10.2498683828308,43.9480121670586));
#171508=CARTESIAN_POINT('Ctrl Pts',(70.5525190016502,10.2492835853794,43.9370766897919));
#171509=CARTESIAN_POINT('Ctrl Pts',(70.7098017635962,10.2463015868333,43.9062151002667));
#171510=CARTESIAN_POINT('Ctrl Pts',(70.8112534132081,10.2428122278487,43.8862648617424));
#171511=CARTESIAN_POINT('Ctrl Pts',(71.047492832534,10.2310366352245,43.8397276179595));
#171512=CARTESIAN_POINT('Ctrl Pts',(71.1821986972139,10.2215477550215,43.8131299529958));
#171513=CARTESIAN_POINT('Ctrl Pts',(71.6932438072268,10.174994197067,43.7120622472136));
#171514=CARTESIAN_POINT('Ctrl Pts',(72.0675660000018,10.1190765654494,43.6377099036488));
#171515=CARTESIAN_POINT('Ctrl Pts',(72.8616746715027,9.95340129435716,43.4799818104551));
#171516=CARTESIAN_POINT('Ctrl Pts',(73.2794109686977,9.83721198043801,43.3970224981221));
#171517=CARTESIAN_POINT('Ctrl Pts',(73.8336696704474,9.64315796272915,43.2872835621363));
#171518=CARTESIAN_POINT('Ctrl Pts',(73.977630182317,9.58897289097414,43.2588093095473));
#171519=CARTESIAN_POINT('Ctrl Pts',(74.212848065994,9.49415453236284,43.212334985081));
#171520=CARTESIAN_POINT('Ctrl Pts',(74.3048264595144,9.45545997342302,43.1941746489131));
#171521=CARTESIAN_POINT('Ctrl Pts',(74.4864143138544,9.37583517147386,43.158345658732));
#171522=CARTESIAN_POINT('Ctrl Pts',(74.5760291630246,9.33494586695202,43.1406756184265));
#171523=CARTESIAN_POINT('Ctrl Pts',(74.7978734570424,9.22972506855056,43.0969586451437));
#171524=CARTESIAN_POINT('Ctrl Pts',(74.9293405211179,9.16377404830954,43.0710748893434));
#171525=CARTESIAN_POINT('Ctrl Pts',(75.4262731441858,8.90059447464323,42.9732944433866));
#171526=CARTESIAN_POINT('Ctrl Pts',(75.7811128544655,8.68339770983549,42.9036119242478));
#171527=CARTESIAN_POINT('Ctrl Pts',(76.5135561745785,8.16991404432632,42.7593196181868));
#171528=CARTESIAN_POINT('Ctrl Pts',(76.8856618724111,7.8673037180736,42.6857229689564));
#171529=CARTESIAN_POINT('Ctrl Pts',(77.3009799864684,7.47718472773244,42.6021653891796));
#171530=CARTESIAN_POINT('Ctrl Pts',(77.3659816192516,7.41446268098955,42.5890419426571));
#171531=CARTESIAN_POINT('Ctrl Pts',(77.4663433017434,7.3149827254597,42.5686959970545));
#171532=CARTESIAN_POINT('Ctrl Pts',(77.5022742208761,7.27882364475396,42.5613946294845));
#171533=CARTESIAN_POINT('Ctrl Pts',(77.5797175807923,7.19969814631131,42.5456172336984));
#171534=CARTESIAN_POINT('Ctrl Pts',(77.6211270061647,7.1566309804866,42.5371553414755));
#171535=CARTESIAN_POINT('Ctrl Pts',(77.7356404153824,7.03539868506445,42.513687687667));
#171536=CARTESIAN_POINT('Ctrl Pts',(77.8078999535786,6.9564235699023,42.4988013904465));
#171537=CARTESIAN_POINT('Ctrl Pts',(77.9740004579499,6.7690012970359,42.4644204104341));
#171538=CARTESIAN_POINT('Ctrl Pts',(78.0668322931986,6.65966212288598,42.4450786823118));
#171539=CARTESIAN_POINT('Ctrl Pts',(78.429030297644,6.21425882325532,42.3691813599199));
#171540=CARTESIAN_POINT('Ctrl Pts',(78.6794806304577,5.86286921127467,42.315719866957));
#171541=CARTESIAN_POINT('Ctrl Pts',(78.9268291409886,5.46481180979472,42.2622341112299));
#171542=CARTESIAN_POINT('Ctrl Pts',(78.946230835509,5.43320728767722,42.2580334744581));
#171543=CARTESIAN_POINT('Ctrl Pts',(79.1257685198872,5.13715680139019,42.2191139680423));
#171544=CARTESIAN_POINT('Ctrl Pts',(79.2741652723773,4.8654926123219,42.1865905829128));
#171545=CARTESIAN_POINT('Ctrl Pts',(79.4650960376256,4.47510786674353,42.1443007534294));
#171546=CARTESIAN_POINT('Ctrl Pts',(79.5179603256464,4.36184888822867,42.1325345864788));
#171547=CARTESIAN_POINT('Ctrl Pts',(79.6079640825577,4.15951019654728,42.1123986869945));
#171548=CARTESIAN_POINT('Ctrl Pts',(79.6459311887863,4.070831741312,42.1038683651965));
#171549=CARTESIAN_POINT('Ctrl Pts',(79.7238303008384,3.88160671489311,42.0862860561136));
#171550=CARTESIAN_POINT('Ctrl Pts',(79.763439428332,3.78093423302513,42.0772969346177));
#171551=CARTESIAN_POINT('Ctrl Pts',(79.8698095191329,3.49761694886707,42.0530092576846));
#171552=CARTESIAN_POINT('Ctrl Pts',(79.9330335353391,3.31363594446031,42.0383966059595));
#171553=CARTESIAN_POINT('Ctrl Pts',(80.0679302422039,2.88190894499843,42.0067308774697));
#171554=CARTESIAN_POINT('Ctrl Pts',(80.1356343696011,2.63300748796762,41.9904380516688));
#171555=CARTESIAN_POINT('Ctrl Pts',(80.2717539694384,2.04719203069956,41.9564478910252));
#171556=CARTESIAN_POINT('Ctrl Pts',(80.3328788241228,1.70882907080785,41.940099988337));
#171557=CARTESIAN_POINT('Ctrl Pts',(80.4195677198545,1.04080017210136,41.9136886806186));
#171558=CARTESIAN_POINT('Ctrl Pts',(80.4464152069194,0.711728004257093,
41.9034120510381));
#171559=CARTESIAN_POINT('Ctrl Pts',(80.4602703761031,0.299926844175113,
41.8935757132368));
#171560=CARTESIAN_POINT('Ctrl Pts',(80.4620549104904,0.21794597738313,41.8917663727201));
#171561=CARTESIAN_POINT('Ctrl Pts',(80.4633800212526,0.0839173239754168,
41.8890433426507));
#171562=CARTESIAN_POINT('Ctrl Pts',(80.4635022811982,0.031880557681116,
41.8880439701639));
#171563=CARTESIAN_POINT('Ctrl Pts',(80.4629370090956,-0.0770085414591912,
41.8860712680392));
#171564=CARTESIAN_POINT('Ctrl Pts',(80.4621735584137,-0.133858539639717,
41.8851092383684));
#171565=CARTESIAN_POINT('Ctrl Pts',(80.4587018760738,-0.294110881801409,
41.8825929946396));
#171566=CARTESIAN_POINT('Ctrl Pts',(80.4549129781255,-0.397485575460832,
41.8811995041147));
#171567=CARTESIAN_POINT('Ctrl Pts',(80.4424814359409,-0.638217094768553,
41.8785096601645));
#171568=CARTESIAN_POINT('Ctrl Pts',(80.432650123389,-0.775495110739907,
41.8773977992621));
#171569=CARTESIAN_POINT('Ctrl Pts',(80.3849301185938,-1.29632652018824,
41.8748554590984));
#171570=CARTESIAN_POINT('Ctrl Pts',(80.3284341970514,-1.67787306675583,
41.8764679728648));
#171571=CARTESIAN_POINT('Ctrl Pts',(80.1622481194629,-2.48730663912413,
41.8880657533685));
#171572=CARTESIAN_POINT('Ctrl Pts',(80.0462333950024,-2.91310231668167,
41.899221147135));
#171573=CARTESIAN_POINT('Ctrl Pts',(79.8530739754205,-3.47799654955143,
41.9212721918112));
#171574=CARTESIAN_POINT('Ctrl Pts',(79.7991836532735,-3.62471447984029,
41.9276843794151));
#171575=CARTESIAN_POINT('Ctrl Pts',(79.7049509080823,-3.86442905708363,
41.9393010896296));
#171576=CARTESIAN_POINT('Ctrl Pts',(79.6665120939782,-3.95816360141368,
41.9441368259146));
#171577=CARTESIAN_POINT('Ctrl Pts',(79.5874453973038,-4.14321436707407,
41.9542682657217));
#171578=CARTESIAN_POINT('Ctrl Pts',(79.5468577566825,-4.23453613561992,
41.9595564373218));
#171579=CARTESIAN_POINT('Ctrl Pts',(79.4424488798874,-4.46060148907393,
41.973366700595));
#171580=CARTESIAN_POINT('Ctrl Pts',(79.377037637944,-4.59456594006752,41.982197902062));
#171581=CARTESIAN_POINT('Ctrl Pts',(79.116119264361,-5.10092843624674,42.0180470341715));
#171582=CARTESIAN_POINT('Ctrl Pts',(78.9010055203383,-5.46247757647484,
42.0488626867741));
#171583=CARTESIAN_POINT('Ctrl Pts',(78.3927332564295,-6.20884953275891,
42.1233420135616));
#171584=CARTESIAN_POINT('Ctrl Pts',(78.0933548524537,-6.58808203293845,
42.1681461285969));
#171585=CARTESIAN_POINT('Ctrl Pts',(77.7073968319673,-7.01160015308173,
42.225875150338));
#171586=CARTESIAN_POINT('Ctrl Pts',(77.645343471579,-7.07789312757804,42.2351549271454));
#171587=CARTESIAN_POINT('Ctrl Pts',(77.5469217535134,-7.1802631269752,42.2498598583782));
#171588=CARTESIAN_POINT('Ctrl Pts',(77.5111468528833,-7.2169160438839,42.2552021615061));
#171589=CARTESIAN_POINT('Ctrl Pts',(77.4328605580079,-7.29592258117641,
42.2668841055561));
#171590=CARTESIAN_POINT('Ctrl Pts',(77.3902492573673,-7.3381722964953,42.273237334268));
#171591=CARTESIAN_POINT('Ctrl Pts',(77.2702985495597,-7.45502110503297,
42.2911120302992));
#171592=CARTESIAN_POINT('Ctrl Pts',(77.1921564287853,-7.52876783686154,
42.3027456034984));
#171593=CARTESIAN_POINT('Ctrl Pts',(77.0067105705779,-7.69831509586957,
42.3303517321786));
#171594=CARTESIAN_POINT('Ctrl Pts',(76.8985240962022,-7.79309526278899,
42.3464549556596));
#171595=CARTESIAN_POINT('Ctrl Pts',(76.4578298731816,-8.16297009740647,
42.4121291955713));
#171596=CARTESIAN_POINT('Ctrl Pts',(76.110188206841,-8.41889901772776,42.4641274590054));
#171597=CARTESIAN_POINT('Ctrl Pts',(75.7164900589895,-8.67177745262435,
42.5236755250436));
#171598=CARTESIAN_POINT('Ctrl Pts',(75.6852323620228,-8.69161382475175,
42.5284075058163));
#171599=CARTESIAN_POINT('Ctrl Pts',(75.3924376438511,-8.87518222965952,
42.5727729458325));
#171600=CARTESIAN_POINT('Ctrl Pts',(75.1238135274487,-9.02697212858223,
42.6137815914077));
#171601=CARTESIAN_POINT('Ctrl Pts',(74.7378848836248,-9.2223457783011,42.6732076398196));
#171602=CARTESIAN_POINT('Ctrl Pts',(74.6259284837652,-9.2764501124498,42.6905038071214));
#171603=CARTESIAN_POINT('Ctrl Pts',(74.4259342752012,-9.36858307230592,
42.7215023733009));
#171604=CARTESIAN_POINT('Ctrl Pts',(74.3382891223546,-9.40745464771453,
42.7351208818856));
#171605=CARTESIAN_POINT('Ctrl Pts',(74.1512810429809,-9.48722343314812,
42.7642488580347));
#171606=CARTESIAN_POINT('Ctrl Pts',(74.0517951333466,-9.5277917535606,42.7797859444671));
#171607=CARTESIAN_POINT('Ctrl Pts',(73.7718360886688,-9.63676335451079,
42.8236185175525));
#171608=CARTESIAN_POINT('Ctrl Pts',(73.5900576958591,-9.70156431619152,
42.8522064008754));
#171609=CARTESIAN_POINT('Ctrl Pts',(73.1635420745201,-9.83991033501786,
42.9195328131501));
#171610=CARTESIAN_POINT('Ctrl Pts',(72.9176772818257,-9.90941510410055,
42.9585306482728));
#171611=CARTESIAN_POINT('Ctrl Pts',(72.3390535260209,-10.0493690708103,
43.0505690255109));
#171612=CARTESIAN_POINT('Ctrl Pts',(72.0048785436739,-10.1124040851137,
43.103923149561));
#171613=CARTESIAN_POINT('Ctrl Pts',(71.3450958954378,-10.2023622571799,
43.2091349153755));
#171614=CARTESIAN_POINT('Ctrl Pts',(71.0200752168912,-10.2305863885873,
43.2609021370449));
#171615=CARTESIAN_POINT('Ctrl Pts',(70.6132659133987,-10.2459391287523,
43.3252402956022));
#171616=CARTESIAN_POINT('Ctrl Pts',(70.5322749150267,-10.248010740736,43.3380265148535));
#171617=CARTESIAN_POINT('Ctrl Pts',(70.3998567494346,-10.2497885692975,
43.3588860328936));
#171618=CARTESIAN_POINT('Ctrl Pts',(70.3484433223744,-10.2500825110509,
43.3669737924953));
#171619=CARTESIAN_POINT('Ctrl Pts',(70.240854096352,-10.2498683828307,43.3838723010288));
#171620=CARTESIAN_POINT('Ctrl Pts',(70.1846802397678,-10.2492835853794,
43.3926806209306));
#171621=CARTESIAN_POINT('Ctrl Pts',(70.0263275037152,-10.2463015868331,
43.4174740857719));
#171622=CARTESIAN_POINT('Ctrl Pts',(69.9241707537666,-10.2428122278484,
43.4334255015889));
#171623=CARTESIAN_POINT('Ctrl Pts',(69.6862616398917,-10.2310366352235,
43.4704934370725));
#171624=CARTESIAN_POINT('Ctrl Pts',(69.5505825956879,-10.2215477550199,
43.4915719267213));
#171625=CARTESIAN_POINT('Ctrl Pts',(69.0357900856737,-10.1749941970615,
43.571387071175));
#171626=CARTESIAN_POINT('Ctrl Pts',(68.6586122840996,-10.1190765654379,
43.6295444526155));
#171627=CARTESIAN_POINT('Ctrl Pts',(67.858448040357,-9.95340129433929,43.7529296889922));
#171628=CARTESIAN_POINT('Ctrl Pts',(67.4375305685867,-9.83721198042683,
43.8178476636013));
#171629=CARTESIAN_POINT('Ctrl Pts',(66.8791648299632,-9.64315796272882,
43.9042944358496));
#171630=CARTESIAN_POINT('Ctrl Pts',(66.7341474313231,-9.58897289097375,
43.9267747857123));
#171631=CARTESIAN_POINT('Ctrl Pts',(66.4972197666391,-9.49415453236207,
43.9635524602433));
#171632=CARTESIAN_POINT('Ctrl Pts',(66.4045771481974,-9.45545997342227,
43.9779457896901));
#171633=CARTESIAN_POINT('Ctrl Pts',(66.221686145093,-9.37583517147317,44.0063842559742));
#171634=CARTESIAN_POINT('Ctrl Pts',(66.131432222897,-9.33494586695127,44.0204299330474));
#171635=CARTESIAN_POINT('Ctrl Pts',(65.9080146913774,-9.22972506854991,
44.0552246330863));
#171636=CARTESIAN_POINT('Ctrl Pts',(65.775623295521,-9.16377404830908,44.0758662428602));
#171637=CARTESIAN_POINT('Ctrl Pts',(65.2752164944573,-8.90059447464353,
44.1539436463021));
#171638=CARTESIAN_POINT('Ctrl Pts',(64.9179434119637,-8.68339770983664,
44.2098258258369));
#171639=CARTESIAN_POINT('Ctrl Pts',(64.1803209537105,-8.16991404432835,
44.324745779918));
#171640=CARTESIAN_POINT('Ctrl Pts',(63.8054844387862,-7.86730371807531,
44.3828551958267));
#171641=CARTESIAN_POINT('Ctrl Pts',(63.3866346963149,-7.47718472773274,
44.4463839155955));
#171642=CARTESIAN_POINT('Ctrl Pts',(63.3210646585895,-7.4144626809903,44.4562837774999));
#171643=CARTESIAN_POINT('Ctrl Pts',(63.2197968029131,-7.3149827254624,44.4714905595842));
#171644=CARTESIAN_POINT('Ctrl Pts',(63.1835355685625,-7.27882364475602,
44.4769186164687));
#171645=CARTESIAN_POINT('Ctrl Pts',(63.1053664275514,-7.19969814631249,
44.4885799031316));
#171646=CARTESIAN_POINT('Ctrl Pts',(63.0635601585069,-7.15663098048755,
44.4947911830527));
#171647=CARTESIAN_POINT('Ctrl Pts',(62.9479263425654,-7.03539868506595,
44.5119046945751));
#171648=CARTESIAN_POINT('Ctrl Pts',(62.8749331742322,-6.95642356990395,
44.5226303685366));
#171649=CARTESIAN_POINT('Ctrl Pts',(62.7070907682543,-6.7690012970378,44.547132533635));
#171650=CARTESIAN_POINT('Ctrl Pts',(62.6132421170728,-6.65966212288828,
44.5607076120422));
#171651=CARTESIAN_POINT('Ctrl Pts',(62.2469289119509,-6.21425882325954,
44.6132664716456));
#171652=CARTESIAN_POINT('Ctrl Pts',(61.9932976748477,-5.86286921128045,
44.6486881599369));
#171653=CARTESIAN_POINT('Ctrl Pts',(61.7425728988971,-5.46481180979694,
44.6830261629865));
#171654=CARTESIAN_POINT('Ctrl Pts',(61.722904567331,-5.43320728767347,44.6857146259506));
#171655=CARTESIAN_POINT('Ctrl Pts',(61.5408830750034,-5.13715680138255,
44.7105477575107));
#171656=CARTESIAN_POINT('Ctrl Pts',(61.3903120888982,-4.86549261231695,
44.7307404510571));
#171657=CARTESIAN_POINT('Ctrl Pts',(61.1964318841738,-4.47510786674152,
44.7563031780524));
#171658=CARTESIAN_POINT('Ctrl Pts',(61.1427314367107,-4.36184888822653,
44.7633272491598));
#171659=CARTESIAN_POINT('Ctrl Pts',(61.0512686872711,-4.15951019654608,
44.77518879084));
#171660=CARTESIAN_POINT('Ctrl Pts',(61.0126737358313,-4.0708317413104,44.7801584255075));
#171661=CARTESIAN_POINT('Ctrl Pts',(60.9334590111974,-3.88160671489095,
44.7902795248749));
#171662=CARTESIAN_POINT('Ctrl Pts',(60.8931641457534,-3.78093423302279,
44.7953796332002));
#171663=CARTESIAN_POINT('Ctrl Pts',(60.7849020816094,-3.49761694886339,
44.8089373961114));
#171664=CARTESIAN_POINT('Ctrl Pts',(60.7204931188863,-3.31363594445542,
44.8168298821998));
#171665=CARTESIAN_POINT('Ctrl Pts',(60.58290136188,-2.88190894499112,44.8332112218223));
#171666=CARTESIAN_POINT('Ctrl Pts',(60.513707818352,-2.63300748795805,44.8410571490016));
#171667=CARTESIAN_POINT('Ctrl Pts',(60.3283602700609,-1.85486038514426,
44.8604709180007));
#171668=CARTESIAN_POINT('Ctrl Pts',(60.2442547230065,-1.3188352359329,44.8666826188784));
#171669=CARTESIAN_POINT('Ctrl Pts',(60.1898644273114,-0.621316886541912,
44.864268571302));
#171670=CARTESIAN_POINT('Ctrl Pts',(60.1811636672246,-0.463675701607057,
44.8630346952966));
#171671=CARTESIAN_POINT('Ctrl Pts',(60.1741655665948,-0.248381985595741,
44.8603650018948));
#171672=CARTESIAN_POINT('Ctrl Pts',(60.1727707935746,-0.190844644938373,
44.8595556628521));
#171673=CARTESIAN_POINT('Ctrl Pts',(60.1711405545296,-0.088864956530352,
44.8579482502389));
#171674=CARTESIAN_POINT('Ctrl Pts',(60.1707134643357,-0.0444365562647033,
44.8571898040892));
#171675=CARTESIAN_POINT('Ctrl Pts',(60.1705693073443,2.15049072447686E-6,
44.8563721954731));
#171676=CARTESIAN_POINT('Ctrl Pts',(60.1543689253998,-1.15483570402281E-9,
44.7644952638818));
#171677=CARTESIAN_POINT('Ctrl Pts',(60.1544335380298,-0.0199166192528812,
44.7648617003024));
#171678=CARTESIAN_POINT('Ctrl Pts',(60.1545556301466,-0.0398332865460885,
44.765219826651));
#171679=CARTESIAN_POINT('Ctrl Pts',(60.1553035651452,-0.122792370642498,
44.7666766472281));
#171680=CARTESIAN_POINT('Ctrl Pts',(60.1564477107353,-0.185829839162329,
44.767699708579));
#171681=CARTESIAN_POINT('Ctrl Pts',(60.1619033127762,-0.385803791935395,
44.7706725481338));
#171682=CARTESIAN_POINT('Ctrl Pts',(60.1683551897962,-0.522671862930262,
44.7723013594263));
#171683=CARTESIAN_POINT('Ctrl Pts',(60.2108588050916,-1.15698867587593,
44.7778759236443));
#171684=CARTESIAN_POINT('Ctrl Pts',(60.2800257466418,-1.65159608120817,
44.7765486489021));
#171685=CARTESIAN_POINT('Ctrl Pts',(60.4606916331271,-2.49619847305522,
44.7631669203097));
#171686=CARTESIAN_POINT('Ctrl Pts',(60.5557456738136,-2.84881779514516,
44.7540996937084));
#171687=CARTESIAN_POINT('Ctrl Pts',(60.7253863733359,-3.36792906345627,
44.7352808831733));
#171688=CARTESIAN_POINT('Ctrl Pts',(60.7861804439288,-3.53871633551991,
44.7281741386553));
#171689=CARTESIAN_POINT('Ctrl Pts',(60.8895195636392,-3.80664699843975,
44.7155559443905));
#171690=CARTESIAN_POINT('Ctrl Pts',(60.9291505531237,-3.90489943795874,
44.7106087880791));
#171691=CARTESIAN_POINT('Ctrl Pts',(61.0080817819441,-4.09227342619886,
44.7005575550456));
#171692=CARTESIAN_POINT('Ctrl Pts',(61.0471477319428,-4.18148362684842,
44.695498703219));
#171693=CARTESIAN_POINT('Ctrl Pts',(61.1425166787578,-4.3911861099131,44.6829592667386));
#171694=CARTESIAN_POINT('Ctrl Pts',(61.1998873183109,-4.51116079544422,
44.6752709696757));
#171695=CARTESIAN_POINT('Ctrl Pts',(61.4522052578221,-5.01373677828991,
44.640891948042));
#171696=CARTESIAN_POINT('Ctrl Pts',(61.6684024320991,-5.3848894393157,44.6100734139114));
#171697=CARTESIAN_POINT('Ctrl Pts',(62.1063892874136,-6.03926454968155,
44.5460656424816));
#171698=CARTESIAN_POINT('Ctrl Pts',(62.3211695503718,-6.32647943306077,
44.5141402096601));
#171699=CARTESIAN_POINT('Ctrl Pts',(62.635049775427,-6.70328554143873,44.4672598906789));
#171700=CARTESIAN_POINT('Ctrl Pts',(62.7216254629264,-6.80321365569073,
44.4543092542136));
#171701=CARTESIAN_POINT('Ctrl Pts',(62.8778004195768,-6.97655883481724,
44.4309484982464));
#171702=CARTESIAN_POINT('Ctrl Pts',(62.946605206381,-7.05068289042323,44.4206570104763));
#171703=CARTESIAN_POINT('Ctrl Pts',(63.057100811273,-7.16622502557467,44.4041452694206));
#171704=CARTESIAN_POINT('Ctrl Pts',(63.0980739954297,-7.20833445731159,
44.3980258062601));
#171705=CARTESIAN_POINT('Ctrl Pts',(63.1760015825637,-7.28704883316404,
44.3863968985025));
#171706=CARTESIAN_POINT('Ctrl Pts',(63.2128773424897,-7.32373044764001,
44.3808980271677));
#171707=CARTESIAN_POINT('Ctrl Pts',(63.3182970546813,-7.42700060747211,
44.365185922196));
#171708=CARTESIAN_POINT('Ctrl Pts',(63.3874928474175,-7.49290220592788,
44.3548821316821));
#171709=CARTESIAN_POINT('Ctrl Pts',(63.8336274340093,-7.90598092875223,
44.2884643332931));
#171710=CARTESIAN_POINT('Ctrl Pts',(64.2351126276922,-8.22498923683794,
44.228726166918));
#171711=CARTESIAN_POINT('Ctrl Pts',(64.9788572543902,-8.72938955394705,
44.1166671640505));
#171712=CARTESIAN_POINT('Ctrl Pts',(65.3111565060333,-8.92799775556546,
44.0661759639856));
#171713=CARTESIAN_POINT('Ctrl Pts',(65.7813052853928,-9.17361945482924,
43.9939483178637));
#171714=CARTESIAN_POINT('Ctrl Pts',(65.9102404697575,-9.23751280379088,
43.9740646488257));
#171715=CARTESIAN_POINT('Ctrl Pts',(66.1295558638234,-9.34041736638353,
43.9401132340323));
#171716=CARTESIAN_POINT('Ctrl Pts',(66.2192395628354,-9.38090806588518,
43.926193975315));
#171717=CARTESIAN_POINT('Ctrl Pts',(66.4024019950372,-9.46039777279593,
43.8976951514502));
#171718=CARTESIAN_POINT('Ctrl Pts',(66.4959048809363,-9.4993129734784,43.8831097263679));
#171719=CARTESIAN_POINT('Ctrl Pts',(66.738235768412,-9.59590946159948,43.8452170096186));
#171720=CARTESIAN_POINT('Ctrl Pts',(66.8878527562691,-9.65146434570958,
43.8217335110625));
#171721=CARTESIAN_POINT('Ctrl Pts',(67.2228099917319,-9.76684812705613,
43.7689854471539));
#171722=CARTESIAN_POINT('Ctrl Pts',(67.40867777952,-9.82489103648375,43.7395994111689));
#171723=CARTESIAN_POINT('Ctrl Pts',(68.0691778471187,-10.0102543626263,
43.6348639168474));
#171724=CARTESIAN_POINT('Ctrl Pts',(68.5510961498953,-10.1080158997696,
43.5578620979039));
#171725=CARTESIAN_POINT('Ctrl Pts',(69.3333075600327,-10.2075532106292,
43.4331625120587));
#171726=CARTESIAN_POINT('Ctrl Pts',(69.629973381005,-10.2319216640304,43.3859415000183));
#171727=CARTESIAN_POINT('Ctrl Pts',(70.0076417257142,-10.2460289865898,
43.3262154485403));
#171728=CARTESIAN_POINT('Ctrl Pts',(70.0880040421732,-10.2480611409662,
43.3135291019613));
#171729=CARTESIAN_POINT('Ctrl Pts',(70.2196813255477,-10.2498031702913,
43.2927870270688));
#171730=CARTESIAN_POINT('Ctrl Pts',(70.2709829635795,-10.2500872636329,
43.284717136905));
#171731=CARTESIAN_POINT('Ctrl Pts',(70.3786740949611,-10.249855408428,43.2678031644929));
#171732=CARTESIAN_POINT('Ctrl Pts',(70.4350616130504,-10.2492574044026,
43.258961666125));
#171733=CARTESIAN_POINT('Ctrl Pts',(70.5946988596947,-10.2462150053732,
43.2339680875963));
#171734=CARTESIAN_POINT('Ctrl Pts',(70.6979255942784,-10.2426490761611,
43.2178506375705));
#171735=CARTESIAN_POINT('Ctrl Pts',(70.9388687218488,-10.2305910133748,
43.1803129051586));
#171736=CARTESIAN_POINT('Ctrl Pts',(71.0765081765009,-10.2208484336994,
43.158932150096));
#171737=CARTESIAN_POINT('Ctrl Pts',(71.6046269993583,-10.1724837301423,
43.0770600611678));
#171738=CARTESIAN_POINT('Ctrl Pts',(71.9930125237041,-10.113772390402,43.0171864013352));
#171739=CARTESIAN_POINT('Ctrl Pts',(72.8272572909885,-9.93706629584623,
42.8885466787075));
#171740=CARTESIAN_POINT('Ctrl Pts',(73.2705258626672,-9.81080340615027,
42.8201634146415));
#171741=CARTESIAN_POINT('Ctrl Pts',(73.8321843902975,-9.60817022279217,
42.7331506611185));
#171742=CARTESIAN_POINT('Ctrl Pts',(73.9596903722518,-9.55921025997451,
42.7133744091333));
#171743=CARTESIAN_POINT('Ctrl Pts',(74.1753462646005,-9.47132024709691,
42.6798864231748));
#171744=CARTESIAN_POINT('Ctrl Pts',(74.2639976999074,-9.43369728463362,
42.6661086584929));
#171745=CARTESIAN_POINT('Ctrl Pts',(74.4462863326864,-9.35322791833252,
42.6377558402625));
#171746=CARTESIAN_POINT('Ctrl Pts',(74.5398352423263,-9.31020493537004,
42.6231929538129));
#171747=CARTESIAN_POINT('Ctrl Pts',(74.7855769951801,-9.19258952491959,
42.5849098230035));
#171748=CARTESIAN_POINT('Ctrl Pts',(74.9365956910636,-9.11556821643338,
42.5613538173131));
#171749=CARTESIAN_POINT('Ctrl Pts',(75.186782754201,-8.97991513765112,42.5223029891664));
#171750=CARTESIAN_POINT('Ctrl Pts',(75.2869998209127,-8.92333752135874,
42.50665324063));
#171751=CARTESIAN_POINT('Ctrl Pts',(75.7131453799762,-8.6730549016473,42.4401020361524));
#171752=CARTESIAN_POINT('Ctrl Pts',(76.0291662229347,-8.46269522764463,
42.3907249940435));
#171753=CARTESIAN_POINT('Ctrl Pts',(76.6112096133001,-8.02625244617443,
42.3003501661901));
#171754=CARTESIAN_POINT('Ctrl Pts',(76.8788179653258,-7.80324216687985,
42.25906021943));
#171755=CARTESIAN_POINT('Ctrl Pts',(77.206602026039,-7.50038007347266,42.2092774195641));
#171756=CARTESIAN_POINT('Ctrl Pts',(77.2775531196989,-7.43290933024477,
42.1985531037319));
#171757=CARTESIAN_POINT('Ctrl Pts',(77.3890782390824,-7.32376650238012,
42.1817929999155));
#171758=CARTESIAN_POINT('Ctrl Pts',(77.4302738884402,-7.28275881709131,
42.1756238312646));
#171759=CARTESIAN_POINT('Ctrl Pts',(77.5134159955473,-7.19857660824525,
42.1632214523772));
#171760=CARTESIAN_POINT('Ctrl Pts',(77.5553358622813,-7.15537847828065,
42.1569937530078));
#171761=CARTESIAN_POINT('Ctrl Pts',(77.671675823996,-7.03336027321952,42.1397771701164));
#171762=CARTESIAN_POINT('Ctrl Pts',(77.7452435670081,-6.95371309507588,
42.1289685943587));
#171763=CARTESIAN_POINT('Ctrl Pts',(77.914706706801,-6.76431168256126,42.1042345012843));
#171764=CARTESIAN_POINT('Ctrl Pts',(78.009569098743,-6.6536373863326,42.0905167864875));
#171765=CARTESIAN_POINT('Ctrl Pts',(78.3841168538635,-6.19735516804941,
42.0367963263584));
#171766=CARTESIAN_POINT('Ctrl Pts',(78.6438141651905,-5.83552764715924,
42.000568059813));
#171767=CARTESIAN_POINT('Ctrl Pts',(79.0530090012289,-5.17947451038125,
41.9446143542519));
#171768=CARTESIAN_POINT('Ctrl Pts',(79.2132833316153,-4.89290933682466,
41.9230923896796));
#171769=CARTESIAN_POINT('Ctrl Pts',(79.4163045905892,-4.48541768054737,
41.8963101480454));
#171770=CARTESIAN_POINT('Ctrl Pts',(79.4708356116372,-4.37071142343845,
41.8891741498132));
#171771=CARTESIAN_POINT('Ctrl Pts',(79.5632254819026,-4.16674846523351,
41.8771877520599));
#171772=CARTESIAN_POINT('Ctrl Pts',(79.6019667746226,-4.07791736080481,
41.8721972843117));
#171773=CARTESIAN_POINT('Ctrl Pts',(79.6810616419954,-3.88936357596394,
41.8620872847738));
#171774=CARTESIAN_POINT('Ctrl Pts',(79.7211204682305,-3.7895274661613,41.8570143291583));
#171775=CARTESIAN_POINT('Ctrl Pts',(79.8276449335569,-3.51157212168754,
41.8436649582457));
#171776=CARTESIAN_POINT('Ctrl Pts',(79.8907772006661,-3.33219725453737,
41.8359179284451));
#171777=CARTESIAN_POINT('Ctrl Pts',(80.1991808156335,-2.37232788355457,
41.7991032088621));
#171778=CARTESIAN_POINT('Ctrl Pts',(80.356369193319,-1.56619826433015,41.7839983275279));
#171779=CARTESIAN_POINT('Ctrl Pts',(80.4292834038212,-0.596598155405868,
41.7878709014643));
#171780=CARTESIAN_POINT('Ctrl Pts',(80.4374262264858,-0.442995382190262,
41.7891395160404));
#171781=CARTESIAN_POINT('Ctrl Pts',(80.4442617473451,-0.221867699396258,
41.7919526294067));
#171782=CARTESIAN_POINT('Ctrl Pts',(80.445693233636,-0.15444170199019,41.7929422484627));
#171783=CARTESIAN_POINT('Ctrl Pts',(80.4470597942346,-0.0362263074402389,
41.7949133209436));
#171784=CARTESIAN_POINT('Ctrl Pts',(80.447277108525,0.0145575883017807,
41.7958366534171));
#171785=CARTESIAN_POINT('Ctrl Pts',(80.44693244556,0.129435886879059,41.7980992895404));
#171786=CARTESIAN_POINT('Ctrl Pts',(80.446151160613,0.19352556587406,41.7994835927479));
#171787=CARTESIAN_POINT('Ctrl Pts',(80.441715190715,0.400920069772679,41.8043513192942));
#171788=CARTESIAN_POINT('Ctrl Pts',(80.4357023297616,0.544146405024124,
41.8083128592234));
#171789=CARTESIAN_POINT('Ctrl Pts',(80.4129703810276,0.907042064359414,
41.8198170930238));
#171790=CARTESIAN_POINT('Ctrl Pts',(80.3922414766065,1.12636372738025,41.828136807102));
#171791=CARTESIAN_POINT('Ctrl Pts',(80.281410250048,2.00147495859493,41.8665419581647));
#171792=CARTESIAN_POINT('Ctrl Pts',(80.1357966959054,2.64819629436514,41.9066161249942));
#171793=CARTESIAN_POINT('Ctrl Pts',(79.8778890351759,3.43325423914305,41.9688167868748));
#171794=CARTESIAN_POINT('Ctrl Pts',(79.8224190979191,3.58931492827038,41.9818904577881));
#171795=CARTESIAN_POINT('Ctrl Pts',(79.7264514199753,3.8399877714725,42.0040459577929));
#171796=CARTESIAN_POINT('Ctrl Pts',(79.6882438704159,3.93547592931995,42.0127635132903));
#171797=CARTESIAN_POINT('Ctrl Pts',(79.6106865597225,4.12118350218499,42.0302662368209));
#171798=CARTESIAN_POINT('Ctrl Pts',(79.571459500868,4.21144386550842,42.0390316734453));
#171799=CARTESIAN_POINT('Ctrl Pts',(79.4728282003867,4.42975916261849,42.0608696029861));
#171800=CARTESIAN_POINT('Ctrl Pts',(79.4120769241394,4.55716142752468,42.0741553278741));
#171801=CARTESIAN_POINT('Ctrl Pts',(79.1414639165277,5.09578921273117,42.132690549279));
#171802=CARTESIAN_POINT('Ctrl Pts',(78.9067731816421,5.49348743263157,42.1818781498277));
#171803=CARTESIAN_POINT('Ctrl Pts',(78.3914111492602,6.24571825266891,42.2880802973488));
#171804=CARTESIAN_POINT('Ctrl Pts',(78.1123826943308,6.60014221682026,42.3447970372081));
#171805=CARTESIAN_POINT('Ctrl Pts',(77.749182457666,7.00343540193265,42.4186447482027));
#171806=CARTESIAN_POINT('Ctrl Pts',(77.6861947713095,7.07148195498237,42.4314532254602));
#171807=CARTESIAN_POINT('Ctrl Pts',(77.5868937593087,7.17585961097028,42.4516600036497));
#171808=CARTESIAN_POINT('Ctrl Pts',(77.5512072335956,7.21280575164807,42.458924599158));
#171809=CARTESIAN_POINT('Ctrl Pts',(77.4738726114266,7.29166523002439,42.4746760507925));
#171810=CARTESIAN_POINT('Ctrl Pts',(77.4321377248062,7.33348695929728,42.4831818331765));
#171811=CARTESIAN_POINT('Ctrl Pts',(77.3161658017376,7.44768876893271,42.5068270905542));
#171812=CARTESIAN_POINT('Ctrl Pts',(77.2411969166165,7.51928299708685,42.5221229295825));
#171813=CARTESIAN_POINT('Ctrl Pts',(77.0646167606054,7.68280642087837,42.5581539268041));
#171814=CARTESIAN_POINT('Ctrl Pts',(76.9622280836394,7.77383121131077,42.5790487425704));
#171815=CARTESIAN_POINT('Ctrl Pts',(76.5620669725293,8.11525953956883,42.6606474011505));
#171816=CARTESIAN_POINT('Ctrl Pts',(76.2520344130197,8.35020244765254,42.7237241647739));
#171817=CARTESIAN_POINT('Ctrl Pts',(75.6125317189732,8.7787379928646,42.8528974961526));
#171818=CARTESIAN_POINT('Ctrl Pts',(75.284008834267,8.97264397171745,42.9188173197737));
#171819=CARTESIAN_POINT('Ctrl Pts',(74.8294841094273,9.20691745409177,43.0092499321159));
#171820=CARTESIAN_POINT('Ctrl Pts',(74.712406871467,9.2643803176519,43.0324799664187));
#171821=CARTESIAN_POINT('Ctrl Pts',(74.5073672723046,9.36006333071543,43.0730514916028));
#171822=CARTESIAN_POINT('Ctrl Pts',(74.4199072395709,9.3993474965955,43.0903229149195));
#171823=CARTESIAN_POINT('Ctrl Pts',(74.235829748319,9.47885030221642,43.1266033819154));
#171824=CARTESIAN_POINT('Ctrl Pts',(74.1391195066904,9.5188192075385,43.1456242467234));
#171825=CARTESIAN_POINT('Ctrl Pts',(73.8743575531548,9.62337594965442,43.1975930507576));
#171826=CARTESIAN_POINT('Ctrl Pts',(73.705177513008,9.68492391296871,43.2306872600623));
#171827=CARTESIAN_POINT('Ctrl Pts',(73.2111234426127,9.84958967443477,43.3270501243312));
#171828=CARTESIAN_POINT('Ctrl Pts',(72.8825749904206,9.94058132118908,43.3907794376997));
#171829=CARTESIAN_POINT('Ctrl Pts',(71.9934711344537,10.138121872299,43.5628122627297));
#171830=CARTESIAN_POINT('Ctrl Pts',(71.4274635072994,10.2134351550852,43.6718527906004));
#171831=CARTESIAN_POINT('Ctrl Pts',(70.7642427952375,10.2439126278387,43.8008064812598));
#171832=CARTESIAN_POINT('Ctrl Pts',(70.6700033746303,10.2468924228968,43.8191591167497));
#171833=CARTESIAN_POINT('Ctrl Pts',(70.5214125154391,10.2494625531567,43.8481553665839));
#171834=CARTESIAN_POINT('Ctrl Pts',(70.46707699971,10.2499539351324,43.8587709118182));
#171835=CARTESIAN_POINT('Ctrl Pts',(70.3600499035572,10.2500385885598,43.8797085143961));
#171836=CARTESIAN_POINT('Ctrl Pts',(70.3073600924855,10.2496585372523,43.8900295141274));
#171837=CARTESIAN_POINT('Ctrl Pts',(70.1684414773438,10.2475444433968,43.9172730483735));
#171838=CARTESIAN_POINT('Ctrl Pts',(70.0822310083332,10.2451022628853,43.934212238722));
#171839=CARTESIAN_POINT('Ctrl Pts',(69.5892208234616,10.2246678286397,44.031235834295));
#171840=CARTESIAN_POINT('Ctrl Pts',(69.1838579249568,10.1826483000773,44.111596314172));
#171841=CARTESIAN_POINT('Ctrl Pts',(68.2126659171701,10.0208103096813,44.30439220126));
#171842=CARTESIAN_POINT('Ctrl Pts',(67.6522807306225,9.87612814579876,44.415812418359));
#171843=CARTESIAN_POINT('Ctrl Pts',(66.967048277767,9.63371740256559,44.5514642782997));
#171844=CARTESIAN_POINT('Ctrl Pts',(66.8281030064351,9.58102982810751,44.5789434180771));
#171845=CARTESIAN_POINT('Ctrl Pts',(66.5987556340911,9.48813281509504,44.624254362307));
#171846=CARTESIAN_POINT('Ctrl Pts',(66.5077033647201,9.44966427277173,44.6422305836622));
#171847=CARTESIAN_POINT('Ctrl Pts',(66.3262623846365,9.36980452747353,44.678028393732));
#171848=CARTESIAN_POINT('Ctrl Pts',(66.2358896088186,9.32840357396158,44.6958467144927));
#171849=CARTESIAN_POINT('Ctrl Pts',(66.0087730412191,9.22022208857846,44.7405997219895));
#171850=CARTESIAN_POINT('Ctrl Pts',(65.8728808341264,9.15163883679588,44.7673523152967));
#171851=CARTESIAN_POINT('Ctrl Pts',(65.5749640871962,8.99264085785811,44.8259679838072));
#171852=CARTESIAN_POINT('Ctrl Pts',(65.413755523149,8.90075613378588,44.857662750292));
#171853=CARTESIAN_POINT('Ctrl Pts',(64.8510116982668,8.55894524525192,44.9683121631765));
#171854=CARTESIAN_POINT('Ctrl Pts',(64.4643023879459,8.28490780011079,45.0443422507495));
#171855=CARTESIAN_POINT('Ctrl Pts',(63.9069027295949,7.82753809667824,45.1549880735582));
#171856=CARTESIAN_POINT('Ctrl Pts',(63.7215775920452,7.66370094881584,45.1919813961789));
#171857=CARTESIAN_POINT('Ctrl Pts',(63.4847302524726,7.43825287285645,45.2397158903179));
#171858=CARTESIAN_POINT('Ctrl Pts',(63.4277276403445,7.38269324179563,45.2512413843217));
#171859=CARTESIAN_POINT('Ctrl Pts',(63.3324928269611,7.28764519533255,45.270568735491));
#171860=CARTESIAN_POINT('Ctrl Pts',(63.293919648172,7.24851364405408,45.2784175710745));
#171861=CARTESIAN_POINT('Ctrl Pts',(63.2091527102532,7.16110306387053,45.2957138604662));
#171862=CARTESIAN_POINT('Ctrl Pts',(63.1631131201746,7.11267495385704,45.305139627345));
#171863=CARTESIAN_POINT('Ctrl Pts',(63.0175902577066,6.95653002081841,45.3350268681521));
#171864=CARTESIAN_POINT('Ctrl Pts',(62.9199433224521,6.84707698346953,45.3552245466701));
#171865=CARTESIAN_POINT('Ctrl Pts',(62.6760478551066,6.56144424658541,45.4059852125525));
#171866=CARTESIAN_POINT('Ctrl Pts',(62.5332773196419,6.38230638959384,45.4360027255352));
#171867=CARTESIAN_POINT('Ctrl Pts',(62.0350798095629,5.71198144882276,45.5416088721145));
#171868=CARTESIAN_POINT('Ctrl Pts',(61.717113197429,5.19351337138165,45.6106580551813));
#171869=CARTESIAN_POINT('Ctrl Pts',(61.3859971935355,4.52782309721815,45.683872127209));
#171870=CARTESIAN_POINT('Ctrl Pts',(61.3280118748508,4.40524110317338,45.6967601643282));
#171871=CARTESIAN_POINT('Ctrl Pts',(61.2324813075535,4.19254000294612,45.7181100338742));
#171872=CARTESIAN_POINT('Ctrl Pts',(61.1937748110581,4.10298566251397,45.726797188772));
#171873=CARTESIAN_POINT('Ctrl Pts',(61.1162215581349,3.91633815426279,45.7442822848895));
#171874=CARTESIAN_POINT('Ctrl Pts',(61.0775665003081,3.81917415623401,45.7530428458193));
#171875=CARTESIAN_POINT('Ctrl Pts',(60.9782459576933,3.55806321443092,45.7756819122062));
#171876=CARTESIAN_POINT('Ctrl Pts',(60.9202342389636,3.39310032082398,45.789045543741));
#171877=CARTESIAN_POINT('Ctrl Pts',(60.7347617478341,2.81970978904979,45.8323332666847));
#171878=CARTESIAN_POINT('Ctrl Pts',(60.6283272193907,2.40465593321471,45.8582081005878));
#171879=CARTESIAN_POINT('Ctrl Pts',(60.4505135006237,1.47581028769749,45.9050809027698));
#171880=CARTESIAN_POINT('Ctrl Pts',(60.3912855530988,0.96078511143066,45.9238727462837));
#171881=CARTESIAN_POINT('Ctrl Pts',(60.3671377522047,0.3507955582706,45.9389994618556));
#171882=CARTESIAN_POINT('Ctrl Pts',(60.3647148433716,0.258213846078,45.9411038164074));
#171883=CARTESIAN_POINT('Ctrl Pts',(60.3628372297609,0.110963761724782,
45.9441578451942));
#171884=CARTESIAN_POINT('Ctrl Pts',(60.3625729586119,0.0563133755297087,
45.9452271959814));
#171885=CARTESIAN_POINT('Ctrl Pts',(60.3627431879399,0.00110819107845439,
45.9462441719599));
#171886=CARTESIAN_POINT('Ctrl Pts',(60.3627449410238,0.000554095481200964,
45.9462543729349));
#171887=CARTESIAN_POINT('Ctrl Pts',(60.3627467385963,-1.13830090535116E-13,
45.9462645674752));
#171888=CARTESIAN_POINT('Origin',(69.7358040552328,0.,40.0761166693274));
#171889=CARTESIAN_POINT('',(60.5873249407211,2.12028922040352E-12,47.2199108422682));
#171890=CARTESIAN_POINT('',(60.571124584323,-1.00246535761107E-5,47.128034055528));
#171891=CARTESIAN_POINT('',(59.6415245868576,-1.25526296912604E-15,41.8560104904131));
#171892=CARTESIAN_POINT('Ctrl Pts',(60.5873249407211,4.24183370377617E-12,
47.2199108422682));
#171893=CARTESIAN_POINT('Ctrl Pts',(60.5871564475275,0.0519374417576126,
47.2189552698825));
#171894=CARTESIAN_POINT('Ctrl Pts',(60.5873745952724,0.103873817754455,
47.217919139388));
#171895=CARTESIAN_POINT('Ctrl Pts',(60.5890147051784,0.244664900100287,
47.2148949648136));
#171896=CARTESIAN_POINT('Ctrl Pts',(60.5911823537611,0.333503310376602,
47.2127540973366));
#171897=CARTESIAN_POINT('Ctrl Pts',(60.5986397676944,0.534130867503647,
47.2074058867246));
#171898=CARTESIAN_POINT('Ctrl Pts',(60.6045932141645,0.645880780145617,
47.2040663378404));
#171899=CARTESIAN_POINT('Ctrl Pts',(60.6304768520209,1.01870811056277,47.1917537198258));
#171900=CARTESIAN_POINT('Ctrl Pts',(60.6584366639251,1.27907486694412,47.1812349816448));
#171901=CARTESIAN_POINT('Ctrl Pts',(60.7880120193026,2.16808233850058,47.1390937889102));
#171902=CARTESIAN_POINT('Ctrl Pts',(60.9374985460543,2.78786671149221,47.0990072009642));
#171903=CARTESIAN_POINT('Ctrl Pts',(61.1900215853618,3.52748128373783,47.0387965184134));
#171904=CARTESIAN_POINT('Ctrl Pts',(61.2401114909548,3.66459092317205,47.0270823680358));
#171905=CARTESIAN_POINT('Ctrl Pts',(61.3255306601509,3.88382929836638,47.007454930536));
#171906=CARTESIAN_POINT('Ctrl Pts',(61.3590542006774,3.96666480758704,46.9998286393197));
#171907=CARTESIAN_POINT('Ctrl Pts',(61.4321884305318,4.14081609533997,46.9833470018634));
#171908=CARTESIAN_POINT('Ctrl Pts',(61.4720532157607,4.23201124356125,46.9744516285704));
#171909=CARTESIAN_POINT('Ctrl Pts',(61.5744035817512,4.45717904801317,46.9518224235189));
#171910=CARTESIAN_POINT('Ctrl Pts',(61.6384592545527,4.59038750526218,46.9378399665963));
#171911=CARTESIAN_POINT('Ctrl Pts',(61.8921155097484,5.0899640530361,46.8830904450713));
#171912=CARTESIAN_POINT('Ctrl Pts',(62.1007438273467,5.4458847515296,46.839296717377));
#171913=CARTESIAN_POINT('Ctrl Pts',(62.6031325361139,6.19534142306503,46.7355277545459));
#171914=CARTESIAN_POINT('Ctrl Pts',(62.9048803410925,6.58207761561037,46.6741998497982));
#171915=CARTESIAN_POINT('Ctrl Pts',(63.293271610961,7.01212801484634,46.5952290695433));
#171916=CARTESIAN_POINT('Ctrl Pts',(63.3546606214733,7.07830913213025,46.5827451887376));
#171917=CARTESIAN_POINT('Ctrl Pts',(63.4520625791018,7.18055135714168,46.5629241663619));
#171918=CARTESIAN_POINT('Ctrl Pts',(63.4874920916229,7.2171858876578,46.555711603057));
#171919=CARTESIAN_POINT('Ctrl Pts',(63.5650691999907,7.29620384287648,46.5399101309933));
#171920=CARTESIAN_POINT('Ctrl Pts',(63.6073161003812,7.33848254909956,46.5312996565791));
#171921=CARTESIAN_POINT('Ctrl Pts',(63.7263408827705,7.45551145249706,46.5070311125269));
#171922=CARTESIAN_POINT('Ctrl Pts',(63.8039156271988,7.52940467225742,46.4912029541305));
#171923=CARTESIAN_POINT('Ctrl Pts',(63.9881085295817,7.6993645425123,46.4536182221693));
#171924=CARTESIAN_POINT('Ctrl Pts',(64.0956077657255,7.794402565646,46.4316811394151));
#171925=CARTESIAN_POINT('Ctrl Pts',(64.5348417557687,8.16634727674466,46.3421279905083));
#171926=CARTESIAN_POINT('Ctrl Pts',(64.8818441192843,8.4237997354602,46.2715763734489));
#171927=CARTESIAN_POINT('Ctrl Pts',(65.2700328272329,8.67467908947449,46.1933213604471));
#171928=CARTESIAN_POINT('Ctrl Pts',(65.2961334872847,8.69137610097679,46.1880627096418));
#171929=CARTESIAN_POINT('Ctrl Pts',(65.5828359801181,8.87291260119502,46.1303329060429));
#171930=CARTESIAN_POINT('Ctrl Pts',(65.8506843749084,9.02563123887694,46.076710619746));
#171931=CARTESIAN_POINT('Ctrl Pts',(66.2352631706985,9.22187963702733,46.0002380995568));
#171932=CARTESIAN_POINT('Ctrl Pts',(66.3465147266043,9.27606144512495,45.9781734877417));
#171933=CARTESIAN_POINT('Ctrl Pts',(66.5451966231694,9.36828070798211,45.9388711386241));
#171934=CARTESIAN_POINT('Ctrl Pts',(66.6322270728671,9.4071657652942,45.9216891775339));
#171935=CARTESIAN_POINT('Ctrl Pts',(66.8178548917409,9.48692223649771,45.8851123870488));
#171936=CARTESIAN_POINT('Ctrl Pts',(66.9165760963242,9.52746766906352,45.8657016045507));
#171937=CARTESIAN_POINT('Ctrl Pts',(67.1941347364996,9.63627045143624,45.8112382341993));
#171938=CARTESIAN_POINT('Ctrl Pts',(67.3742908986744,9.70094777096812,45.7760149853913));
#171939=CARTESIAN_POINT('Ctrl Pts',(67.7968053742221,9.83897598914569,45.6936568011168));
#171940=CARTESIAN_POINT('Ctrl Pts',(68.040301335604,9.90832710885732,45.6463811983437));
#171941=CARTESIAN_POINT('Ctrl Pts',(68.6146589195713,10.0483790543752,45.5351293205157));
#171942=CARTESIAN_POINT('Ctrl Pts',(68.9469805374208,10.1115920792684,45.4709604920435));
#171943=CARTESIAN_POINT('Ctrl Pts',(69.6044930380109,10.2020797536131,45.3438728708097));
#171944=CARTESIAN_POINT('Ctrl Pts',(69.9291162995728,10.2305157759936,45.2810663848514));
#171945=CARTESIAN_POINT('Ctrl Pts',(70.3349339806519,10.2459346665038,45.2020885532685));
#171946=CARTESIAN_POINT('Ctrl Pts',(70.4154447647139,10.2480082394494,45.1863971062708));
#171947=CARTESIAN_POINT('Ctrl Pts',(70.5470480816301,10.2497878425927,45.160701858097));
#171948=CARTESIAN_POINT('Ctrl Pts',(70.5981326345252,10.2500822701963,45.1507163660395));
#171949=CARTESIAN_POINT('Ctrl Pts',(70.7050082934605,10.2498690109389,45.1297990482548));
#171950=CARTESIAN_POINT('Ctrl Pts',(70.7607967475691,10.2492848580112,45.1188656108937));
#171951=CARTESIAN_POINT('Ctrl Pts',(70.9180175300403,10.2463057933422,45.0880162319155));
#171952=CARTESIAN_POINT('Ctrl Pts',(71.0194175813151,10.2428201418387,45.0680761907018));
#171953=CARTESIAN_POINT('Ctrl Pts',(71.2555110077228,10.2310581916697,45.0215678482867));
#171954=CARTESIAN_POINT('Ctrl Pts',(71.3901226643612,10.2215815350339,44.9949888957795));
#171955=CARTESIAN_POINT('Ctrl Pts',(71.9005363163362,10.1751141686502,44.8940465128647));
#171956=CARTESIAN_POINT('Ctrl Pts',(72.2743287847078,10.1193283777581,44.8197999528818));
#171957=CARTESIAN_POINT('Ctrl Pts',(73.0686513712459,9.95379079981624,44.6620294481148));
#171958=CARTESIAN_POINT('Ctrl Pts',(73.4871007991411,9.83745271014495,44.5789280180757));
#171959=CARTESIAN_POINT('Ctrl Pts',(74.0420450640677,9.64315886050844,44.4690533444287));
#171960=CARTESIAN_POINT('Ctrl Pts',(74.1860060644551,9.58897364333637,44.4405789949054));
#171961=CARTESIAN_POINT('Ctrl Pts',(74.421224520611,9.4941550969204,44.394104556992));
#171962=CARTESIAN_POINT('Ctrl Pts',(74.5132030050931,9.45546051520291,44.3759442027451));
#171963=CARTESIAN_POINT('Ctrl Pts',(74.6947908819492,9.37583573131703,44.3401152079155));
#171964=CARTESIAN_POINT('Ctrl Pts',(74.7844056646576,9.33494647237442,44.3224451806072));
#171965=CARTESIAN_POINT('Ctrl Pts',(75.0062494890913,9.22972593820227,44.2787282995957));
#171966=CARTESIAN_POINT('Ctrl Pts',(75.1377161578585,9.16377515270088,44.2528446214116));
#171967=CARTESIAN_POINT('Ctrl Pts',(75.6346452031636,8.90059765838181,44.1550648786954));
#171968=CARTESIAN_POINT('Ctrl Pts',(75.9894819445791,8.68340312009844,44.0853829409446));
#171969=CARTESIAN_POINT('Ctrl Pts',(76.7219272858651,8.16991955358759,43.9410902482714));
#171970=CARTESIAN_POINT('Ctrl Pts',(77.0940372937178,7.86730609168436,43.8674927572876));
#171971=CARTESIAN_POINT('Ctrl Pts',(77.5093589639703,7.47718361018491,43.7839344578914));
#171972=CARTESIAN_POINT('Ctrl Pts',(77.5743603497403,7.41446178376609,43.7708110606936));
#171973=CARTESIAN_POINT('Ctrl Pts',(77.6747217500709,7.31498208913852,43.7504651716978));
#171974=CARTESIAN_POINT('Ctrl Pts',(77.7106526285462,7.2788230430956,43.7431638121824));
#171975=CARTESIAN_POINT('Ctrl Pts',(77.7880960133048,7.19969750684008,43.7273864109151));
#171976=CARTESIAN_POINT('Ctrl Pts',(77.8295055023672,7.15663026675921,43.7189245054143));
#171977=CARTESIAN_POINT('Ctrl Pts',(77.9440193072145,7.03539752640193,43.6954567697067));
#171978=CARTESIAN_POINT('Ctrl Pts',(78.0162791671139,6.95642203091557,43.6805704053421));
#171979=CARTESIAN_POINT('Ctrl Pts',(78.1823805770609,6.76899864007856,43.6461892352308));
#171980=CARTESIAN_POINT('Ctrl Pts',(78.2752129779155,6.65965871258256,43.6268473869962));
#171981=CARTESIAN_POINT('Ctrl Pts',(78.6374155050432,6.21424936763742,43.5509491057436));
#171982=CARTESIAN_POINT('Ctrl Pts',(78.8878691627596,5.86285397478378,43.4974868806145));
#171983=CARTESIAN_POINT('Ctrl Pts',(79.1352093193116,5.46480783062019,43.4440029010219));
#171984=CARTESIAN_POINT('Ctrl Pts',(79.1546002497502,5.43322088197864,43.4398045953535));
#171985=CARTESIAN_POINT('Ctrl Pts',(79.3341334925697,5.13718010259645,43.400886083636));
#171986=CARTESIAN_POINT('Ctrl Pts',(79.482535628112,4.8655074135214,43.3683615333574));
#171987=CARTESIAN_POINT('Ctrl Pts',(79.6734714121739,4.47511303312139,43.3260705991843));
#171988=CARTESIAN_POINT('Ctrl Pts',(79.7263361053394,4.36185333848243,43.314304343712));
#171989=CARTESIAN_POINT('Ctrl Pts',(79.816340313465,4.15951384729163,43.2941683456253));
#171990=CARTESIAN_POINT('Ctrl Pts',(79.8543074901914,4.07083532066365,43.2856380090069));
#171991=CARTESIAN_POINT('Ctrl Pts',(79.9322065376245,3.88161064836288,43.2680557166844));
#171992=CARTESIAN_POINT('Ctrl Pts',(79.9718155453191,3.78093859836991,43.2590666237938));
#171993=CARTESIAN_POINT('Ctrl Pts',(80.0781847516176,3.49762409667531,43.2347791536815));
#171994=CARTESIAN_POINT('Ctrl Pts',(80.1414081208651,3.3136454852178,43.2201666573747));
#171995=CARTESIAN_POINT('Ctrl Pts',(80.2763031662515,2.88192563767089,43.1885013418342));
#171996=CARTESIAN_POINT('Ctrl Pts',(80.3440064937989,2.63302899713405,43.1722087327176));
#171997=CARTESIAN_POINT('Ctrl Pts',(80.4801266227141,2.04721819758891,43.1382185405716));
#171998=CARTESIAN_POINT('Ctrl Pts',(80.541252417161,1.70885495919348,43.1218704635874));
#171999=CARTESIAN_POINT('Ctrl Pts',(80.627944089206,1.04081766298725,43.0954585336299));
#172000=CARTESIAN_POINT('Ctrl Pts',(80.6547926742552,0.711737294504319,
43.0851815816499));
#172001=CARTESIAN_POINT('Ctrl Pts',(80.6686481681964,0.299927717328372,
43.0753450364434));
#172002=CARTESIAN_POINT('Ctrl Pts',(80.6704327125468,0.217946679402327,
43.0735356912178));
#172003=CARTESIAN_POINT('Ctrl Pts',(80.6717578321756,0.0839178240909962,
43.0708126560324));
#172004=CARTESIAN_POINT('Ctrl Pts',(80.67188009463,0.0318810271266049,43.0698132826031));
#172005=CARTESIAN_POINT('Ctrl Pts',(80.6713148272797,-0.0770080455644929,
43.0678405802884));
#172006=CARTESIAN_POINT('Ctrl Pts',(80.6705513802445,-0.133857986641344,
43.0668785511626));
#172007=CARTESIAN_POINT('Ctrl Pts',(80.667079714772,-0.294109986102082,
43.0643623114152));
#172008=CARTESIAN_POINT('Ctrl Pts',(80.6632908376584,-0.397484394424257,
43.0629688231807));
#172009=CARTESIAN_POINT('Ctrl Pts',(80.6508593713272,-0.638215106263754,
43.0602789829982));
#172010=CARTESIAN_POINT('Ctrl Pts',(80.6410281260701,-0.775492601098059,
43.0591671216325));
#172011=CARTESIAN_POINT('Ctrl Pts',(80.5933085952772,-1.29632051534599,
43.0566247738066));
#172012=CARTESIAN_POINT('Ctrl Pts',(80.536813390687,-1.67786412892185,43.0582372283862));
#172013=CARTESIAN_POINT('Ctrl Pts',(80.3706280454606,-2.48729888203156,
43.0698348543323));
#172014=CARTESIAN_POINT('Ctrl Pts',(80.2546125106642,-2.91309850439924,
43.0809903021381));
#172015=CARTESIAN_POINT('Ctrl Pts',(80.0614517956559,-3.47799653012537,
43.1030414945953));
#172016=CARTESIAN_POINT('Ctrl Pts',(80.0075614723663,-3.62471446433682,
43.1094536823156));
#172017=CARTESIAN_POINT('Ctrl Pts',(79.913328725701,-3.8644290461771,43.1210703926915));
#172018=CARTESIAN_POINT('Ctrl Pts',(79.8748899114175,-3.95816359123738,
43.1259061289921));
#172019=CARTESIAN_POINT('Ctrl Pts',(79.7958232148824,-4.1432143570785,43.1360375687693));
#172020=CARTESIAN_POINT('Ctrl Pts',(79.7552355746164,-4.23453612509113,
43.1413257403168));
#172021=CARTESIAN_POINT('Ctrl Pts',(79.6508266998838,-4.46060147477623,
43.155136003301));
#172022=CARTESIAN_POINT('Ctrl Pts',(79.5854154597721,-4.59456592259702,
43.1639672045073));
#172023=CARTESIAN_POINT('Ctrl Pts',(79.3244971024167,-5.10092839006078,
43.1998163343256));
#172024=CARTESIAN_POINT('Ctrl Pts',(79.1093833757438,-5.46247750646331,
43.230631984325));
#172025=CARTESIAN_POINT('Ctrl Pts',(78.6011111125618,-6.20884947895576,
43.3051113107463));
#172026=CARTESIAN_POINT('Ctrl Pts',(78.3017326841511,-6.58808201372149,
43.3499154294459));
#172027=CARTESIAN_POINT('Ctrl Pts',(77.9157746364577,-7.01160016243578,
43.4076444552552));
#172028=CARTESIAN_POINT('Ctrl Pts',(77.8537212777866,-7.07789313494804,
43.4169242318052));
#172029=CARTESIAN_POINT('Ctrl Pts',(77.7552995617537,-7.1802631320795,43.4316291627336));
#172030=CARTESIAN_POINT('Ctrl Pts',(77.7195246613939,-7.21691604866152,
43.4369714658208));
#172031=CARTESIAN_POINT('Ctrl Pts',(77.6412383662243,-7.29592258615367,
43.4486534099141));
#172032=CARTESIAN_POINT('Ctrl Pts',(77.5986270650052,-7.33817230198449,
43.4550066387119));
#172033=CARTESIAN_POINT('Ctrl Pts',(77.4786763537277,-7.45502111370519,
43.4728813352592));
#172034=CARTESIAN_POINT('Ctrl Pts',(77.4005342299879,-7.52876784812212,
43.4845149088992));
#172035=CARTESIAN_POINT('Ctrl Pts',(77.2150883630637,-7.69831511441796,
43.5121210388767));
#172036=CARTESIAN_POINT('Ctrl Pts',(77.1069018828138,-7.79309528589141,
43.5282242632328));
#172037=CARTESIAN_POINT('Ctrl Pts',(76.6662076126637,-8.16297015691732,
43.5938985101831));
#172038=CARTESIAN_POINT('Ctrl Pts',(76.3185659012665,-8.41889910404204,
43.6458967804122));
#172039=CARTESIAN_POINT('Ctrl Pts',(75.9248678412809,-8.67177747161641,
43.7054448333481));
#172040=CARTESIAN_POINT('Ctrl Pts',(75.8936102813695,-8.69161375696135,
43.7101767933696));
#172041=CARTESIAN_POINT('Ctrl Pts',(75.6008156388286,-8.87518212604365,
43.7545422217171));
#172042=CARTESIAN_POINT('Ctrl Pts',(75.3321914560878,-9.02697206838936,
43.7955508772855));
#172043=CARTESIAN_POINT('Ctrl Pts',(74.9462627371051,-9.22234575861689,
43.8549769372163));
#172044=CARTESIAN_POINT('Ctrl Pts',(74.8343063316602,-9.27645009603366,
43.8722731053681));
#172045=CARTESIAN_POINT('Ctrl Pts',(74.6343121168603,-9.36858305952962,
43.903271672497));
#172046=CARTESIAN_POINT('Ctrl Pts',(74.5466669634561,-9.40745463550601,
43.9168901811612));
#172047=CARTESIAN_POINT('Ctrl Pts',(74.3596588868407,-9.48722342041452,
43.9460181568663));
#172048=CARTESIAN_POINT('Ctrl Pts',(74.2601729805711,-9.52779173985729,
43.9615552427644));
#172049=CARTESIAN_POINT('Ctrl Pts',(73.9802139575753,-9.63676333365362,
44.0053878124279));
#172050=CARTESIAN_POINT('Ctrl Pts',(73.7984355834092,-9.70156429009606,
44.0339756927895));
#172051=CARTESIAN_POINT('Ctrl Pts',(73.3719200177862,-9.83991029545085,
44.1013020961864));
#172052=CARTESIAN_POINT('Ctrl Pts',(73.1260552626071,-9.90941505802381,
44.1402999252907));
#172053=CARTESIAN_POINT('Ctrl Pts',(72.5474315430654,-10.0493690288865,
44.232338296622));
#172054=CARTESIAN_POINT('Ctrl Pts',(72.2132565585436,-10.1124040507284,
44.2856924209878));
#172055=CARTESIAN_POINT('Ctrl Pts',(71.5534738449002,-10.202362245212,44.3909041972888));
#172056=CARTESIAN_POINT('Ctrl Pts',(71.2284531024807,-10.2305863855897,
44.4426714292048));
#172057=CARTESIAN_POINT('Ctrl Pts',(70.8216437334047,-10.2459391285614,
44.5070095981421));
#172058=CARTESIAN_POINT('Ctrl Pts',(70.7406527336991,-10.248010740629,44.5197958176052));
#172059=CARTESIAN_POINT('Ctrl Pts',(70.608234566533,-10.2497885692664,44.5406553358949));
#172060=CARTESIAN_POINT('Ctrl Pts',(70.5568211392339,-10.2500825110406,
44.5487430955347));
#172061=CARTESIAN_POINT('Ctrl Pts',(70.4492319134183,-10.2498683828576,
44.5656416040368));
#172062=CARTESIAN_POINT('Ctrl Pts',(70.3930580572796,-10.2492835854339,
44.5744499238695));
#172063=CARTESIAN_POINT('Ctrl Pts',(70.2347053238982,-10.2463015870132,
44.5992433882946));
#172064=CARTESIAN_POINT('Ctrl Pts',(70.1325485761743,-10.2428122281872,
44.6151948037664));
#172065=CARTESIAN_POINT('Ctrl Pts',(69.8946394685958,-10.2310366361465,
44.652262738275));
#172066=CARTESIAN_POINT('Ctrl Pts',(69.7589604284561,-10.2215477564663,
44.6733412272971));
#172067=CARTESIAN_POINT('Ctrl Pts',(69.2441679456989,-10.174994202201,44.7531563675436));
#172068=CARTESIAN_POINT('Ctrl Pts',(68.8669901670021,-10.1190765762285,
44.8113137454806));
#172069=CARTESIAN_POINT('Ctrl Pts',(68.066825914051,-9.95340131103121,44.9346989832805));
#172070=CARTESIAN_POINT('Ctrl Pts',(67.6459084115125,-9.83721199074886,
44.9996169626139));
#172071=CARTESIAN_POINT('Ctrl Pts',(67.0875426433126,-9.64315796278377,
45.0860637394411));
#172072=CARTESIAN_POINT('Ctrl Pts',(66.942525244642,-9.58897289101964,45.1085440893086));
#172073=CARTESIAN_POINT('Ctrl Pts',(66.7055975799226,-9.49415453239639,
45.1453217638451));
#172074=CARTESIAN_POINT('Ctrl Pts',(66.6129549614752,-9.45545997345516,
45.1597150932927));
#172075=CARTESIAN_POINT('Ctrl Pts',(66.4300639583688,-9.3758351715069,45.1881535595771));
#172076=CARTESIAN_POINT('Ctrl Pts',(66.339810036177,-9.3349458669878,45.2021992366496));
#172077=CARTESIAN_POINT('Ctrl Pts',(66.1163925046861,-9.22972506860246,
45.2369939366841));
#172078=CARTESIAN_POINT('Ctrl Pts',(65.9840011088537,-9.16377404837579,
45.2576355464542));
#172079=CARTESIAN_POINT('Ctrl Pts',(65.4835943080076,-8.90059447483589,
45.3357129498621));
#172080=CARTESIAN_POINT('Ctrl Pts',(65.1263212256947,-8.68339771016354,
45.3915951293686));
#172081=CARTESIAN_POINT('Ctrl Pts',(64.3886987673181,-8.16991404466073,
45.5065150834696));
#172082=CARTESIAN_POINT('Ctrl Pts',(64.0138622521309,-7.86730371821761,
45.5646244994196));
#172083=CARTESIAN_POINT('Ctrl Pts',(63.5950125094422,-7.47718472766329,
45.6281532192212));
#172084=CARTESIAN_POINT('Ctrl Pts',(63.5294424717323,-7.41446268093463,
45.6380530811232));
#172085=CARTESIAN_POINT('Ctrl Pts',(63.4281746160734,-7.31498272542267,
45.6532598632049));
#172086=CARTESIAN_POINT('Ctrl Pts',(63.3919133817252,-7.27882364471826,
45.658687920089));
#172087=CARTESIAN_POINT('Ctrl Pts',(63.3137442407122,-7.19969814627209,
45.6703492067521));
#172088=CARTESIAN_POINT('Ctrl Pts',(63.2719379716636,-7.15663098044244,
45.6765604866738));
#172089=CARTESIAN_POINT('Ctrl Pts',(63.1563041556976,-7.03539868499352,
45.6936739981997));
#172090=CARTESIAN_POINT('Ctrl Pts',(63.0833109873441,-6.95642356980787,
45.7043996721642));
#172091=CARTESIAN_POINT('Ctrl Pts',(62.9154685813085,-6.76900129687135,
45.7289018372709));
#172092=CARTESIAN_POINT('Ctrl Pts',(62.8216199300911,-6.65966212267454,
45.7424769156831));
#172093=CARTESIAN_POINT('Ctrl Pts',(62.4553067246819,-6.21425882266641,
45.795035775327));
#172094=CARTESIAN_POINT('Ctrl Pts',(62.2016754873669,-5.86286921032458,
45.8304574636465));
#172095=CARTESIAN_POINT('Ctrl Pts',(61.9509507119463,-5.46481180954629,
45.8647954666217));
#172096=CARTESIAN_POINT('Ctrl Pts',(61.9312823810656,-5.43320728852651,
45.8674839294922));
#172097=CARTESIAN_POINT('Ctrl Pts',(61.7492608890216,-5.13715680284549,
45.8923170610155));
#172098=CARTESIAN_POINT('Ctrl Pts',(61.5986899025736,-4.86549261324594,
45.9125097546087));
#172099=CARTESIAN_POINT('Ctrl Pts',(61.4048096975294,-4.47510786706544,
45.9380724816467));
#172100=CARTESIAN_POINT('Ctrl Pts',(61.3511092500408,-4.3618488885061,45.9450965527575));
#172101=CARTESIAN_POINT('Ctrl Pts',(61.2596465005726,-4.15951019677586,
45.9569580944416));
#172102=CARTESIAN_POINT('Ctrl Pts',(61.2210515491285,-4.07083174153613,
45.9619277291097));
#172103=CARTESIAN_POINT('Ctrl Pts',(61.1418368244989,-3.88160671513911,
45.9720488284767));
#172104=CARTESIAN_POINT('Ctrl Pts',(61.1015419590627,-3.78093423329831,
45.9771489368012));
#172105=CARTESIAN_POINT('Ctrl Pts',(60.9932798949756,-3.49761694931462,
45.9907066997055));
#172106=CARTESIAN_POINT('Ctrl Pts',(60.9288709322941,-3.31363594505769,
45.9985991857891));
#172107=CARTESIAN_POINT('Ctrl Pts',(60.791279175395,-2.88190894604371,46.0149805254003));
#172108=CARTESIAN_POINT('Ctrl Pts',(60.7220856319191,-2.63300748931425,
46.0228264525751));
#172109=CARTESIAN_POINT('Ctrl Pts',(60.582549728761,-2.04719203233801,46.0374417944943));
#172110=CARTESIAN_POINT('Ctrl Pts',(60.5195198417882,-1.70882907243014,
46.0429857225426));
#172111=CARTESIAN_POINT('Ctrl Pts',(60.4290257267372,-1.04080017320016,
46.0478165601401));
#172112=CARTESIAN_POINT('Ctrl Pts',(60.4002825268621,-0.711728004843181,
46.0473420685351));
#172113=CARTESIAN_POINT('Ctrl Pts',(60.3838987009321,-0.299926844234377,
46.0428376814325));
#172114=CARTESIAN_POINT('Ctrl Pts',(60.3816029562331,-0.21794597743042,
46.0417478042074));
#172115=CARTESIAN_POINT('Ctrl Pts',(60.3795355269043,-0.0906355194028028,
46.0397477506953));
#172116=CARTESIAN_POINT('Ctrl Pts',(60.3790941463259,-0.0453180362328119,
46.0389753237333));
#172117=CARTESIAN_POINT('Ctrl Pts',(60.3789471275204,1.31869374016412E-10,
46.0381415386512));
#172118=CARTESIAN_POINT('Ctrl Pts',(60.3627467385963,-1.13830090535116E-13,
45.9462645674752));
#172119=CARTESIAN_POINT('Ctrl Pts',(60.3629210969066,-0.0537453435861863,
45.9472534025903));
#172120=CARTESIAN_POINT('Ctrl Pts',(60.3635140173742,-0.107489596541202,
45.9481816946506));
#172121=CARTESIAN_POINT('Ctrl Pts',(60.3662357203024,-0.252129721537147,
45.9505137108538));
#172122=CARTESIAN_POINT('Ctrl Pts',(60.3691429658746,-0.343008082848155,
45.9518021386462));
#172123=CARTESIAN_POINT('Ctrl Pts',(60.3784525920476,-0.549144354899051,
45.9543100815123));
#172124=CARTESIAN_POINT('Ctrl Pts',(60.3855850233311,-0.664358651866915,
45.9554172690278));
#172125=CARTESIAN_POINT('Ctrl Pts',(60.4163177143643,-1.05503640493196,
45.9581327905588));
#172126=CARTESIAN_POINT('Ctrl Pts',(60.4489978372468,-1.32967619768264,
45.9582819908947));
#172127=CARTESIAN_POINT('Ctrl Pts',(60.5885132993943,-2.20373001633204,
45.9526845389634));
#172128=CARTESIAN_POINT('Ctrl Pts',(60.7369835307299,-2.79513263192651,
45.9395791997444));
#172129=CARTESIAN_POINT('Ctrl Pts',(60.9850572371069,-3.51115661396042,
45.9110331525872));
#172130=CARTESIAN_POINT('Ctrl Pts',(61.0370396938302,-3.65135059926042,
45.9048159910799));
#172131=CARTESIAN_POINT('Ctrl Pts',(61.1251537700211,-3.87413141348213,
45.8939207614984));
#172132=CARTESIAN_POINT('Ctrl Pts',(61.1593746367891,-3.95746834551078,
45.8896130140066));
#172133=CARTESIAN_POINT('Ctrl Pts',(61.2335610766254,-4.13165034516851,
45.8801200764335));
#172134=CARTESIAN_POINT('Ctrl Pts',(61.2737528242459,-4.22238656688466,
45.8748907015453));
#172135=CARTESIAN_POINT('Ctrl Pts',(61.3758566536567,-4.44424755395228,
45.8614036960955));
#172136=CARTESIAN_POINT('Ctrl Pts',(61.4392213392701,-4.57466247116494,
45.8528636219607));
#172137=CARTESIAN_POINT('Ctrl Pts',(61.6826735746847,-5.05008549496835,
45.81947997045));
#172138=CARTESIAN_POINT('Ctrl Pts',(61.879326184238,-5.38600561318496,45.7914280866291));
#172139=CARTESIAN_POINT('Ctrl Pts',(62.3783059639627,-6.13745551539409,
45.7186009764369));
#172140=CARTESIAN_POINT('Ctrl Pts',(62.6935772200122,-6.54287847846962,
45.6714425313701));
#172141=CARTESIAN_POINT('Ctrl Pts',(63.1020705535991,-6.99373713347628,
45.6103407892075));
#172142=CARTESIAN_POINT('Ctrl Pts',(63.1674870136203,-7.06392324356832,
45.6005570398216));
#172143=CARTESIAN_POINT('Ctrl Pts',(63.2699187681363,-7.1707596524641,45.5852515637908));
#172144=CARTESIAN_POINT('Ctrl Pts',(63.3062476940756,-7.20807396295211,
45.5798259531585));
#172145=CARTESIAN_POINT('Ctrl Pts',(63.3841084912721,-7.28682911761619,
45.5682062473634));
#172146=CARTESIAN_POINT('Ctrl Pts',(63.4257148039169,-7.3281921431653,45.5620021934324));
#172147=CARTESIAN_POINT('Ctrl Pts',(63.5396952313653,-7.43956450023324,
45.5450155661601));
#172148=CARTESIAN_POINT('Ctrl Pts',(63.6127471497991,-7.50885650709635,
45.5341386032939));
#172149=CARTESIAN_POINT('Ctrl Pts',(63.7834338217886,-7.66601574938943,
45.5087287945943));
#172150=CARTESIAN_POINT('Ctrl Pts',(63.8817580485864,-7.75309171207928,
45.4940945493024));
#172151=CARTESIAN_POINT('Ctrl Pts',(64.2509400991073,-8.06750558799496,
45.4390971857092));
#172152=CARTESIAN_POINT('Ctrl Pts',(64.5317749777085,-8.28246482312865,
45.3971575890294));
#172153=CARTESIAN_POINT('Ctrl Pts',(65.1796830971222,-8.72683161959794,
45.2996129541909));
#172154=CARTESIAN_POINT('Ctrl Pts',(65.5513081540276,-8.94820225798396,
45.2431427454616));
#172155=CARTESIAN_POINT('Ctrl Pts',(66.0530038921372,-9.20510060597355,
45.1659548702342));
#172156=CARTESIAN_POINT('Ctrl Pts',(66.1715292554078,-9.26289296654748,
45.1476553991507));
#172157=CARTESIAN_POINT('Ctrl Pts',(66.3787231055926,-9.35894403805032,
45.1155543724818));
#172158=CARTESIAN_POINT('Ctrl Pts',(66.466885753228,-9.39828742775446,45.1018608747481));
#172159=CARTESIAN_POINT('Ctrl Pts',(66.6520886273164,-9.47776749994737,
45.0730247213876));
#172160=CARTESIAN_POINT('Ctrl Pts',(66.7492160415553,-9.5176644533488,45.0578623295626));
#172161=CARTESIAN_POINT('Ctrl Pts',(67.0141733890003,-9.62169026337531,
45.0163975351537));
#172162=CARTESIAN_POINT('Ctrl Pts',(67.1830910319922,-9.68284408437236,
44.9898517591112));
#172163=CARTESIAN_POINT('Ctrl Pts',(67.6926848912736,-9.85203783106043,
44.9094825471871));
#172164=CARTESIAN_POINT('Ctrl Pts',(68.0374421943896,-9.94641933020242,
44.8547273931204));
#172165=CARTESIAN_POINT('Ctrl Pts',(68.8606804526575,-10.1251489765166,
44.7235902363861));
#172166=CARTESIAN_POINT('Ctrl Pts',(69.3416223638702,-10.1934737053383,
44.6466678097345));
#172167=CARTESIAN_POINT('Ctrl Pts',(69.9679911044351,-10.2363736959526,
44.5472219732214));
#172168=CARTESIAN_POINT('Ctrl Pts',(70.110543023416,-10.2430760478758,44.5246408207548));
#172169=CARTESIAN_POINT('Ctrl Pts',(70.3166748660034,-10.2483506458548,
44.4921015816188));
#172170=CARTESIAN_POINT('Ctrl Pts',(70.3801664949231,-10.2493705227098,
44.4820945678289));
#172171=CARTESIAN_POINT('Ctrl Pts',(70.4938303869501,-10.2501140724956,
44.4642121487561));
#172172=CARTESIAN_POINT('Ctrl Pts',(70.5439972620434,-10.2500649704298,
44.4563311322078));
#172173=CARTESIAN_POINT('Ctrl Pts',(70.6617756049254,-10.2490640284763,
44.4378555056053));
#172174=CARTESIAN_POINT('Ctrl Pts',(70.7293829254277,-10.2478042331192,
44.427270433084));
#172175=CARTESIAN_POINT('Ctrl Pts',(70.9673230379516,-10.240958181047,44.390079295044));
#172176=CARTESIAN_POINT('Ctrl Pts',(71.1375391116156,-10.2317072888623,
44.3635860777138));
#172177=CARTESIAN_POINT('Ctrl Pts',(71.5995033240834,-10.1947550182515,
44.2918838205177));
#172178=CARTESIAN_POINT('Ctrl Pts',(71.8904490470167,-10.1585882197607,
44.2469404631009));
#172179=CARTESIAN_POINT('Ctrl Pts',(72.7395208250848,-10.0150058563067,
44.1159379662807));
#172180=CARTESIAN_POINT('Ctrl Pts',(73.2907769626046,-9.87283043966821,
44.0310331869294));
#172181=CARTESIAN_POINT('Ctrl Pts',(73.9690212236715,-9.63498248067833,
43.9260107583852));
#172182=CARTESIAN_POINT('Ctrl Pts',(74.1096484363916,-9.58209792534047,
43.9042082570258));
#172183=CARTESIAN_POINT('Ctrl Pts',(74.3414367412509,-9.48894970069511,
43.8682253495136));
#172184=CARTESIAN_POINT('Ctrl Pts',(74.4332675145068,-9.45045248926828,
43.8539570690286));
#172185=CARTESIAN_POINT('Ctrl Pts',(74.6160189034456,-9.37062962594823,
43.8255384242235));
#172186=CARTESIAN_POINT('Ctrl Pts',(74.7069263835331,-9.32930112281805,
43.8113900396457));
#172187=CARTESIAN_POINT('Ctrl Pts',(74.9349003330417,-9.22153850265106,
43.775883228647));
#172188=CARTESIAN_POINT('Ctrl Pts',(75.0711172754451,-9.15332794471267,
43.7546431175649));
#172189=CARTESIAN_POINT('Ctrl Pts',(75.3694320448253,-8.99539122241514,
43.708093592273));
#172190=CARTESIAN_POINT('Ctrl Pts',(75.5307236640642,-8.9042263174588,43.6829023872182));
#172191=CARTESIAN_POINT('Ctrl Pts',(76.0897573432447,-8.56763067672749,
43.5955982706218));
#172192=CARTESIAN_POINT('Ctrl Pts',(76.4731412819818,-8.29896087700861,
43.5357170139515));
#172193=CARTESIAN_POINT('Ctrl Pts',(77.037456562796,-7.84235692315833,43.4485821656145));
#172194=CARTESIAN_POINT('Ctrl Pts',(77.2317809219798,-7.67251750957461,
43.4187906970589));
#172195=CARTESIAN_POINT('Ctrl Pts',(77.478104087099,-7.44020544823845,43.3815107049779));
#172196=CARTESIAN_POINT('Ctrl Pts',(77.5359859775027,-7.38431155568068,
43.3727877092191));
#172197=CARTESIAN_POINT('Ctrl Pts',(77.6325014416984,-7.28888816280562,
43.3583141346835));
#172198=CARTESIAN_POINT('Ctrl Pts',(77.6714789556455,-7.24972346637005,
43.3524894778163));
#172199=CARTESIAN_POINT('Ctrl Pts',(77.756893509239,-7.16250023184012,43.3397729638602));
#172200=CARTESIAN_POINT('Ctrl Pts',(77.8031830606127,-7.11429737354174,
43.3329124263439));
#172201=CARTESIAN_POINT('Ctrl Pts',(77.9487082318632,-6.95976294760169,
43.3114361643479));
#172202=CARTESIAN_POINT('Ctrl Pts',(78.0461819095162,-6.85174566132742,
43.2971894866158));
#172203=CARTESIAN_POINT('Ctrl Pts',(78.2887357799658,-6.57118963592098,
43.2620388806591));
#172204=CARTESIAN_POINT('Ctrl Pts',(78.4305347328856,-6.39583619833343,
43.241778663432));
#172205=CARTESIAN_POINT('Ctrl Pts',(78.9402590384094,-5.72125868764573,
43.169795660147));
#172206=CARTESIAN_POINT('Ctrl Pts',(79.2689273126923,-5.19329707652492,
43.1250781316381));
#172207=CARTESIAN_POINT('Ctrl Pts',(79.6086844404968,-4.518604276133,43.0801780059318));
#172208=CARTESIAN_POINT('Ctrl Pts',(79.6667461609775,-4.3974766723292,43.0725691258047));
#172209=CARTESIAN_POINT('Ctrl Pts',(79.7628822454898,-4.18645187756787,
43.0600836221655));
#172210=CARTESIAN_POINT('Ctrl Pts',(79.8020721324873,-4.09709336258671,
43.0550299401882));
#172211=CARTESIAN_POINT('Ctrl Pts',(79.8809588588637,-3.91006239615493,
43.0449353168022));
#172212=CARTESIAN_POINT('Ctrl Pts',(79.9204394425517,-3.812309287656,43.0399285118045));
#172213=CARTESIAN_POINT('Ctrl Pts',(80.0227041100148,-3.54751383887044,
43.0270899072709));
#172214=CARTESIAN_POINT('Ctrl Pts',(80.0826786602154,-3.37940479590762,
43.0197041501388));
#172215=CARTESIAN_POINT('Ctrl Pts',(80.2738526992248,-2.79633897034405,
42.9967365023146));
#172216=CARTESIAN_POINT('Ctrl Pts',(80.3832694847052,-2.37460581584302,
42.9846450180873));
#172217=CARTESIAN_POINT('Ctrl Pts',(80.5618018003175,-1.45150579628832,
42.9685699092611));
#172218=CARTESIAN_POINT('Ctrl Pts',(80.6214510966608,-0.949445864507903,
42.9662086504445));
#172219=CARTESIAN_POINT('Ctrl Pts',(80.6488332517447,-0.352236933514285,
42.9720192689296));
#172220=CARTESIAN_POINT('Ctrl Pts',(80.6518514835544,-0.259336887938741,
42.9731696689341));
#172221=CARTESIAN_POINT('Ctrl Pts',(80.6546790942502,-0.111702451308424,
42.9754008249226));
#172222=CARTESIAN_POINT('Ctrl Pts',(80.6552975981326,-0.056986277958104,
42.9763156374376));
#172223=CARTESIAN_POINT('Ctrl Pts',(80.6556746885256,0.0519676945265764,
42.9783153064823));
#172224=CARTESIAN_POINT('Ctrl Pts',(80.6554407689613,0.106203715414807,
42.9793986064886));
#172225=CARTESIAN_POINT('Ctrl Pts',(80.6536895151984,0.251031796056709,
42.9825226610243));
#172226=CARTESIAN_POINT('Ctrl Pts',(80.6514167543075,0.341606701826619,
42.9847181540605));
#172227=CARTESIAN_POINT('Ctrl Pts',(80.6330993184868,0.82220059335519,42.9976203926994));
#172228=CARTESIAN_POINT('Ctrl Pts',(80.5963815172592,1.21100446686805,43.0124318899873));
#172229=CARTESIAN_POINT('Ctrl Pts',(80.4464285729306,2.20025734822541,43.0603767248664));
#172230=CARTESIAN_POINT('Ctrl Pts',(80.3019601354889,2.79416722331763,43.0989821326822));
#172231=CARTESIAN_POINT('Ctrl Pts',(80.0582437363962,3.51232919463471,43.1571964434274));
#172232=CARTESIAN_POINT('Ctrl Pts',(80.0073340152638,3.65229881537172,43.1691170888978));
#172233=CARTESIAN_POINT('Ctrl Pts',(79.9208882618855,3.87482165377092,43.188995938758));
#172234=CARTESIAN_POINT('Ctrl Pts',(79.8872658527491,3.95812179729244,43.1966499761715));
#172235=CARTESIAN_POINT('Ctrl Pts',(79.8142953100193,4.1322990173888,43.2131045870906));
#172236=CARTESIAN_POINT('Ctrl Pts',(79.7747176624397,4.22306641842177,43.2219412926025));
#172237=CARTESIAN_POINT('Ctrl Pts',(79.6740350787655,4.44515511869587,43.2442155063629));
#172238=CARTESIAN_POINT('Ctrl Pts',(79.6114611227259,4.57576285996777,43.2578856011995));
#172239=CARTESIAN_POINT('Ctrl Pts',(79.5048986406616,4.78661651051017,43.2809079168193));
#172240=CARTESIAN_POINT('Ctrl Pts',(79.4625506151416,4.86769677599351,43.2899966564355));
#172241=CARTESIAN_POINT('Ctrl Pts',(79.2948212238833,5.17862443130876,43.3257779641757));
#172242=CARTESIAN_POINT('Ctrl Pts',(79.1617957323111,5.40408866030519,43.3537046588196));
#172243=CARTESIAN_POINT('Ctrl Pts',(78.83262293428,5.91609954628576,43.4220320630696));
#172244=CARTESIAN_POINT('Ctrl Pts',(78.6302871003758,6.19813365337136,43.4634750166297));
#172245=CARTESIAN_POINT('Ctrl Pts',(78.2713525315724,6.64818542212518,43.5366264382315));
#172246=CARTESIAN_POINT('Ctrl Pts',(78.1225994869778,6.8223182383764,43.5668544867521));
#172247=CARTESIAN_POINT('Ctrl Pts',(77.9140611953691,7.0504050650835,43.6092602171263));
#172248=CARTESIAN_POINT('Ctrl Pts',(77.8592226037651,7.10897730187663,43.6204141512894));
#172249=CARTESIAN_POINT('Ctrl Pts',(77.7656306047343,7.20660055735756,43.6394630792646));
#172250=CARTESIAN_POINT('Ctrl Pts',(77.7272352903052,7.24600426098306,43.6472814578416));
#172251=CARTESIAN_POINT('Ctrl Pts',(77.6417639963485,7.33230720410671,43.6646959930862));
#172252=CARTESIAN_POINT('Ctrl Pts',(77.5945474634561,7.37905645851623,43.6743222202586));
#172253=CARTESIAN_POINT('Ctrl Pts',(77.4432997607954,7.52589357013387,43.7051688088887));
#172254=CARTESIAN_POINT('Ctrl Pts',(77.3376254047933,7.6241898842825,43.7267370479436));
#172255=CARTESIAN_POINT('Ctrl Pts',(77.0633341659678,7.86859514650933,43.7827008928775));
#172256=CARTESIAN_POINT('Ctrl Pts',(76.8919759487901,8.01138531900531,43.8176446406624));
#172257=CARTESIAN_POINT('Ctrl Pts',(76.2301027931177,8.52665885219056,43.9522653118987));
#172258=CARTESIAN_POINT('Ctrl Pts',(75.7110952982463,8.85899961456718,44.0570519771855));
#172259=CARTESIAN_POINT('Ctrl Pts',(75.0479580644837,9.20189918723911,44.1890145874175));
#172260=CARTESIAN_POINT('Ctrl Pts',(74.9293268917585,9.2602782148456,44.2125564061781));
#172261=CARTESIAN_POINT('Ctrl Pts',(74.7225091505826,9.3569854333983,44.2534841448613));
#172262=CARTESIAN_POINT('Ctrl Pts',(74.6348527110893,9.39643524604626,44.2707960936901));
#172263=CARTESIAN_POINT('Ctrl Pts',(74.4512566615219,9.47588217732843,44.3069850517531));
#172264=CARTESIAN_POINT('Ctrl Pts',(74.3552354874421,9.51565687875646,44.3258723855551));
#172265=CARTESIAN_POINT('Ctrl Pts',(74.0948032159035,9.61877876741822,44.3769972229015));
#172266=CARTESIAN_POINT('Ctrl Pts',(73.9293254733919,9.6792599627662,44.4093730810716));
#172267=CARTESIAN_POINT('Ctrl Pts',(73.4166713731958,9.85130809364957,44.5093858144987));
#172268=CARTESIAN_POINT('Ctrl Pts',(73.0649864042846,9.94813044846011,44.577587149333));
#172269=CARTESIAN_POINT('Ctrl Pts',(72.2261774860944,10.1299897403704,44.7398524944165));
#172270=CARTESIAN_POINT('Ctrl Pts',(71.7365088094433,10.1983438376698,44.8342561796209));
#172271=CARTESIAN_POINT('Ctrl Pts',(71.1135125218988,10.2381934697919,44.9551674741933));
#172272=CARTESIAN_POINT('Ctrl Pts',(70.9828739377346,10.2439495431846,44.9805682283276));
#172273=CARTESIAN_POINT('Ctrl Pts',(70.7909403808074,10.2485924268276,45.0179867540857));
#172274=CARTESIAN_POINT('Ctrl Pts',(70.7296964534421,10.2495040933913,45.0299415410962));
#172275=CARTESIAN_POINT('Ctrl Pts',(70.6184403884264,10.2501252936398,45.0516900179658));
#172276=CARTESIAN_POINT('Ctrl Pts',(70.5684310298726,10.2500246503311,45.0614777686095));
#172277=CARTESIAN_POINT('Ctrl Pts',(70.4488203392759,10.2488753040572,45.0849152377932));
#172278=CARTESIAN_POINT('Ctrl Pts',(70.3792271322961,10.2474704627822,45.0985737273884));
#172279=CARTESIAN_POINT('Ctrl Pts',(70.1214640977061,10.2395393724093,45.1492329203671));
#172280=CARTESIAN_POINT('Ctrl Pts',(69.9334926394964,10.2283665196997,45.1863137924143));
#172281=CARTESIAN_POINT('Ctrl Pts',(69.3958588721882,10.1809444913754,45.2926155751259));
#172282=CARTESIAN_POINT('Ctrl Pts',(69.0476403642592,10.1313857049403,45.3617557807614));
#172283=CARTESIAN_POINT('Ctrl Pts',(68.2421753444426,9.97252878900785,45.5217306327631));
#172284=CARTESIAN_POINT('Ctrl Pts',(67.7884573143866,9.84897258228748,45.611862846335));
#172285=CARTESIAN_POINT('Ctrl Pts',(67.1998728434787,9.64282427306771,45.7283974456558));
#172286=CARTESIAN_POINT('Ctrl Pts',(67.0560937525458,9.58869321103137,45.7568356997508));
#172287=CARTESIAN_POINT('Ctrl Pts',(66.8210884633804,9.49394458976434,45.803267894746));
#172288=CARTESIAN_POINT('Ctrl Pts',(66.7291438420976,9.4552584806206,45.8214215184769));
#172289=CARTESIAN_POINT('Ctrl Pts',(66.5475642482472,9.37562691060056,45.8572488022389));
#172290=CARTESIAN_POINT('Ctrl Pts',(66.457924625181,9.33472062605483,45.8749236873815));
#172291=CARTESIAN_POINT('Ctrl Pts',(66.2359053963485,9.22940140113565,45.9186750347101));
#172292=CARTESIAN_POINT('Ctrl Pts',(66.104291083856,9.16336293784568,45.9445877017524));
#172293=CARTESIAN_POINT('Ctrl Pts',(65.6060235529111,8.89940750163991,46.0426305356261));
#172294=CARTESIAN_POINT('Ctrl Pts',(65.2500760480114,8.68137953927731,46.1125299907108));
#172295=CARTESIAN_POINT('Ctrl Pts',(64.5185634190718,8.1679834078953,46.2566432754873));
#172296=CARTESIAN_POINT('Ctrl Pts',(64.1482245484443,7.86669262032007,46.3298943287175));
#172297=CARTESIAN_POINT('Ctrl Pts',(63.7342857131744,7.47797554740454,46.4131714854007));
#172298=CARTESIAN_POINT('Ctrl Pts',(63.6691090366818,7.41509738375306,46.4263298851424));
#172299=CARTESIAN_POINT('Ctrl Pts',(63.5685473570574,7.31543249169649,46.4467159541363));
#172300=CARTESIAN_POINT('Ctrl Pts',(63.5325875742219,7.27924878646794,46.4540230405205));
#172301=CARTESIAN_POINT('Ctrl Pts',(63.455161497815,7.20014972570824,46.4697966184252));
#172302=CARTESIAN_POINT('Ctrl Pts',(63.41379694177,7.15713487938176,46.4782491562529));
#172303=CARTESIAN_POINT('Ctrl Pts',(63.2995621216697,7.03621589125165,46.5016591393423));
#172304=CARTESIAN_POINT('Ctrl Pts',(63.2275291092484,6.95750854247805,46.5164981584575));
#172305=CARTESIAN_POINT('Ctrl Pts',(63.0620658426728,6.77087280472048,46.550745372892));
#172306=CARTESIAN_POINT('Ctrl Pts',(62.9696319172445,6.66206340482518,46.5700026055298));
#172307=CARTESIAN_POINT('Ctrl Pts',(62.6105961049359,6.22088612783867,46.6452295182885));
#172308=CARTESIAN_POINT('Ctrl Pts',(62.3624711536996,5.87353238193372,46.6981790684783));
#172309=CARTESIAN_POINT('Ctrl Pts',(62.1060842513098,5.46251119810423,46.7535972737332));
#172310=CARTESIAN_POINT('Ctrl Pts',(62.0760609759145,5.41346544106682,46.7600995648005));
#172311=CARTESIAN_POINT('Ctrl Pts',(61.8933508275054,5.10927361376937,46.7997454523949));
#172312=CARTESIAN_POINT('Ctrl Pts',(61.7512935358652,4.84765245666622,46.8308963519295));
#172313=CARTESIAN_POINT('Ctrl Pts',(61.566313278203,4.46867822573259,46.8718765570834));
#172314=CARTESIAN_POINT('Ctrl Pts',(61.5139492009717,4.35630335929961,46.8835334313065));
#172315=CARTESIAN_POINT('Ctrl Pts',(61.4245016956969,4.15494833510534,46.9035477964139));
#172316=CARTESIAN_POINT('Ctrl Pts',(61.3866207472589,4.06635466372642,46.912060032723));
#172317=CARTESIAN_POINT('Ctrl Pts',(61.3086361935644,3.87667471311965,46.9296643567785));
#172318=CARTESIAN_POINT('Ctrl Pts',(61.2688747724967,3.77545451536933,46.9386898284297));
#172319=CARTESIAN_POINT('Ctrl Pts',(61.1613788985319,3.48859620573651,46.9632407414657));
#172320=CARTESIAN_POINT('Ctrl Pts',(61.0973327171974,3.3015675145769,46.9780509811067));
#172321=CARTESIAN_POINT('Ctrl Pts',(60.9603164140632,2.86068557313158,47.0102439523115));
#172322=CARTESIAN_POINT('Ctrl Pts',(60.8915956994273,2.60560186705304,47.0268130095019));
#172323=CARTESIAN_POINT('Ctrl Pts',(60.7089553747825,1.80753641260781,47.0725950268692));
#172324=CARTESIAN_POINT('Ctrl Pts',(60.6286562534582,1.25756617858406,47.0955803210865));
#172325=CARTESIAN_POINT('Ctrl Pts',(60.5837428466699,0.564422640247255,
47.1155101252095));
#172326=CARTESIAN_POINT('Ctrl Pts',(60.577532758024,0.425075990803095,47.1190668737045));
#172327=CARTESIAN_POINT('Ctrl Pts',(60.5728429545518,0.232437560486106,
47.1233962230586));
#172328=CARTESIAN_POINT('Ctrl Pts',(60.5719577001284,0.179227946904613,
47.1245301965381));
#172329=CARTESIAN_POINT('Ctrl Pts',(60.5711076850732,0.0840102689892994,
47.1264512370528));
#172330=CARTESIAN_POINT('Ctrl Pts',(60.5709882801534,0.0420052607569114,
47.1272610361969));
#172331=CARTESIAN_POINT('Ctrl Pts',(60.5711245517966,-1.29611701639584E-15,
47.1280338710899));
#172332=CARTESIAN_POINT('Origin',(69.7358040552328,0.,40.0761166693274));
#172333=CARTESIAN_POINT('',(60.7795023650012,-6.55271312842658E-10,48.3098031747286));
#172334=CARTESIAN_POINT('Ctrl Pts',(60.571124584323,-1.00246535761108E-5,
47.128034055528));
#172335=CARTESIAN_POINT('Ctrl Pts',(60.5712148032041,-0.0278113824378972,
47.1285455556463));
#172336=CARTESIAN_POINT('Ctrl Pts',(60.5714169343916,-0.0556025639840617,
47.1290406821915));
#172337=CARTESIAN_POINT('Ctrl Pts',(60.5720858854301,-0.11480023329174,
47.1300604955834));
#172338=CARTESIAN_POINT('Ctrl Pts',(60.5725834899719,-0.146196177168539,
47.1305804830234));
#172339=CARTESIAN_POINT('Ctrl Pts',(60.575032242565,-0.266248040290342,
47.1324880221005));
#172340=CARTESIAN_POINT('Ctrl Pts',(60.5779789971853,-0.35488218316995,
47.133727828746));
#172341=CARTESIAN_POINT('Ctrl Pts',(60.6092552542877,-1.0334123568815,47.1418865635819));
#172342=CARTESIAN_POINT('Ctrl Pts',(60.6867863375073,-1.62004253220283,
47.1411617285872));
#172343=CARTESIAN_POINT('Ctrl Pts',(60.8874434000863,-2.53283045702649,
47.1257427289583));
#172344=CARTESIAN_POINT('Ctrl Pts',(60.9779031647833,-2.86492265784167,
47.117028961743));
#172345=CARTESIAN_POINT('Ctrl Pts',(61.1410732466115,-3.36487994114951,
47.0989433042988));
#172346=CARTESIAN_POINT('Ctrl Pts',(61.2020699062065,-3.53638546197852,
47.0918164663893));
#172347=CARTESIAN_POINT('Ctrl Pts',(61.3056812367078,-3.80515603437629,
47.0791682513928));
#172348=CARTESIAN_POINT('Ctrl Pts',(61.3453491786462,-3.90354199471231,
47.074217486293));
#172349=CARTESIAN_POINT('Ctrl Pts',(61.424291867263,-4.09101024679259,47.0641663919241));
#172350=CARTESIAN_POINT('Ctrl Pts',(61.4633272452909,-4.18018332693093,
47.0591122739339));
#172351=CARTESIAN_POINT('Ctrl Pts',(61.5585061688121,-4.38954657088156,
47.0465996654256));
#172352=CARTESIAN_POINT('Ctrl Pts',(61.6157067757008,-4.50922437742387,
47.0389355170984));
#172353=CARTESIAN_POINT('Ctrl Pts',(61.9586335262266,-5.19268799918991,
46.9922200214171));
#172354=CARTESIAN_POINT('Ctrl Pts',(62.2928722184951,-5.72993047556373,
46.943685630173));
#172355=CARTESIAN_POINT('Ctrl Pts',(62.8073668453159,-6.40877746633383,
46.8673143615842));
#172356=CARTESIAN_POINT('Ctrl Pts',(62.9465139892635,-6.58054681578012,
46.8465372175401));
#172357=CARTESIAN_POINT('Ctrl Pts',(63.1850727850178,-6.85627088397663,
46.8108665824421));
#172358=CARTESIAN_POINT('Ctrl Pts',(63.2813415000775,-6.96290790738683,
46.7964600198185));
#172359=CARTESIAN_POINT('Ctrl Pts',(63.4254277181341,-7.11588985339365,
46.7749196304762));
#172360=CARTESIAN_POINT('Ctrl Pts',(63.4715158877616,-7.16387366600094,
46.7680327961607));
#172361=CARTESIAN_POINT('Ctrl Pts',(63.556775656516,-7.25091744339383,46.7553035211773));
#172362=CARTESIAN_POINT('Ctrl Pts',(63.5958028082764,-7.2901171656847,46.7494812824883));
#172363=CARTESIAN_POINT('Ctrl Pts',(63.6927496964427,-7.3859189542384,46.7350275964303));
#172364=CARTESIAN_POINT('Ctrl Pts',(63.7510252740847,-7.44214793288821,
46.7263469290494));
#172365=CARTESIAN_POINT('Ctrl Pts',(63.9986631721268,-7.67545018964536,
46.6894726448285));
#172366=CARTESIAN_POINT('Ctrl Pts',(64.1940153141472,-7.845888334824,46.6604148077498));
#172367=CARTESIAN_POINT('Ctrl Pts',(64.7586916046057,-8.30178340996116,
46.5761579625035));
#172368=CARTESIAN_POINT('Ctrl Pts',(65.1412784408068,-8.56938334510254,
46.5187538767455));
#172369=CARTESIAN_POINT('Ctrl Pts',(65.6991825987615,-8.90493236734765,
46.4339531611846));
#172370=CARTESIAN_POINT('Ctrl Pts',(65.8603597593676,-8.9959511205643,46.4093400838637));
#172371=CARTESIAN_POINT('Ctrl Pts',(66.1584632334814,-9.15367217966799,
46.3635862445074));
#172372=CARTESIAN_POINT('Ctrl Pts',(66.2945944560027,-9.22180691583146,
46.3426079832871));
#172373=CARTESIAN_POINT('Ctrl Pts',(66.5224559358261,-9.32948465021821,
46.3073506625335));
#172374=CARTESIAN_POINT('Ctrl Pts',(66.6133489666176,-9.37079842131573,
46.2932499279432));
#172375=CARTESIAN_POINT('Ctrl Pts',(66.7961017713411,-9.45061390581593,
46.2648260300776));
#172376=CARTESIAN_POINT('Ctrl Pts',(66.8879490377325,-9.48911710502249,
46.250504967349));
#172377=CARTESIAN_POINT('Ctrl Pts',(67.1198544806631,-9.58231688646064,
46.2142588005508));
#172378=CARTESIAN_POINT('Ctrl Pts',(67.2605746935562,-9.63524219942648,
46.192185963904));
#172379=CARTESIAN_POINT('Ctrl Pts',(68.0376430613358,-9.90778602276534,
46.0699100043904));
#172380=CARTESIAN_POINT('Ctrl Pts',(68.6929573644766,-10.0660067363506,
45.9652586327518));
#172381=CARTESIAN_POINT('Ctrl Pts',(69.5808601216022,-10.1877346382761,
45.8236671205603));
#172382=CARTESIAN_POINT('Ctrl Pts',(69.8037204760739,-10.2106946458299,
45.7881576587774));
#172383=CARTESIAN_POINT('Ctrl Pts',(70.1711086181769,-10.2361102646359,
45.7298248138721));
#172384=CARTESIAN_POINT('Ctrl Pts',(70.3152502964532,-10.2429519182616,
45.7069903189383));
#172385=CARTESIAN_POINT('Ctrl Pts',(70.523230246374,-10.2483170465695,45.6741582330827));
#172386=CARTESIAN_POINT('Ctrl Pts',(70.5869773276538,-10.2493518294266,
45.6641106521459));
#172387=CARTESIAN_POINT('Ctrl Pts',(70.7008828351484,-10.2501118898927,
45.6461897745921));
#172388=CARTESIAN_POINT('Ctrl Pts',(70.7510357683067,-10.2500694791727,
45.6383107340837));
#172389=CARTESIAN_POINT('Ctrl Pts',(70.8673239408612,-10.2490969264566,
45.6200684001011));
#172390=CARTESIAN_POINT('Ctrl Pts',(70.933455253354,-10.2478882161687,45.6097137388107));
#172391=CARTESIAN_POINT('Ctrl Pts',(71.1484918722356,-10.2418254652421,
45.5760992976301));
#172392=CARTESIAN_POINT('Ctrl Pts',(71.2973149936773,-10.2343026359673,
45.5529215986974));
#172393=CARTESIAN_POINT('Ctrl Pts',(72.2558405027365,-10.1643783646006,
45.4040288101855));
#172394=CARTESIAN_POINT('Ctrl Pts',(73.0560702454888,-10.0069883564334,
45.2812576116335));
#172395=CARTESIAN_POINT('Ctrl Pts',(74.0085779719508,-9.69602214883924,
45.1339341707801));
#172396=CARTESIAN_POINT('Ctrl Pts',(74.1865130200952,-9.63232441115741,
45.1063732880928));
#172397=CARTESIAN_POINT('Ctrl Pts',(74.4619826268559,-9.52485547428383,
45.0636344637706));
#172398=CARTESIAN_POINT('Ctrl Pts',(74.560772876472,-9.48449120277262,45.0482929323982));
#172399=CARTESIAN_POINT('Ctrl Pts',(74.7472193492221,-9.4048265966382,45.0193127493898));
#172400=CARTESIAN_POINT('Ctrl Pts',(74.8349897316404,-9.36582906736572,
45.0056590074803));
#172401=CARTESIAN_POINT('Ctrl Pts',(75.0363308297293,-9.27289785179124,
44.9743147558886));
#172402=CARTESIAN_POINT('Ctrl Pts',(75.1494836782866,-9.21807801207909,
44.9566820144759));
#172403=CARTESIAN_POINT('Ctrl Pts',(75.5449595466918,-9.01725522478599,
44.8950087976443));
#172404=CARTESIAN_POINT('Ctrl Pts',(75.8214737807829,-8.85998224334017,
44.8517979763908));
#172405=CARTESIAN_POINT('Ctrl Pts',(76.4698789015359,-8.44954028808022,
44.7505688507741));
#172406=CARTESIAN_POINT('Ctrl Pts',(76.8333495250869,-8.1840296067559,44.6938965114066));
#172407=CARTESIAN_POINT('Ctrl Pts',(77.2905427321294,-7.80112343946986,
44.6235401114811));
#172408=CARTESIAN_POINT('Ctrl Pts',(77.4007012998642,-7.70475351910916,
44.6066682609185));
#172409=CARTESIAN_POINT('Ctrl Pts',(77.5890830040765,-7.532664726504,44.5780052686678));
#172410=CARTESIAN_POINT('Ctrl Pts',(77.6682231850741,-7.45801752128144,
44.5660249995239));
#172411=CARTESIAN_POINT('Ctrl Pts',(77.7893504880082,-7.34006242190119,
44.5478036059522));
#172412=CARTESIAN_POINT('Ctrl Pts',(77.8321568309724,-7.29763479756387,
44.541387207907));
#172413=CARTESIAN_POINT('Ctrl Pts',(77.9154656299549,-7.21359399412603,
44.5289494435067));
#172414=CARTESIAN_POINT('Ctrl Pts',(77.9559932322748,-7.17201005074573,
44.5229226526456));
#172415=CARTESIAN_POINT('Ctrl Pts',(78.0636894564502,-7.05961310135321,
44.5069676192112));
#172416=CARTESIAN_POINT('Ctrl Pts',(78.1302143806874,-6.98817199927902,
44.4971760707883));
#172417=CARTESIAN_POINT('Ctrl Pts',(78.4461193230978,-6.6390657861382,44.450957322891));
#172418=CARTESIAN_POINT('Ctrl Pts',(78.6814420171409,-6.34868604587716,
44.4173747315025));
#172419=CARTESIAN_POINT('Ctrl Pts',(79.1149602139214,-5.74976439653213,
44.3566175617764));
#172420=CARTESIAN_POINT('Ctrl Pts',(79.3135402069697,-5.44217813132996,
44.3293619421705));
#172421=CARTESIAN_POINT('Ctrl Pts',(79.6129935773734,-4.91917326217556,
44.2889637400265));
#172422=CARTESIAN_POINT('Ctrl Pts',(79.7234985966133,-4.70977652232714,
44.2742531957818));
#172423=CARTESIAN_POINT('Ctrl Pts',(79.8768559283336,-4.39325204051632,
44.2541179920027));
#172424=CARTESIAN_POINT('Ctrl Pts',(79.9252539433013,-4.28895629647708,
44.2478114452241));
#172425=CARTESIAN_POINT('Ctrl Pts',(80.0108619709941,-4.09610496024231,
44.2367467145892));
#172426=CARTESIAN_POINT('Ctrl Pts',(80.0485961480015,-4.00780112245531,
44.2319053178921));
#172427=CARTESIAN_POINT('Ctrl Pts',(80.1299350222782,-3.80986632484421,
44.2215527338582));
#172428=CARTESIAN_POINT('Ctrl Pts',(80.1729064929177,-3.6999847728598,44.216141788707));
#172429=CARTESIAN_POINT('Ctrl Pts',(80.3019749275425,-3.3525371606697,44.2000886228256));
#172430=CARTESIAN_POINT('Ctrl Pts',(80.3812706981692,-3.11249779706675,
44.1905278482389));
#172431=CARTESIAN_POINT('Ctrl Pts',(80.4905516205075,-2.73598656892681,
44.1779459418813));
#172432=CARTESIAN_POINT('Ctrl Pts',(80.526681023091,-2.60143807971074,44.1739177365803));
#172433=CARTESIAN_POINT('Ctrl Pts',(80.6787136901535,-1.98605398938358,
44.1576652541872));
#172434=CARTESIAN_POINT('Ctrl Pts',(80.7628924573915,-1.49793652580564,
44.1507276544172));
#172435=CARTESIAN_POINT('Ctrl Pts',(80.827446997135,-0.852294322658078,
44.1502701775411));
#172436=CARTESIAN_POINT('Ctrl Pts',(80.839380454511,-0.698605869535761,
44.1508038580746));
#172437=CARTESIAN_POINT('Ctrl Pts',(80.8541193166427,-0.432663225378754,
44.1528885103362));
#172438=CARTESIAN_POINT('Ctrl Pts',(80.858523369788,-0.320522586653946,
44.1541233691532));
#172439=CARTESIAN_POINT('Ctrl Pts',(80.8624785355301,-0.149774858189465,
44.1565639634004));
#172440=CARTESIAN_POINT('Ctrl Pts',(80.8633430127721,-0.0912030828018238,
44.1575014640504));
#172441=CARTESIAN_POINT('Ctrl Pts',(80.8640419151073,0.0186491112984646,
44.1594513223032));
#172442=CARTESIAN_POINT('Ctrl Pts',(80.8639912768604,0.0699268206422241,
44.1604400821254));
#172443=CARTESIAN_POINT('Ctrl Pts',(80.8629174979052,0.198673804398144,
44.1631179089744));
#172444=CARTESIAN_POINT('Ctrl Pts',(80.861410638048,0.276133945101377,44.1649063761142));
#172445=CARTESIAN_POINT('Ctrl Pts',(80.8516318630623,0.595906695800077,
44.1730070544069));
#172446=CARTESIAN_POINT('Ctrl Pts',(80.8357897122155,0.83787206041321,44.1808377488813));
#172447=CARTESIAN_POINT('Ctrl Pts',(80.7567641370625,1.62332390246877,44.2114772410717));
#172448=CARTESIAN_POINT('Ctrl Pts',(80.6592196732919,2.16215553067159,44.2406474350728));
#172449=CARTESIAN_POINT('Ctrl Pts',(80.4675369104719,2.88777777805181,44.2902009737457));
#172450=CARTESIAN_POINT('Ctrl Pts',(80.4095582262334,3.08356688755194,44.3046436770043));
#172451=CARTESIAN_POINT('Ctrl Pts',(80.2941959382061,3.43453529807525,44.3324615995049));
#172452=CARTESIAN_POINT('Ctrl Pts',(80.2388034243116,3.59031997843296,44.3455156265546));
#172453=CARTESIAN_POINT('Ctrl Pts',(80.1429378206459,3.84066897455588,44.3676461927745));
#172454=CARTESIAN_POINT('Ctrl Pts',(80.1047434918303,3.93610510796475,44.3763602786074));
#172455=CARTESIAN_POINT('Ctrl Pts',(80.0276132484011,4.12075847331712,44.3937658733821));
#172456=CARTESIAN_POINT('Ctrl Pts',(79.9888269187536,4.21002848816928,44.4024333955731));
#172457=CARTESIAN_POINT('Ctrl Pts',(79.9002264450712,4.40627470334876,44.422053521333));
#172458=CARTESIAN_POINT('Ctrl Pts',(79.8498283935279,4.51296253986985,44.4330984400104));
#172459=CARTESIAN_POINT('Ctrl Pts',(79.5126187776257,5.19606077186552,44.5063059973374));
#172460=CARTESIAN_POINT('Ctrl Pts',(79.1742821913063,5.74451787765544,44.5765677906907));
#172461=CARTESIAN_POINT('Ctrl Pts',(78.6583567644974,6.42757934270093,44.6820229833376));
#172462=CARTESIAN_POINT('Ctrl Pts',(78.5240629578254,6.594202497137,44.7093601643086));
#172463=CARTESIAN_POINT('Ctrl Pts',(78.2931446207121,6.86294764063671,44.7563219597435));
#172464=CARTESIAN_POINT('Ctrl Pts',(78.1994176618604,6.96756726847844,44.7753722742591));
#172465=CARTESIAN_POINT('Ctrl Pts',(78.0586718524208,7.11827615544848,44.804001183889));
#172466=CARTESIAN_POINT('Ctrl Pts',(78.0132891658441,7.16593536585266,44.8132356381705));
#172467=CARTESIAN_POINT('Ctrl Pts',(77.9290299288515,7.2527187679944,44.8303916092196));
#172468=CARTESIAN_POINT('Ctrl Pts',(77.8902890125125,7.29197574467653,44.838284212732));
#172469=CARTESIAN_POINT('Ctrl Pts',(77.7936066872988,7.38836303068299,44.8579904287636));
#172470=CARTESIAN_POINT('Ctrl Pts',(77.7353024820702,7.44510788266909,44.8698819765888));
#172471=CARTESIAN_POINT('Ctrl Pts',(77.4816047554304,7.68614265782594,44.9216393160743));
#172472=CARTESIAN_POINT('Ctrl Pts',(77.27975271499,7.86318703315804,44.962852134825));
#172473=CARTESIAN_POINT('Ctrl Pts',(76.7174670584843,8.31798736759351,45.0773622019873));
#172474=CARTESIAN_POINT('Ctrl Pts',(76.3451364867638,8.5794828862537,45.1528650960693));
#172475=CARTESIAN_POINT('Ctrl Pts',(75.8005420867777,8.90905104515565,45.2622380173261));
#172476=CARTESIAN_POINT('Ctrl Pts',(75.641880387846,8.99922098860143,45.2939889082202));
#172477=CARTESIAN_POINT('Ctrl Pts',(75.3480817719023,9.15568800037619,45.3525535375993));
#172478=CARTESIAN_POINT('Ctrl Pts',(75.2137265059827,9.22338111647456,45.3792512183673));
#172479=CARTESIAN_POINT('Ctrl Pts',(74.9884325573904,9.33056232199089,45.423876488021));
#172480=CARTESIAN_POINT('Ctrl Pts',(74.8983263053219,9.37179022542599,45.4416874644431));
#172481=CARTESIAN_POINT('Ctrl Pts',(74.7168568222614,9.45156372102435,45.4774850288662));
#172482=CARTESIAN_POINT('Ctrl Pts',(74.625502504406,9.49010249204443,45.4954697936684));
#172483=CARTESIAN_POINT('Ctrl Pts',(74.3942440458679,9.58360991023536,45.5409093207623));
#172484=CARTESIAN_POINT('Ctrl Pts',(74.2536557864928,9.63677584874654,45.5684531735549));
#172485=CARTESIAN_POINT('Ctrl Pts',(73.5959464807408,9.86857373579511,45.6969766515089));
#172486=CARTESIAN_POINT('Ctrl Pts',(73.0661039440133,10.0073371192394,45.7995116645105));
#172487=CARTESIAN_POINT('Ctrl Pts',(72.2301899963443,10.1537701536665,45.961048660037));
#172488=CARTESIAN_POINT('Ctrl Pts',(71.9304177825758,10.192238742476,46.0189475407777));
#172489=CARTESIAN_POINT('Ctrl Pts',(71.5096073395762,10.2267524012556,46.100496468681));
#172490=CARTESIAN_POINT('Ctrl Pts',(71.3896196493146,10.2343929861575,46.1237802463463));
#172491=CARTESIAN_POINT('Ctrl Pts',(71.1763879444469,10.2440694253526,46.1652427215803));
#172492=CARTESIAN_POINT('Ctrl Pts',(71.0831928121456,10.2469775845504,46.183392984091));
#172493=CARTESIAN_POINT('Ctrl Pts',(70.9358614690237,10.2494883115732,46.2121444938566));
#172494=CARTESIAN_POINT('Ctrl Pts',(70.8817404909017,10.2499657004367,46.2227184841259));
#172495=CARTESIAN_POINT('Ctrl Pts',(70.7747509104128,10.2500299837307,46.2436493857298));
#172496=CARTESIAN_POINT('Ctrl Pts',(70.7218840565727,10.2496371808114,46.2540054154293));
#172497=CARTESIAN_POINT('Ctrl Pts',(70.5819074259259,10.2474728267927,46.2814574155939));
#172498=CARTESIAN_POINT('Ctrl Pts',(70.4948167023751,10.2449727678598,46.2985704526487));
#172499=CARTESIAN_POINT('Ctrl Pts',(69.8631186230343,10.2184660167189,46.4228952904468));
#172500=CARTESIAN_POINT('Ctrl Pts',(69.321364176781,10.1505355790661,46.5305412933948));
#172501=CARTESIAN_POINT('Ctrl Pts',(68.4015272723725,9.95691999091736,46.7132424322025));
#172502=CARTESIAN_POINT('Ctrl Pts',(68.0203930196076,9.85255851926371,46.7889333508227));
#172503=CARTESIAN_POINT('Ctrl Pts',(67.4847246744987,9.67088274177677,46.8950349661311));
#172504=CARTESIAN_POINT('Ctrl Pts',(67.3246142255615,9.61194108129113,46.9267142040233));
#172505=CARTESIAN_POINT('Ctrl Pts',(67.0704531729611,9.51087667780468,46.9769422299198));
#172506=CARTESIAN_POINT('Ctrl Pts',(66.9754389415886,9.47137853925105,46.9957056332596));
#172507=CARTESIAN_POINT('Ctrl Pts',(66.7924881954681,9.39197736983452,47.0318096220627));
#172508=CARTESIAN_POINT('Ctrl Pts',(66.7044881493277,9.352255994829,47.0491643235425));
#172509=CARTESIAN_POINT('Ctrl Pts',(66.4947638623784,9.25389988261604,47.0905001495394));
#172510=CARTESIAN_POINT('Ctrl Pts',(66.3736070676214,9.19404974525078,47.1143595211593));
#172511=CARTESIAN_POINT('Ctrl Pts',(65.7258228253963,8.85752883569113,47.2418509639892));
#172512=CARTESIAN_POINT('Ctrl Pts',(65.2227263756756,8.53633246810886,47.3405117912805));
#172513=CARTESIAN_POINT('Ctrl Pts',(64.5675028067047,8.03073720708396,47.470078292076));
#172514=CARTESIAN_POINT('Ctrl Pts',(64.3893799651125,7.88323492718028,47.5054349807229));
#172515=CARTESIAN_POINT('Ctrl Pts',(64.106046092681,7.63166795566416,47.5620681211979));
#172516=CARTESIAN_POINT('Ctrl Pts',(63.9978167774939,7.53123808994899,47.5838019397277));
#172517=CARTESIAN_POINT('Ctrl Pts',(63.8437240938318,7.38181862714292,47.614938242529));
#172518=CARTESIAN_POINT('Ctrl Pts',(63.7961073795064,7.33471712411558,47.6245876173148));
#172519=CARTESIAN_POINT('Ctrl Pts',(63.7103039766681,7.24813463892236,47.6420318291885));
#172520=CARTESIAN_POINT('Ctrl Pts',(63.671966467166,7.20881216751893,47.6498475097459));
#172521=CARTESIAN_POINT('Ctrl Pts',(63.5790330997845,7.11192197836666,47.668844864131));
#172522=CARTESIAN_POINT('Ctrl Pts',(63.5247863902146,7.05401519000976,47.6799777541437));
#172523=CARTESIAN_POINT('Ctrl Pts',(63.3065223651301,6.81545795282461,47.7249355548842));
#172524=CARTESIAN_POINT('Ctrl Pts',(63.1483043268279,6.62945212943957,47.7579092172451));
#172525=CARTESIAN_POINT('Ctrl Pts',(62.700039465136,6.06223290556525,47.8521989594965));
#172526=CARTESIAN_POINT('Ctrl Pts',(62.4297615124453,5.66570545217994,47.9102024273087));
#172527=CARTESIAN_POINT('Ctrl Pts',(62.0934208371174,5.0891486175109,47.9833990808422));
#172528=CARTESIAN_POINT('Ctrl Pts',(62.0033051966152,4.92446444490717,48.0031395705416));
#172529=CARTESIAN_POINT('Ctrl Pts',(61.8474786200503,4.62021065602418,48.0374935143791));
#172530=CARTESIAN_POINT('Ctrl Pts',(61.7803114853395,4.48148172601328,48.0523867790885));
#172531=CARTESIAN_POINT('Ctrl Pts',(61.674453929789,4.24973781162177,48.076001485579));
#172532=CARTESIAN_POINT('Ctrl Pts',(61.6339834657458,4.15759935959977,48.0850682207215));
#172533=CARTESIAN_POINT('Ctrl Pts',(61.5559721933895,3.97270128857706,48.1026252343321));
#172534=CARTESIAN_POINT('Ctrl Pts',(61.5184190479317,3.87995913646557,48.1111177785738));
#172535=CARTESIAN_POINT('Ctrl Pts',(61.4278217225578,3.64653817106006,48.1317147872399));
#172536=CARTESIAN_POINT('Ctrl Pts',(61.3764764397989,3.50519678930873,48.143489395866));
#172537=CARTESIAN_POINT('Ctrl Pts',(61.1384690317617,2.80271719503812,48.1986344324567));
#172538=CARTESIAN_POINT('Ctrl Pts',(60.9967884040585,2.2268672065966,48.2332713097903));
#172539=CARTESIAN_POINT('Ctrl Pts',(60.8607433709496,1.36008477544737,48.2716507968488));
#172540=CARTESIAN_POINT('Ctrl Pts',(60.8281471100261,1.07670858810491,48.2820955947034));
#172541=CARTESIAN_POINT('Ctrl Pts',(60.7949289875252,0.624213451717764,
48.2957313806341));
#172542=CARTESIAN_POINT('Ctrl Pts',(60.7866872932901,0.455842228828194,
48.3001405576672));
#172543=CARTESIAN_POINT('Ctrl Pts',(60.7808939206339,0.219462490995435,
48.3054587822185));
#172544=CARTESIAN_POINT('Ctrl Pts',(60.7798976545732,0.151577621009194,
48.3068853995553));
#172545=CARTESIAN_POINT('Ctrl Pts',(60.7794341281953,0.0557908786371534,
48.3087604010123));
#172546=CARTESIAN_POINT('Ctrl Pts',(60.779411867806,0.0278954436961792,
48.3092899396518));
#172547=CARTESIAN_POINT('Ctrl Pts',(60.7795023650012,-1.31054137042235E-9,
48.3098031747286));
#172548=CARTESIAN_POINT('',(60.7957027539178,5.63053972823762E-10,48.4016801458623));
#172549=CARTESIAN_POINT('',(59.6415245868576,-1.25526296912604E-15,41.8560104904131));
#172550=CARTESIAN_POINT('Ctrl Pts',(60.7957027539178,1.12610920091049E-9,
48.4016801458622));
#172551=CARTESIAN_POINT('Ctrl Pts',(60.7956407021154,0.0191272543263107,
48.4013282325916));
#172552=CARTESIAN_POINT('Ctrl Pts',(60.7956310882385,0.0382545525903811,
48.4009653897912));
#172553=CARTESIAN_POINT('Ctrl Pts',(60.7958141432303,0.119992421931868,
48.3993683697433));
#172554=CARTESIAN_POINT('Ctrl Pts',(60.7965163606537,0.182598288115929,
48.3980286631963));
#172555=CARTESIAN_POINT('Ctrl Pts',(60.8004959192312,0.379594606971077,
48.3934526272087));
#172556=CARTESIAN_POINT('Ctrl Pts',(60.8058029680528,0.513920459702991,
48.3898042296417));
#172557=CARTESIAN_POINT('Ctrl Pts',(60.8431551615082,1.14837467604115,48.3701598674042));
#172558=CARTESIAN_POINT('Ctrl Pts',(60.9086010446192,1.64565792010428,48.3476930150286));
#172559=CARTESIAN_POINT('Ctrl Pts',(61.0834588810541,2.49413586098243,48.2983014301159));
#172560=CARTESIAN_POINT('Ctrl Pts',(61.1761499579601,2.84798882452612,48.274236671391));
#172561=CARTESIAN_POINT('Ctrl Pts',(61.3423766118459,3.36822335352085,48.2338091552142));
#172562=CARTESIAN_POINT('Ctrl Pts',(61.4019159928038,3.53894144694612,48.2196993707237));
#172563=CARTESIAN_POINT('Ctrl Pts',(61.5033130501057,3.80679120184683,48.19621878482));
#172564=CARTESIAN_POINT('Ctrl Pts',(61.5422425634555,3.90503077212232,48.1873138850712));
#172565=CARTESIAN_POINT('Ctrl Pts',(61.619850380846,4.09239573051365,48.1697632677733));
#172566=CARTESIAN_POINT('Ctrl Pts',(61.6582935509874,4.18160956398272,48.161155106083));
#172567=CARTESIAN_POINT('Ctrl Pts',(61.7522180430712,4.39134505081754,48.1403163522377));
#172568=CARTESIAN_POINT('Ctrl Pts',(61.8087746987146,4.51134859732828,48.1279156262983));
#172569=CARTESIAN_POINT('Ctrl Pts',(62.0562625820615,5.0111248034433,48.074221795361));
#172570=CARTESIAN_POINT('Ctrl Pts',(62.2682268076956,5.37963653237417,48.0295943522921));
#172571=CARTESIAN_POINT('Ctrl Pts',(62.7006251459201,6.03367683168163,47.9401421565941));
#172572=CARTESIAN_POINT('Ctrl Pts',(62.9145602433688,6.32283840416465,47.8964375255591));
#172573=CARTESIAN_POINT('Ctrl Pts',(63.2271517103667,6.70177190310662,47.8328093486643));
#172574=CARTESIAN_POINT('Ctrl Pts',(63.3131788514659,6.80201893769789,47.8153188273904));
#172575=CARTESIAN_POINT('Ctrl Pts',(63.4683178614429,6.9758448396921,47.7837759384149));
#172576=CARTESIAN_POINT('Ctrl Pts',(63.5366358111993,7.05013661455441,47.7698851748001));
#172577=CARTESIAN_POINT('Ctrl Pts',(63.6462902192209,7.16587563302743,47.7475738291046));
#172578=CARTESIAN_POINT('Ctrl Pts',(63.6869136656239,7.20801822301824,47.7393048586609));
#172579=CARTESIAN_POINT('Ctrl Pts',(63.7641238605713,7.28674374510451,47.7235786997223));
#172580=CARTESIAN_POINT('Ctrl Pts',(63.8006322275545,7.32340423822185,47.7161386550899));
#172581=CARTESIAN_POINT('Ctrl Pts',(63.9049076078787,7.42652561564756,47.6948803313079));
#172582=CARTESIAN_POINT('Ctrl Pts',(63.9733149022665,7.4923030583153,47.6809248867538));
#172583=CARTESIAN_POINT('Ctrl Pts',(64.3640529058159,7.85759510535715,47.6011986993135));
#172584=CARTESIAN_POINT('Ctrl Pts',(64.7043143139839,8.1364320630722,47.5317394437224));
#172585=CARTESIAN_POINT('Ctrl Pts',(65.4373550479627,8.66082627983858,47.3831787401561));
#172586=CARTESIAN_POINT('Ctrl Pts',(65.8311129601765,8.90321252224248,47.3039413422658));
#172587=CARTESIAN_POINT('Ctrl Pts',(66.3636434756009,9.18208987898382,47.1978919938694));
#172588=CARTESIAN_POINT('Ctrl Pts',(66.4887097590223,9.24426954336362,47.1730588781052));
#172589=CARTESIAN_POINT('Ctrl Pts',(66.7030038505289,9.3452446399822,47.1306342748845));
#172590=CARTESIAN_POINT('Ctrl Pts',(66.7915826926268,9.38540632480728,47.1131334825956));
#172591=CARTESIAN_POINT('Ctrl Pts',(66.9738078620823,9.46482588748011,47.0772021479379));
#172592=CARTESIAN_POINT('Ctrl Pts',(67.0674945295657,9.50396062911089,47.0587667980213));
#172593=CARTESIAN_POINT('Ctrl Pts',(67.3133700258608,9.6022697012904,47.0104791394805));
#172594=CARTESIAN_POINT('Ctrl Pts',(67.466427738063,9.6591312259943,46.9805139053764));
#172595=CARTESIAN_POINT('Ctrl Pts',(68.2370084144984,9.92396536405127,46.8300649497402));
#172596=CARTESIAN_POINT('Ctrl Pts',(68.8721621277378,10.0743849098331,46.7074752020394));
#172597=CARTESIAN_POINT('Ctrl Pts',(69.7316861643122,10.1902689570851,46.5413312233425));
#172598=CARTESIAN_POINT('Ctrl Pts',(69.9471387215376,10.2121438629284,46.4996529095671));
#172599=CARTESIAN_POINT('Ctrl Pts',(70.3035773732664,10.2365435675069,46.4305030817386));
#172600=CARTESIAN_POINT('Ctrl Pts',(70.4442341038064,10.2431563971155,46.4031643516186));
#172601=CARTESIAN_POINT('Ctrl Pts',(70.6478754054477,10.2483724969894,46.3634708957887));
#172602=CARTESIAN_POINT('Ctrl Pts',(70.710795239774,10.2493826647817,46.3511910729874));
#172603=CARTESIAN_POINT('Ctrl Pts',(70.8235652607529,10.2501154181836,46.3291497587947));
#172604=CARTESIAN_POINT('Ctrl Pts',(70.8734123378434,10.2500619082221,46.3193952783228));
#172605=CARTESIAN_POINT('Ctrl Pts',(70.9894350708341,10.2490588628604,46.2966641919293));
#172606=CARTESIAN_POINT('Ctrl Pts',(71.0556039137051,10.2478214124625,46.2836805737815));
#172607=CARTESIAN_POINT('Ctrl Pts',(71.2725712001932,10.2415810330529,46.2410504157295));
#172608=CARTESIAN_POINT('Ctrl Pts',(71.4232583116735,10.2337865047158,46.2113530303485));
#172609=CARTESIAN_POINT('Ctrl Pts',(72.3746796013367,10.1626722109809,46.0234534774516));
#172610=CARTESIAN_POINT('Ctrl Pts',(73.1654907719064,10.0052509963959,45.8657602557628));
#172611=CARTESIAN_POINT('Ctrl Pts',(74.1073249453324,9.69512549840155,45.67914149771));
#172612=CARTESIAN_POINT('Ctrl Pts',(74.2833350222481,9.63160437773884,45.644306086122));
#172613=CARTESIAN_POINT('Ctrl Pts',(74.5560861964528,9.52437557358169,45.5903945680753));
#172614=CARTESIAN_POINT('Ctrl Pts',(74.6540525278367,9.48404392001777,45.5710451142434));
#172615=CARTESIAN_POINT('Ctrl Pts',(74.8390775828875,9.40439477664596,45.534526891957));
#172616=CARTESIAN_POINT('Ctrl Pts',(74.9262470416164,9.36537583794669,45.5173336333379));
#172617=CARTESIAN_POINT('Ctrl Pts',(75.1263953366559,9.27231057064868,45.4778798904959));
#172618=CARTESIAN_POINT('Ctrl Pts',(75.2389583300217,9.2173708539392,45.4557087705101));
#172619=CARTESIAN_POINT('Ctrl Pts',(75.6386962047256,9.01286644033033,45.3770207602173));
#172620=CARTESIAN_POINT('Ctrl Pts',(75.9197933067054,8.85138375494903,45.3217815902134));
#172621=CARTESIAN_POINT('Ctrl Pts',(76.5636429013016,8.43873533544804,45.195146427409));
#172622=CARTESIAN_POINT('Ctrl Pts',(76.918847927094,8.17661833087698,45.1252023031759));
#172623=CARTESIAN_POINT('Ctrl Pts',(77.3665955832659,7.79833137928525,45.0361197754086));
#172624=CARTESIAN_POINT('Ctrl Pts',(77.4751702165876,7.70251587293689,45.0144379332026));
#172625=CARTESIAN_POINT('Ctrl Pts',(77.6609424390612,7.53131297011153,44.9771509681051));
#172626=CARTESIAN_POINT('Ctrl Pts',(77.73905120902,7.45697907637112,44.9614122133987));
#172627=CARTESIAN_POINT('Ctrl Pts',(77.8586895954159,7.33940908681387,44.9371902559852));
#172628=CARTESIAN_POINT('Ctrl Pts',(77.9010397445653,7.29704328186987,44.928592871904));
#172629=CARTESIAN_POINT('Ctrl Pts',(77.983558384167,7.21301049474357,44.9117909136498));
#172630=CARTESIAN_POINT('Ctrl Pts',(78.023750330805,7.17137067001636,44.9035831216388));
#172631=CARTESIAN_POINT('Ctrl Pts',(78.1307082735172,7.05863650086592,44.8816796267686));
#172632=CARTESIAN_POINT('Ctrl Pts',(78.1968156176301,6.98690742133993,44.8680766381385));
#172633=CARTESIAN_POINT('Ctrl Pts',(78.4928853110067,6.65618915672465,44.8068871295681));
#172634=CARTESIAN_POINT('Ctrl Pts',(78.7106709243835,6.38627106067666,44.7611327084919));
#172635=CARTESIAN_POINT('Ctrl Pts',(79.1378138970357,5.79776604854028,44.6703309407971));
#172636=CARTESIAN_POINT('Ctrl Pts',(79.3440141469304,5.47745183160361,44.6258493945515));
#172637=CARTESIAN_POINT('Ctrl Pts',(79.589169016565,5.04556607541324,44.5723515634568));
#172638=CARTESIAN_POINT('Ctrl Pts',(79.6445452754241,4.94405802254751,44.5602187527157));
#172639=CARTESIAN_POINT('Ctrl Pts',(79.777269572704,4.69069679162793,44.5310239019012));
#172640=CARTESIAN_POINT('Ctrl Pts',(79.8525993070769,4.53778182874249,44.5143498814705));
#172641=CARTESIAN_POINT('Ctrl Pts',(79.967579539728,4.28900376493974,44.4887321738162));
#172642=CARTESIAN_POINT('Ctrl Pts',(80.0096189256019,4.19432912719339,44.4793252236839));
#172643=CARTESIAN_POINT('Ctrl Pts',(80.0882227485604,4.00987807881692,44.4616551540784));
#172644=CARTESIAN_POINT('Ctrl Pts',(80.1249614132303,3.92019121743338,44.4533583100141));
#172645=CARTESIAN_POINT('Ctrl Pts',(80.2107503757952,3.70207041534065,44.4338871232293));
#172646=CARTESIAN_POINT('Ctrl Pts',(80.2585199403275,3.57313125421282,44.4229615588669));
#172647=CARTESIAN_POINT('Ctrl Pts',(80.4581007480095,2.99961265964152,44.3769045866386));
#172648=CARTESIAN_POINT('Ctrl Pts',(80.5822739415818,2.5456011955061,44.3471333409612));
#172649=CARTESIAN_POINT('Ctrl Pts',(80.7528314314767,1.69989962469362,44.3028742635563));
#172650=CARTESIAN_POINT('Ctrl Pts',(80.8085692791001,1.31109515934199,44.286697083169));
#172651=CARTESIAN_POINT('Ctrl Pts',(80.8540160308513,0.781627644295828,
44.2696724388824));
#172652=CARTESIAN_POINT('Ctrl Pts',(80.8631120487898,0.643072813701096,
44.2656755941091));
#172653=CARTESIAN_POINT('Ctrl Pts',(80.874153401148,0.400364665669781,44.2594349753772));
#172654=CARTESIAN_POINT('Ctrl Pts',(80.8773178009215,0.29629222971149,44.2570031128034));
#172655=CARTESIAN_POINT('Ctrl Pts',(80.8797853678576,0.135202963460496,
44.2536006461113));
#172656=CARTESIAN_POINT('Ctrl Pts',(80.8801879312855,0.0782135254226426,
44.2524669349703));
#172657=CARTESIAN_POINT('Ctrl Pts',(80.8800578296401,-0.030741306703425,
44.2504299779556));
#172658=CARTESIAN_POINT('Ctrl Pts',(80.8796044925397,-0.0827043997496042,
44.2495150116257));
#172659=CARTESIAN_POINT('Ctrl Pts',(80.8774342689301,-0.216246525200686,
44.2473114193674));
#172660=CARTESIAN_POINT('Ctrl Pts',(80.8751443945932,-0.297814272844059,
44.2461073780376));
#172661=CARTESIAN_POINT('Ctrl Pts',(80.859229190897,-0.696762037044488,
44.2409337106242));
#172662=CARTESIAN_POINT('Ctrl Pts',(80.831984558409,-1.0134545438031,44.2390474765423));
#172663=CARTESIAN_POINT('Ctrl Pts',(80.7452105349251,-1.66884695902908,
44.2402311211581));
#172664=CARTESIAN_POINT('Ctrl Pts',(80.6832998391857,-2.00684548315895,
44.2437162865044));
#172665=CARTESIAN_POINT('Ctrl Pts',(80.5440555254029,-2.59994400080739,
44.2553124037534));
#172666=CARTESIAN_POINT('Ctrl Pts',(80.4734081546615,-2.85631448270343,
44.2621957986621));
#172667=CARTESIAN_POINT('Ctrl Pts',(80.3329511489704,-3.29909646664805,
44.2774697691701));
#172668=CARTESIAN_POINT('Ctrl Pts',(80.2674520612435,-3.48675357479172,
44.2850386108823));
#172669=CARTESIAN_POINT('Ctrl Pts',(80.1577340117372,-3.77434325417801,
44.2983608575186));
#172670=CARTESIAN_POINT('Ctrl Pts',(80.1172360159011,-3.87567580319108,
44.3033939398344));
#172671=CARTESIAN_POINT('Ctrl Pts',(80.0379033032512,-4.06545065503559,
44.3134617818319));
#172672=CARTESIAN_POINT('Ctrl Pts',(79.9994149115417,-4.1540283220643,44.318429563002));
#172673=CARTESIAN_POINT('Ctrl Pts',(79.9086507796542,-4.35518839907081,
44.3303263837583));
#172674=CARTESIAN_POINT('Ctrl Pts',(79.8555834491748,-4.46738769859569,
44.3374095135131));
#172675=CARTESIAN_POINT('Ctrl Pts',(79.6688597075322,-4.84450684769502,
44.3627336945338));
#172676=CARTESIAN_POINT('Ctrl Pts',(79.5258984371408,-5.1045276194319,44.3827790337421));
#172677=CARTESIAN_POINT('Ctrl Pts',(79.3406140704187,-5.40964398127828,
44.4093653935485));
#172678=CARTESIAN_POINT('Ctrl Pts',(79.3087489438537,-5.4610923568507,44.4139570169332));
#172679=CARTESIAN_POINT('Ctrl Pts',(79.0478189849678,-5.87421542838934,
44.4517002556594));
#172680=CARTESIAN_POINT('Ctrl Pts',(78.7970661222546,-6.2213117667756,44.4888720436358));
#172681=CARTESIAN_POINT('Ctrl Pts',(78.4345178552781,-6.66221925756195,
44.5429909868608));
#172682=CARTESIAN_POINT('Ctrl Pts',(78.3411765096075,-6.77099455615806,
44.5569517329799));
#172683=CARTESIAN_POINT('Ctrl Pts',(78.1741232844086,-6.95757949211454,
44.5819396297114));
#172684=CARTESIAN_POINT('Ctrl Pts',(78.101406859692,-7.03626957578673,44.5928172589728));
#172685=CARTESIAN_POINT('Ctrl Pts',(77.9861018551028,-7.15716778611019,
44.6100491219602));
#172686=CARTESIAN_POINT('Ctrl Pts',(77.9443495293131,-7.20017925531297,
44.6162855521785));
#172687=CARTESIAN_POINT('Ctrl Pts',(77.8661999123292,-7.27927653233073,
44.6279487108804));
#172688=CARTESIAN_POINT('Ctrl Pts',(77.8299041858663,-7.31546183368558,
44.633361592367));
#172689=CARTESIAN_POINT('Ctrl Pts',(77.7284017317043,-7.41513917151991,
44.6484910985241));
#172690=CARTESIAN_POINT('Ctrl Pts',(77.6626204554461,-7.47802743249217,
44.6582873623916));
#172691=CARTESIAN_POINT('Ctrl Pts',(77.2450302830985,-7.8666739804324,44.7204585636653));
#172692=CARTESIAN_POINT('Ctrl Pts',(76.8716682127879,-8.16788997248872,
44.775996631079));
#172693=CARTESIAN_POINT('Ctrl Pts',(76.1343684641899,-8.68126788593136,
44.8868874150028));
#172694=CARTESIAN_POINT('Ctrl Pts',(75.7756326123108,-8.89934071476048,
44.9413135934751));
#172695=CARTESIAN_POINT('Ctrl Pts',(75.2735911890999,-9.16334040808751,
45.0184035461415));
#172696=CARTESIAN_POINT('Ctrl Pts',(75.141003759556,-9.22938356001108,45.0388428221052));
#172697=CARTESIAN_POINT('Ctrl Pts',(74.9173626519533,-9.33470837874229,
45.0734551423237));
#172698=CARTESIAN_POINT('Ctrl Pts',(74.8270754120788,-9.37561558374381,
45.0874648399649));
#172699=CARTESIAN_POINT('Ctrl Pts',(74.6441953046535,-9.45524750118546,
45.1159138546512));
#172700=CARTESIAN_POINT('Ctrl Pts',(74.5515978879351,-9.49393319005151,
45.1303547941148));
#172701=CARTESIAN_POINT('Ctrl Pts',(74.3149414988765,-9.5886777241126,45.1673513814753));
#172702=CARTESIAN_POINT('Ctrl Pts',(74.1701633832244,-9.6428060246807,45.1900675671839));
#172703=CARTESIAN_POINT('Ctrl Pts',(73.5791515094535,-9.8483773786203,45.2830999932603));
#172704=CARTESIAN_POINT('Ctrl Pts',(73.1240704257277,-9.97159930842423,
45.3554491140219));
#172705=CARTESIAN_POINT('Ctrl Pts',(72.3137077236981,-10.1307999853763,
45.4846431810268));
#172706=CARTESIAN_POINT('Ctrl Pts',(71.9619082670843,-10.1806572951188,
45.5408358972255));
#172707=CARTESIAN_POINT('Ctrl Pts',(71.419063013793,-10.2283015198731,45.6271766377918));
#172708=CARTESIAN_POINT('Ctrl Pts',(71.2294789563311,-10.2395124908403,
45.6572604419998));
#172709=CARTESIAN_POINT('Ctrl Pts',(70.9696001391121,-10.2474643850277,
45.6983167703373));
#172710=CARTESIAN_POINT('Ctrl Pts',(70.8995021632802,-10.2488718573973,
45.709372866089));
#172711=CARTESIAN_POINT('Ctrl Pts',(70.7790523440288,-10.2500238663365,
45.7283336507061));
#172712=CARTESIAN_POINT('Ctrl Pts',(70.7287083677262,-10.250125400347,45.7362473225106));
#172713=CARTESIAN_POINT('Ctrl Pts',(70.6167431657534,-10.2495062547478,
45.7538210177922));
#172714=CARTESIAN_POINT('Ctrl Pts',(70.5551248958887,-10.2485963603833,
45.7634752051308));
#172715=CARTESIAN_POINT('Ctrl Pts',(70.3621285679459,-10.2439634854918,
45.7936656451819));
#172716=CARTESIAN_POINT('Ctrl Pts',(70.2308030065516,-10.2382220100505,
45.8141397337392));
#172717=CARTESIAN_POINT('Ctrl Pts',(69.603662278349,-10.1984209701417,45.9116693665396));
#172718=CARTESIAN_POINT('Ctrl Pts',(69.1105498406412,-10.1300647358911,
45.9876580424967));
#172719=CARTESIAN_POINT('Ctrl Pts',(68.269598150233,-9.94898088705509,46.1173325602242));
#172720=CARTESIAN_POINT('Ctrl Pts',(67.9191065053259,-9.85336098913091,
46.1713972467541));
#172721=CARTESIAN_POINT('Ctrl Pts',(67.4042453606154,-9.68241751761035,
46.2510503813024));
#172722=CARTESIAN_POINT('Ctrl Pts',(67.2355450232222,-9.62134447903006,
46.2771863361049));
#172723=CARTESIAN_POINT('Ctrl Pts',(66.9708554109246,-9.51742658013076,
46.3182577645633));
#172724=CARTESIAN_POINT('Ctrl Pts',(66.8737671284838,-9.47754434971928,
46.3333366431497));
#172725=CARTESIAN_POINT('Ctrl Pts',(66.6885929406964,-9.39806857571963,
46.3621217097281));
#172726=CARTESIAN_POINT('Ctrl Pts',(66.6004193911351,-9.35871280994671,
46.3758394525262));
#172727=CARTESIAN_POINT('Ctrl Pts',(66.3931188524541,-9.26258522860232,
46.4081144016209));
#172728=CARTESIAN_POINT('Ctrl Pts',(66.2745057386477,-9.20472423152712,
46.426600485627));
#172729=CARTESIAN_POINT('Ctrl Pts',(65.7831394063063,-8.95296304978737,
46.5032382722179));
#172730=CARTESIAN_POINT('Ctrl Pts',(65.4213712997427,-8.73808896840144,
46.5598214397522));
#172731=CARTESIAN_POINT('Ctrl Pts',(64.7752916217732,-8.29771000806215,
46.6605449161024));
#172732=CARTESIAN_POINT('Ctrl Pts',(64.4877218187872,-8.07831618324674,
46.7052358856107));
#172733=CARTESIAN_POINT('Ctrl Pts',(64.1111484677427,-7.75791190049661,
46.7630848549705));
#172734=CARTESIAN_POINT('Ctrl Pts',(64.0117379420787,-7.66992676327865,
46.7782859186802));
#172735=CARTESIAN_POINT('Ctrl Pts',(63.8394005405125,-7.51129971534814,
46.8044762360614));
#172736=CARTESIAN_POINT('Ctrl Pts',(63.7657699365944,-7.44147409507387,
46.8156113359947));
#172737=CARTESIAN_POINT('Ctrl Pts',(63.6511017124594,-7.32944738852989,
46.8328498123164));
#172738=CARTESIAN_POINT('Ctrl Pts',(63.6093801447359,-7.28797873600959,
46.8390998043601));
#172739=CARTESIAN_POINT('Ctrl Pts',(63.5314791545818,-7.20920587032642,
46.8507238423054));
#172740=CARTESIAN_POINT('Ctrl Pts',(63.4952231208372,-7.17198263228146,
46.8561147467794));
#172741=CARTESIAN_POINT('Ctrl Pts',(63.393311076075,-7.06574880299513,46.8712168930763));
#172742=CARTESIAN_POINT('Ctrl Pts',(63.3283208608638,-6.9960868238204,46.8807865736354));
#172743=CARTESIAN_POINT('Ctrl Pts',(62.9058078137151,-6.53036755962993,
46.9426366692795));
#172744=CARTESIAN_POINT('Ctrl Pts',(62.5782585329474,-6.10742215544912,
46.9888705721308));
#172745=CARTESIAN_POINT('Ctrl Pts',(62.1111184685539,-5.39605665124973,
47.0532787316343));
#172746=CARTESIAN_POINT('Ctrl Pts',(61.9496191976245,-5.12354854216499,
47.0751609016335));
#172747=CARTESIAN_POINT('Ctrl Pts',(61.7203636854676,-4.69261631022918,
47.1057304556297));
#172748=CARTESIAN_POINT('Ctrl Pts',(61.6436342145201,-4.53929301461325,
47.1158587132025));
#172749=CARTESIAN_POINT('Ctrl Pts',(61.5265598997261,-4.2900231366227,47.1311471143641));
#172750=CARTESIAN_POINT('Ctrl Pts',(61.4837931720625,-4.19527456183938,
47.136691942056));
#172751=CARTESIAN_POINT('Ctrl Pts',(61.4038513012846,-4.01078933828968,
47.1469765956848));
#172752=CARTESIAN_POINT('Ctrl Pts',(61.3664974894336,-3.92114377790846,
47.1517448612107));
#172753=CARTESIAN_POINT('Ctrl Pts',(61.2793149775345,-3.70331901729009,
47.1627785320664));
#172754=CARTESIAN_POINT('Ctrl Pts',(61.2307659198831,-3.57463799286622,
47.1688410958831));
#172755=CARTESIAN_POINT('Ctrl Pts',(61.0402420148368,-3.03746267321418,
47.1922564120649));
#172756=CARTESIAN_POINT('Ctrl Pts',(60.9213279926237,-2.62111073909064,
47.2059429267996));
#172757=CARTESIAN_POINT('Ctrl Pts',(60.7030599179109,-1.62509682914602,
47.2276317923128));
#172758=CARTESIAN_POINT('Ctrl Pts',(60.6262083473102,-1.04199845955352,
47.2318458860108));
#172759=CARTESIAN_POINT('Ctrl Pts',(60.594289766227,-0.360824028936842,
47.2253546100265));
#172760=CARTESIAN_POINT('Ctrl Pts',(60.5911399959984,-0.266007535216332,
47.2241945180865));
#172761=CARTESIAN_POINT('Ctrl Pts',(60.5881999181426,-0.116060049539068,
47.2219423547029));
#172762=CARTESIAN_POINT('Ctrl Pts',(60.5875550318019,-0.0609487046800113,
47.2210254656653));
#172763=CARTESIAN_POINT('Ctrl Pts',(60.5873381061323,-0.00389096929625129,
47.2199823173059));
#172764=CARTESIAN_POINT('Ctrl Pts',(60.5873312521756,-0.0019454838982729,
47.2199466363049));
#172765=CARTESIAN_POINT('Ctrl Pts',(60.5873249407211,4.24183370377617E-12,
47.2199108422682));
#172766=CARTESIAN_POINT('Origin',(69.7358040552328,0.,40.0761166693274));
#172767=CARTESIAN_POINT('',(61.0040805671216,1.7419825273942E-11,49.583449449497));
#172768=CARTESIAN_POINT('',(60.9878801781973,-1.65377492662557E-11,49.4915724783198));
#172769=CARTESIAN_POINT('',(59.6415245868576,-1.25526296912604E-15,41.8560104904131));
#172770=CARTESIAN_POINT('Ctrl Pts',(61.0040805671216,3.48409058108532E-11,
49.583449449497));
#172771=CARTESIAN_POINT('Ctrl Pts',(61.0040673449976,0.00407567382671532,
49.5833744631057));
#172772=CARTESIAN_POINT('Ctrl Pts',(61.0040565037605,0.00815135186697398,
49.5832989804273));
#172773=CARTESIAN_POINT('Ctrl Pts',(61.0039320934917,0.0680854659092492,
49.5821816953104));
#172774=CARTESIAN_POINT('Ctrl Pts',(61.0042633855356,0.123942179426902,
49.5810473211021));
#172775=CARTESIAN_POINT('Ctrl Pts',(61.0064153766429,0.278278712675812,
49.5776595482583));
#172776=CARTESIAN_POINT('Ctrl Pts',(61.0091799556003,0.376735212894865,
49.5752131984396));
#172777=CARTESIAN_POINT('Ctrl Pts',(61.0325051331097,0.928931211202058,
49.5599333442491));
#172778=CARTESIAN_POINT('Ctrl Pts',(61.0812548371948,1.38082706604539,49.5415343461584));
#172779=CARTESIAN_POINT('Ctrl Pts',(61.2228842771604,2.1913329685438,49.4988628223748));
#172780=CARTESIAN_POINT('Ctrl Pts',(61.3057167948855,2.55101398941332,49.4763572651825));
#172781=CARTESIAN_POINT('Ctrl Pts',(61.4546898524297,3.0693911988267,49.4389002220721));
#172782=CARTESIAN_POINT('Ctrl Pts',(61.5058965644992,3.23224647348887,49.4263831544526));
#172783=CARTESIAN_POINT('Ctrl Pts',(61.6081089505079,3.53117622055814,49.4020224914558));
#172784=CARTESIAN_POINT('Ctrl Pts',(61.6580017427047,3.6675995294168,49.3903579582932));
#172785=CARTESIAN_POINT('Ctrl Pts',(61.7467760692201,3.89528556576239,49.3699634930242));
#172786=CARTESIAN_POINT('Ctrl Pts',(61.7841293413855,3.98714218525543,49.3614765517485));
#172787=CARTESIAN_POINT('Ctrl Pts',(61.8578013224181,4.16106077273271,49.3449095933209));
#172788=CARTESIAN_POINT('Ctrl Pts',(61.8938792801003,4.24321824562081,49.336867969315));
#172789=CARTESIAN_POINT('Ctrl Pts',(61.9925396913437,4.46012767106206,49.3150578710357));
#172790=CARTESIAN_POINT('Ctrl Pts',(62.0569666463966,4.59398704125687,49.3009971595692));
#172791=CARTESIAN_POINT('Ctrl Pts',(62.3072820697831,5.08641890005117,49.2469812440128));
#172792=CARTESIAN_POINT('Ctrl Pts',(62.5112633589193,5.43505031105863,49.2041469361923));
#172793=CARTESIAN_POINT('Ctrl Pts',(62.9680010973421,6.11945136653108,49.1097604168948));
#172794=CARTESIAN_POINT('Ctrl Pts',(63.2219657960189,6.45345669783525,49.0580132218942));
#172795=CARTESIAN_POINT('Ctrl Pts',(63.5844536915174,6.87376348966324,48.9842977375232));
#172796=CARTESIAN_POINT('Ctrl Pts',(63.6755211219381,6.97516563609575,48.9657874925067));
#172797=CARTESIAN_POINT('Ctrl Pts',(63.8130351868757,7.12223551365012,48.9378153233543));
#172798=CARTESIAN_POINT('Ctrl Pts',(63.8579595653611,7.16936601315166,48.9286738759781));
#172799=CARTESIAN_POINT('Ctrl Pts',(63.9418884873431,7.25574017831345,48.9115847144845));
#172800=CARTESIAN_POINT('Ctrl Pts',(63.980768980659,7.29510509796929,48.9036634249084));
#172801=CARTESIAN_POINT('Ctrl Pts',(64.0785657922458,7.39251549112169,48.8837295587852));
#172802=CARTESIAN_POINT('Ctrl Pts',(64.1378651062253,7.45015389406024,48.8716347212945));
#172803=CARTESIAN_POINT('Ctrl Pts',(64.411617338533,7.70980090357732,48.8157849989339));
#172804=CARTESIAN_POINT('Ctrl Pts',(64.633937889923,7.90295376069808,48.7703915764291));
#172805=CARTESIAN_POINT('Ctrl Pts',(65.2039994328685,8.355997590601,48.6543618629463));
#172806=CARTESIAN_POINT('Ctrl Pts',(65.5605220899802,8.60347392592059,48.5821199313326));
#172807=CARTESIAN_POINT('Ctrl Pts',(66.0373040097512,8.89045490370289,48.4863960877223));
#172808=CARTESIAN_POINT('Ctrl Pts',(66.1441201423704,8.95208296464464,48.465002566873));
#172809=CARTESIAN_POINT('Ctrl Pts',(66.4072739254099,9.09747761472091,48.4124339267184));
#172810=CARTESIAN_POINT('Ctrl Pts',(66.5647318969057,9.17906924168856,48.3810947704945));
#172811=CARTESIAN_POINT('Ctrl Pts',(66.8177909835845,9.30174309763282,48.3309186507373));
#172812=CARTESIAN_POINT('Ctrl Pts',(66.9120334108321,9.34561836260671,48.3122730847958));
#172813=CARTESIAN_POINT('Ctrl Pts',(67.0947067281429,9.42720445646798,48.2762093529906));
#172814=CARTESIAN_POINT('Ctrl Pts',(67.1830334651035,9.46512658565578,48.2588059541097));
#172815=CARTESIAN_POINT('Ctrl Pts',(67.3939087302974,9.55206306608089,48.2173351258885));
#172816=CARTESIAN_POINT('Ctrl Pts',(67.5169013683719,9.59992415779027,48.1932097203439));
#172817=CARTESIAN_POINT('Ctrl Pts',(67.9941691234116,9.7747762603445,48.0998136719632));
#172818=CARTESIAN_POINT('Ctrl Pts',(68.3544683888514,9.88398260549235,48.0297837993292));
#172819=CARTESIAN_POINT('Ctrl Pts',(69.1670658385735,10.0806001285614,47.8724017458725));
#172820=CARTESIAN_POINT('Ctrl Pts',(69.6209786021461,10.1574667226971,47.7848657854983));
#172821=CARTESIAN_POINT('Ctrl Pts',(70.2924683811773,10.2235468767787,47.6548774426344));
#172822=CARTESIAN_POINT('Ctrl Pts',(70.5071330688254,10.2376195699303,47.6132445907046));
#172823=CARTESIAN_POINT('Ctrl Pts',(70.7945972563735,10.247059916598,47.5572647245332));
#172824=CARTESIAN_POINT('Ctrl Pts',(70.8671705467532,10.248642782147,47.5431125370581));
#172825=CARTESIAN_POINT('Ctrl Pts',(70.9900854424749,10.2499684817613,47.5191039792565));
#172826=CARTESIAN_POINT('Ctrl Pts',(71.0404220177089,10.2501265509135,47.5092605390517));
#172827=CARTESIAN_POINT('Ctrl Pts',(71.1501771497844,10.2496320682669,47.4877711481412));
#172828=CARTESIAN_POINT('Ctrl Pts',(71.2095916633332,10.2488280277085,47.4761217045659));
#172829=CARTESIAN_POINT('Ctrl Pts',(71.3893848618278,10.2447713860716,47.4408253099966));
#172830=CARTESIAN_POINT('Ctrl Pts',(71.5097081370372,10.2398526698203,47.4171438904982));
#172831=CARTESIAN_POINT('Ctrl Pts',(72.2218386726454,10.1976779810612,47.2767165395426));
#172832=CARTESIAN_POINT('Ctrl Pts',(72.8093933424619,10.1093534062066,47.1598201382924));
#172833=CARTESIAN_POINT('Ctrl Pts',(73.6319342458763,9.9088108181989,46.9964779357895));
#172834=CARTESIAN_POINT('Ctrl Pts',(73.8756408755417,9.83939181932036,46.94811084902));
#172835=CARTESIAN_POINT('Ctrl Pts',(74.2985017592521,9.70122238367633,46.8643160550229));
#172836=CARTESIAN_POINT('Ctrl Pts',(74.478777627586,9.6364903737699,46.8286337095392));
#172837=CARTESIAN_POINT('Ctrl Pts',(74.7564952780868,9.527611975536,46.773738141561));
#172838=CARTESIAN_POINT('Ctrl Pts',(74.8552364332674,9.48705641825705,46.7542349072487));
#172839=CARTESIAN_POINT('Ctrl Pts',(75.0408825763764,9.40729442242711,46.7175929386025));
#172840=CARTESIAN_POINT('Ctrl Pts',(75.1279098115385,9.36841538698938,46.7004271791125));
#172841=CARTESIAN_POINT('Ctrl Pts',(75.326549230017,9.2762347133933,46.6612696420596));
#172842=CARTESIAN_POINT('Ctrl Pts',(75.43776808863,9.22208740524928,46.6393624207116));
#172843=CARTESIAN_POINT('Ctrl Pts',(75.821807746146,9.02620659869566,46.5637616523185));
#172844=CARTESIAN_POINT('Ctrl Pts',(76.0892452106587,8.87387365141424,46.5112004349527));
#172845=CARTESIAN_POINT('Ctrl Pts',(76.3787138015798,8.6908378026982,46.4542731138968));
#172846=CARTESIAN_POINT('Ctrl Pts',(76.4078917222599,8.67217584096392,46.4485344420631));
#172847=CARTESIAN_POINT('Ctrl Pts',(76.7974269107242,8.42017968097085,46.3719114593987));
#172848=CARTESIAN_POINT('Ctrl Pts',(77.1429246859792,8.16385253383278,46.3038580152475));
#172849=CARTESIAN_POINT('Ctrl Pts',(77.5805623123211,7.79343683031798,46.216773717417));
#172850=CARTESIAN_POINT('Ctrl Pts',(77.6878976081256,7.69858906245689,46.1953363510994));
#172851=CARTESIAN_POINT('Ctrl Pts',(77.8718332748722,7.52893390483562,46.1584142256097));
#172852=CARTESIAN_POINT('Ctrl Pts',(77.9493185650653,7.45514875292869,46.1427997842708));
#172853=CARTESIAN_POINT('Ctrl Pts',(78.0682280501083,7.33825333994719,46.118724105806));
#172854=CARTESIAN_POINT('Ctrl Pts',(78.1104567232221,7.29599601915857,46.1101509572733));
#172855=CARTESIAN_POINT('Ctrl Pts',(78.1880223212825,7.21698660172601,46.0943568138957));
#172856=CARTESIAN_POINT('Ctrl Pts',(78.2234594561265,7.18033851698227,46.0871222645864));
#172857=CARTESIAN_POINT('Ctrl Pts',(78.3209263338557,7.0780016391432,46.0671749591857));
#172858=CARTESIAN_POINT('Ctrl Pts',(78.3823628801202,7.01173804498451,46.054545300444));
#172859=CARTESIAN_POINT('Ctrl Pts',(78.7649939098359,6.58778962157157,45.975564355603));
#172860=CARTESIAN_POINT('Ctrl Pts',(79.0615942226491,6.20804358575574,45.912903385635));
#172861=CARTESIAN_POINT('Ctrl Pts',(79.5639827856835,5.46144651148204,45.8051828536768));
#172862=CARTESIAN_POINT('Ctrl Pts',(79.7761220919811,5.10025123361291,45.7589905416315));
#172863=CARTESIAN_POINT('Ctrl Pts',(80.0331196361417,4.59430834000802,45.7022853161928));
#172864=CARTESIAN_POINT('Ctrl Pts',(80.0975399315968,4.46039098638363,45.6879917243836));
#172865=CARTESIAN_POINT('Ctrl Pts',(80.2003085921771,4.23438069341351,45.6650548598083));
#172866=CARTESIAN_POINT('Ctrl Pts',(80.2402449340321,4.14306684354109,45.6561035219449));
#172867=CARTESIAN_POINT('Ctrl Pts',(80.3134291800371,3.96891087806438,45.6396251955236));
#172868=CARTESIAN_POINT('Ctrl Pts',(80.3469360602918,3.88619247319618,45.6320479987425));
#172869=CARTESIAN_POINT('Ctrl Pts',(80.4321304936543,3.66779165715199,45.612691673642));
#172870=CARTESIAN_POINT('Ctrl Pts',(80.4820506691022,3.53141165359496,45.6012556823369));
#172871=CARTESIAN_POINT('Ctrl Pts',(80.7368300530287,2.7872369657385,45.5423178865471));
#172872=CARTESIAN_POINT('Ctrl Pts',(80.8880433326182,2.16179213325184,45.5052564431246));
#172873=CARTESIAN_POINT('Ctrl Pts',(81.0177905568147,1.26957861901464,45.4675592930169));
#172874=CARTESIAN_POINT('Ctrl Pts',(81.0454722871623,1.01185257793934,45.4583846578112));
#172875=CARTESIAN_POINT('Ctrl Pts',(81.0711989342334,0.642344008651511,
45.4474748180109));
#172876=CARTESIAN_POINT('Ctrl Pts',(81.0771397391497,0.531250048812504,
45.4444827765273));
#172877=CARTESIAN_POINT('Ctrl Pts',(81.0845918423905,0.331668168683652,
45.4396025589623));
#172878=CARTESIAN_POINT('Ctrl Pts',(81.086760798445,0.243218453805301,45.4376139966441));
#172879=CARTESIAN_POINT('Ctrl Pts',(81.0884256696655,0.100950184485942,
45.4346853926625));
#172880=CARTESIAN_POINT('Ctrl Pts',(81.0886360100655,0.04714661561525,45.4336398879946));
#172881=CARTESIAN_POINT('Ctrl Pts',(81.0882122583059,-0.0618632610171435,
45.4316444081162));
#172882=CARTESIAN_POINT('Ctrl Pts',(81.0875560498093,-0.117067658097874,
45.4306977765404));
#172883=CARTESIAN_POINT('Ctrl Pts',(81.0845637515103,-0.267561747610409,
45.4282950839628));
#172884=CARTESIAN_POINT('Ctrl Pts',(81.0813537485863,-0.362830713523165,
45.4269686598293));
#172885=CARTESIAN_POINT('Ctrl Pts',(81.0545999128149,-0.926020272110199,
45.420318260754));
#172886=CARTESIAN_POINT('Ctrl Pts',(81.000684497016,-1.39200765978234,45.4197044297711));
#172887=CARTESIAN_POINT('Ctrl Pts',(80.8188730207129,-2.37623753026221,
45.4302640098083));
#172888=CARTESIAN_POINT('Ctrl Pts',(80.6821727652902,-2.89146758284856,
45.4430574296226));
#172889=CARTESIAN_POINT('Ctrl Pts',(80.4587877575335,-3.53120381771839,
45.4688826648455));
#172890=CARTESIAN_POINT('Ctrl Pts',(80.4079158694468,-3.66762201686016,
45.474985774153));
#172891=CARTESIAN_POINT('Ctrl Pts',(80.3175218561777,-3.8953021079917,45.4861836488402));
#172892=CARTESIAN_POINT('Ctrl Pts',(80.2795187512148,-3.98715782249328,
45.4909840901436));
#172893=CARTESIAN_POINT('Ctrl Pts',(80.2046232464102,-4.16107626087176,
45.5006135933442));
#172894=CARTESIAN_POINT('Ctrl Pts',(80.1679701650797,-4.24323447034296,
45.505396399953));
#172895=CARTESIAN_POINT('Ctrl Pts',(80.0677971090229,-4.46014958911488,
45.5186458938487));
#172896=CARTESIAN_POINT('Ctrl Pts',(80.002443723957,-4.59401381721281,45.5274688624765));
#172897=CARTESIAN_POINT('Ctrl Pts',(79.751162691718,-5.0817577254656,45.5619919879664));
#172898=CARTESIAN_POINT('Ctrl Pts',(79.5477861608664,-5.42599629684176,
45.5910702757448));
#172899=CARTESIAN_POINT('Ctrl Pts',(79.1277308350556,-6.05103096487884,
45.6524973395758));
#172900=CARTESIAN_POINT('Ctrl Pts',(78.9154748071413,-6.33416543875234,
45.6840531754701));
#172901=CARTESIAN_POINT('Ctrl Pts',(78.6050034727639,-6.70650223929368,
45.7304262038561));
#172902=CARTESIAN_POINT('Ctrl Pts',(78.518948475767,-6.80575444824079,45.7432990708961));
#172903=CARTESIAN_POINT('Ctrl Pts',(78.3636145420426,-6.9780799359613,45.7665340086848));
#172904=CARTESIAN_POINT('Ctrl Pts',(78.2951157155577,-7.05184774857841,
45.7767796490357));
#172905=CARTESIAN_POINT('Ctrl Pts',(78.1849954796973,-7.16697177031707,
45.7932351821164));
#172906=CARTESIAN_POINT('Ctrl Pts',(78.1440827458378,-7.2090108747292,45.7993455669863));
#172907=CARTESIAN_POINT('Ctrl Pts',(78.0661645735939,-7.28770253355853,
45.8109729767454));
#172908=CARTESIAN_POINT('Ctrl Pts',(78.0292359088352,-7.32442985533583,
45.8164796948654));
#172909=CARTESIAN_POINT('Ctrl Pts',(77.9234664203589,-7.42802101044722,
45.8322438236062));
#172910=CARTESIAN_POINT('Ctrl Pts',(77.8539667060724,-7.49419031439474,
45.8425927886614));
#172911=CARTESIAN_POINT('Ctrl Pts',(77.5682993208651,-7.7585728062715,45.8851210559512));
#172912=CARTESIAN_POINT('Ctrl Pts',(77.3446354325167,-7.94830257061248,
45.9184003312349));
#172913=CARTESIAN_POINT('Ctrl Pts',(76.7812530010548,-8.38581214569848,
46.0026037301126));
#172914=CARTESIAN_POINT('Ctrl Pts',(76.4338656154348,-8.62258577781445,
46.0548437426379));
#172915=CARTESIAN_POINT('Ctrl Pts',(75.9684924311167,-8.8991457156002,46.1256443746958));
#172916=CARTESIAN_POINT('Ctrl Pts',(75.8627909874382,-8.95941092458015,
46.1417753481643));
#172917=CARTESIAN_POINT('Ctrl Pts',(75.601515544903,-9.10219761974323,46.1817793704878));
#172918=CARTESIAN_POINT('Ctrl Pts',(75.4448505766269,-9.18257529397102,
46.2058779471163));
#172919=CARTESIAN_POINT('Ctrl Pts',(75.1923206429091,-9.30390972558562,
46.2449075485867));
#172920=CARTESIAN_POINT('Ctrl Pts',(75.0977487456319,-9.34756089790883,
46.2595640749589));
#172921=CARTESIAN_POINT('Ctrl Pts',(74.9139616327435,-9.42896336502099,
46.2881235568065));
#172922=CARTESIAN_POINT('Ctrl Pts',(74.8248421693073,-9.46690960124373,
46.3020063189872));
#172923=CARTESIAN_POINT('Ctrl Pts',(74.6112610035641,-9.55423571487202,
46.3353561484672));
#172924=CARTESIAN_POINT('Ctrl Pts',(74.4863482214221,-9.60242456899424,
46.3549237400397));
#172925=CARTESIAN_POINT('Ctrl Pts',(74.0018405292962,-9.77831688357989,
46.431045166004));
#172926=CARTESIAN_POINT('Ctrl Pts',(73.6362463788273,-9.88794313063175,
46.4889643887945));
#172927=CARTESIAN_POINT('Ctrl Pts',(72.6900682040399,-10.1138034185437,
46.6394991502311));
#172928=CARTESIAN_POINT('Ctrl Pts',(72.1040200846467,-10.199863110892,46.7333637028918));
#172929=CARTESIAN_POINT('Ctrl Pts',(71.3961233553964,-10.2403862161788,
46.8456107995423));
#172930=CARTESIAN_POINT('Ctrl Pts',(71.2783702210663,-10.2450410236952,
46.8642425538667));
#172931=CARTESIAN_POINT('Ctrl Pts',(71.1013799408687,-10.2489068919668,
46.8921642895165));
#172932=CARTESIAN_POINT('Ctrl Pts',(71.0421925221178,-10.2496742327309,
46.9014876775396));
#172933=CARTESIAN_POINT('Ctrl Pts',(70.9321765080428,-10.2501241729304,
46.9187880549125));
#172934=CARTESIAN_POINT('Ctrl Pts',(70.8813516080021,-10.2499448116025,
46.9267683086871));
#172935=CARTESIAN_POINT('Ctrl Pts',(70.7682154402204,-10.2486836542141,
46.9445069059908));
#172936=CARTESIAN_POINT('Ctrl Pts',(70.7059074734182,-10.2474070288422,
46.9542591770138));
#172937=CARTESIAN_POINT('Ctrl Pts',(70.4727739729375,-10.2404518933631,
46.9906926394535));
#172938=CARTESIAN_POINT('Ctrl Pts',(70.3020721738944,-10.2309804072448,
47.0172573077076));
#172939=CARTESIAN_POINT('Ctrl Pts',(69.6109075697902,-10.1748539933539,
47.1245199710389));
#172940=CARTESIAN_POINT('Ctrl Pts',(69.0940392714917,-10.091870712187,47.2040885696753));
#172941=CARTESIAN_POINT('Ctrl Pts',(68.3378409925298,-9.90894490389436,
47.3207241779582));
#172942=CARTESIAN_POINT('Ctrl Pts',(68.0921800517385,-9.83950696932494,
47.3586433244153));
#172943=CARTESIAN_POINT('Ctrl Pts',(67.6659992383484,-9.70129836716088,
47.4245538850417));
#172944=CARTESIAN_POINT('Ctrl Pts',(67.4843369957254,-9.63655111956149,
47.4526897972642));
#172945=CARTESIAN_POINT('Ctrl Pts',(67.204529284537,-9.52765191535149,47.4960996270251));
#172946=CARTESIAN_POINT('Ctrl Pts',(67.1050626524839,-9.48709353734558,
47.5115455581197));
#172947=CARTESIAN_POINT('Ctrl Pts',(66.9180720306105,-9.40733002369934,
47.5406093233296));
#172948=CARTESIAN_POINT('Ctrl Pts',(66.8304237779518,-9.36845264967769,
47.5542435923924));
#172949=CARTESIAN_POINT('Ctrl Pts',(66.6303893284162,-9.2762826114878,47.5853833759914));
#172950=CARTESIAN_POINT('Ctrl Pts',(66.5184013821207,-9.22214485084536,
47.6028338605937));
#172951=CARTESIAN_POINT('Ctrl Pts',(66.1318650337091,-9.02637248821874,
47.6631104716653));
#172952=CARTESIAN_POINT('Ctrl Pts',(65.862753936375,-8.87415475948891,47.7051606732697));
#172953=CARTESIAN_POINT('Ctrl Pts',(65.5747679244819,-8.69334486471779,
47.7501248446212));
#172954=CARTESIAN_POINT('Ctrl Pts',(65.5486983017096,-8.67681035273505,
47.7541947891571));
#172955=CARTESIAN_POINT('Ctrl Pts',(65.1566726098513,-8.42564649642074,
47.8153889121942));
#172956=CARTESIAN_POINT('Ctrl Pts',(64.8058745255349,-8.16761862304484,
47.8700587382125));
#172957=CARTESIAN_POINT('Ctrl Pts',(64.3618560895901,-7.79489198067989,
47.9383709197026));
#172958=CARTESIAN_POINT('Ctrl Pts',(64.2532917614047,-7.6997570588825,47.9549947846071));
#172959=CARTESIAN_POINT('Ctrl Pts',(64.0672715067216,-7.52964245613763,
47.9832936984406));
#172960=CARTESIAN_POINT('Ctrl Pts',(63.9889319965957,-7.45569423181673,
47.9951511011832));
#172961=CARTESIAN_POINT('Ctrl Pts',(63.8687408377713,-7.33859834064117,
48.0132300411273));
#172962=CARTESIAN_POINT('Ctrl Pts',(63.8260902515492,-7.29630875339498,
48.0196225586124));
#172963=CARTESIAN_POINT('Ctrl Pts',(63.7477818472157,-7.21728656679977,
48.0313129081549));
#172964=CARTESIAN_POINT('Ctrl Pts',(63.7120243632958,-7.18065888316707,
48.0366324598717));
#172965=CARTESIAN_POINT('Ctrl Pts',(63.6137404304597,-7.07846387164977,
48.051205179706));
#172966=CARTESIAN_POINT('Ctrl Pts',(63.5517969709913,-7.01232448132923,
48.0603341479518));
#172967=CARTESIAN_POINT('Ctrl Pts',(63.1629037520539,-6.58590725616973,
48.1173268257431));
#172968=CARTESIAN_POINT('Ctrl Pts',(62.86070431903,-6.20322789384647,48.160169970309));
#172969=CARTESIAN_POINT('Ctrl Pts',(62.3519059843458,-5.4553149670522,48.2307302784892));
#172970=CARTESIAN_POINT('Ctrl Pts',(62.1382797499242,-5.09620297619264,
48.2596688955328));
#172971=CARTESIAN_POINT('Ctrl Pts',(61.87880738257,-4.59277142093952,48.2940905470742));
#172972=CARTESIAN_POINT('Ctrl Pts',(61.8135444332031,-4.45913267275824,
48.3026702813829));
#172973=CARTESIAN_POINT('Ctrl Pts',(61.7093099052031,-4.23345325529348,
48.3162413593808));
#172974=CARTESIAN_POINT('Ctrl Pts',(61.6687517275544,-4.14218615668145,
48.3214845925173));
#172975=CARTESIAN_POINT('Ctrl Pts',(61.5897014039152,-3.95711622997738,
48.3316257876471));
#172976=CARTESIAN_POINT('Ctrl Pts',(61.5512534577513,-3.86330619699858,
48.3365168769265));
#172977=CARTESIAN_POINT('Ctrl Pts',(61.4569139993982,-3.62311778127344,
48.3484063768129));
#172978=CARTESIAN_POINT('Ctrl Pts',(61.402952818374,-3.47599465238431,48.3550985570037));
#172979=CARTESIAN_POINT('Ctrl Pts',(61.1945207709509,-2.86515841778187,
48.3804403696506));
#172980=CARTESIAN_POINT('Ctrl Pts',(61.0695872723964,-2.39186309715017,
48.3943840153022));
#172981=CARTESIAN_POINT('Ctrl Pts',(60.913282447589,-1.56823970016767,48.4082143148684));
#172982=CARTESIAN_POINT('Ctrl Pts',(60.8654794912693,-1.2219533567363,48.4109596393889));
#172983=CARTESIAN_POINT('Ctrl Pts',(60.8186903445414,-0.685333999625466,
48.4100457573896));
#172984=CARTESIAN_POINT('Ctrl Pts',(60.8073814968257,-0.49633910944873,
48.4087430698905));
#172985=CARTESIAN_POINT('Ctrl Pts',(60.7989069574862,-0.236577787073999,
48.4055282221811));
#172986=CARTESIAN_POINT('Ctrl Pts',(60.7973195590584,-0.165983077583135,
48.4045102554311));
#172987=CARTESIAN_POINT('Ctrl Pts',(60.7960539259737,-0.0635873302775755,
48.402819863519));
#172988=CARTESIAN_POINT('Ctrl Pts',(60.7958058977463,-0.0317937268324048,
48.4022651036016));
#172989=CARTESIAN_POINT('Ctrl Pts',(60.7957027539178,1.12610920091049E-9,
48.4016801458622));
#172990=CARTESIAN_POINT('Ctrl Pts',(60.7795023650012,-1.31054137042235E-9,
48.3098031747286));
#172991=CARTESIAN_POINT('Ctrl Pts',(60.7795765067117,-0.0228539252004177,
48.310223653247));
#172992=CARTESIAN_POINT('Ctrl Pts',(60.779726332016,-0.0457078558460972,
48.3106331887275));
#172993=CARTESIAN_POINT('Ctrl Pts',(60.7805904389733,-0.133284916798912,
48.3121602353422));
#172994=CARTESIAN_POINT('Ctrl Pts',(60.7818359190101,-0.198002387172251,
48.313200131041));
#172995=CARTESIAN_POINT('Ctrl Pts',(60.7879015251552,-0.409940099125638,
48.3163084488624));
#172996=CARTESIAN_POINT('Ctrl Pts',(60.7952541481782,-0.557075269763786,
48.3179963592047));
#172997=CARTESIAN_POINT('Ctrl Pts',(60.8404923029711,-1.19121275142366,
48.32313819393));
#172998=CARTESIAN_POINT('Ctrl Pts',(60.9095924263722,-1.67539614495611,
48.3215957730452));
#172999=CARTESIAN_POINT('Ctrl Pts',(61.1003678533738,-2.56147117870582,
48.3073380182831));
#173000=CARTESIAN_POINT('Ctrl Pts',(61.2128476043723,-2.96433645223241,
48.2962826415568));
#173001=CARTESIAN_POINT('Ctrl Pts',(61.398553863287,-3.50223277365923,48.2749583044959));
#173002=CARTESIAN_POINT('Ctrl Pts',(61.4510412238349,-3.64414850080823,
48.2686894151225));
#173003=CARTESIAN_POINT('Ctrl Pts',(61.5434753960353,-3.87824169459329,
48.2572693516743));
#173004=CARTESIAN_POINT('Ctrl Pts',(61.5817012772225,-3.97108886448879,
48.2524515988262));
#173005=CARTESIAN_POINT('Ctrl Pts',(61.6609814697912,-4.1559933543047,48.2422774476391));
#173006=CARTESIAN_POINT('Ctrl Pts',(61.7020421679011,-4.2480357948693,48.2369195213534));
#173007=CARTESIAN_POINT('Ctrl Pts',(61.8091920736398,-4.47911947043774,
48.2227253218519));
#173008=CARTESIAN_POINT('Ctrl Pts',(61.8770391485022,-4.61729653443926,
48.2135473656859));
#173009=CARTESIAN_POINT('Ctrl Pts',(62.0341735558332,-4.92007396352988,
48.1919096692745));
#173010=CARTESIAN_POINT('Ctrl Pts',(62.1248900566577,-5.08385006970712,
48.1791737231482));
#173011=CARTESIAN_POINT('Ctrl Pts',(62.4610459019524,-5.65365218217333,
48.1312508599801));
#173012=CARTESIAN_POINT('Ctrl Pts',(62.729773664739,-6.0448432735838,48.0916520591102));
#173013=CARTESIAN_POINT('Ctrl Pts',(63.1818130027412,-6.61407985057535,
48.0243061433485));
#173014=CARTESIAN_POINT('Ctrl Pts',(63.3465240915125,-6.80640192010735,
47.99964841869));
#173015=CARTESIAN_POINT('Ctrl Pts',(63.5726427126616,-7.05137667845077,
47.9658316321619));
#173016=CARTESIAN_POINT('Ctrl Pts',(63.6278321061735,-7.10976894082202,
47.9575805133412));
#173017=CARTESIAN_POINT('Ctrl Pts',(63.7221183976014,-7.2071933640807,47.9434967595932));
#173018=CARTESIAN_POINT('Ctrl Pts',(63.7608563329749,-7.2465745887425,47.93771408191));
#173019=CARTESIAN_POINT('Ctrl Pts',(63.847215518413,-7.33295073186859,47.9248326965077));
#173020=CARTESIAN_POINT('Ctrl Pts',(63.8949813477333,-7.37979336047445,
47.9177138690443));
#173021=CARTESIAN_POINT('Ctrl Pts',(64.0484015995225,-7.52731112026731,
47.8948597582135));
#173022=CARTESIAN_POINT('Ctrl Pts',(64.1557422862191,-7.62616921198454,
47.8788860377963));
#173023=CARTESIAN_POINT('Ctrl Pts',(64.434965097946,-7.87244812078303,47.8373141111808));
#173024=CARTESIAN_POINT('Ctrl Pts',(64.6096757214068,-8.01646917727984,
47.811283157596));
#173025=CARTESIAN_POINT('Ctrl Pts',(65.2756754166724,-8.52913912498367,
47.7117002912856));
#173026=CARTESIAN_POINT('Ctrl Pts',(65.7948079728654,-8.85851727020266,
47.6333162159989));
#173027=CARTESIAN_POINT('Ctrl Pts',(66.4589108091594,-9.19974337699546,
47.5311669373846));
#173028=CARTESIAN_POINT('Ctrl Pts',(66.5791222396116,-9.25852181227756,
47.512610830095));
#173029=CARTESIAN_POINT('Ctrl Pts',(66.7882505634683,-9.35567628070652,
47.4802147169227));
#173030=CARTESIAN_POINT('Ctrl Pts',(66.8766319308123,-9.39519920322599,
47.4664890813355));
#173031=CARTESIAN_POINT('Ctrl Pts',(67.0613433228089,-9.47462864696736,
47.4377330021541));
#173032=CARTESIAN_POINT('Ctrl Pts',(67.1577488796595,-9.51432418937986,
47.4226853845674));
#173033=CARTESIAN_POINT('Ctrl Pts',(67.4181775626633,-9.61685917212951,
47.3819354344702));
#173034=CARTESIAN_POINT('Ctrl Pts',(67.5832258774511,-9.6769025253189,47.3560038010921));
#173035=CARTESIAN_POINT('Ctrl Pts',(68.5231633857349,-9.99122789578273,
47.2078059431948));
#173036=CARTESIAN_POINT('Ctrl Pts',(69.3242013150811,-10.1544651041615,
47.0792845889112));
#173037=CARTESIAN_POINT('Ctrl Pts',(70.300930718175,-10.231830670227,46.9240490764136));
#173038=CARTESIAN_POINT('Ctrl Pts',(70.4660935905049,-10.2407978935956,
46.8978590670135));
#173039=CARTESIAN_POINT('Ctrl Pts',(70.6931994158643,-10.2474851876242,
46.8619867841994));
#173040=CARTESIAN_POINT('Ctrl Pts',(70.7550012084679,-10.2487318002441,
46.8522392027246));
#173041=CARTESIAN_POINT('Ctrl Pts',(70.8675396507649,-10.2499585566647,
46.8345194279285));
#173042=CARTESIAN_POINT('Ctrl Pts',(70.9182714022317,-10.2501257164091,
46.826542739719));
#173043=CARTESIAN_POINT('Ctrl Pts',(71.0285527484569,-10.2496504113759,
46.8092292506485));
#173044=CARTESIAN_POINT('Ctrl Pts',(71.0880997877005,-10.2488622430712,
46.7998969368915));
#173045=CARTESIAN_POINT('Ctrl Pts',(71.2673852523826,-10.2448886739982,
46.7718423936476));
#173046=CARTESIAN_POINT('Ctrl Pts',(71.3870850143546,-10.2400853917182,
46.7531700244064));
#173047=CARTESIAN_POINT('Ctrl Pts',(71.676335623008,-10.2232755867876,46.7081560565961));
#173048=CARTESIAN_POINT('Ctrl Pts',(71.845734425581,-10.2090980345999,46.6818828075499));
#173049=CARTESIAN_POINT('Ctrl Pts',(72.6720047468749,-10.1187230726835,
46.5539914500252));
#173050=CARTESIAN_POINT('Ctrl Pts',(73.3209135840049,-9.98190993035056,
46.4542482860221));
#173051=CARTESIAN_POINT('Ctrl Pts',(74.1468086644587,-9.72042310977867,
46.3265632297974));
#173052=CARTESIAN_POINT('Ctrl Pts',(74.3398113943093,-9.65276896211922,
46.2966799600512));
#173053=CARTESIAN_POINT('Ctrl Pts',(74.6338574990111,-9.53950702820404,
46.2510703679023));
#173054=CARTESIAN_POINT('Ctrl Pts',(74.7364095851474,-9.49804989607294,
46.2351481012261));
#173055=CARTESIAN_POINT('Ctrl Pts',(74.9260928779884,-9.41770454404923,
46.2056700648824));
#173056=CARTESIAN_POINT('Ctrl Pts',(75.013392237616,-9.37925356836793,46.1920920337707));
#173057=CARTESIAN_POINT('Ctrl Pts',(75.2103546523868,-9.28913706849641,
46.1614347658374));
#173058=CARTESIAN_POINT('Ctrl Pts',(75.3196639282275,-9.23671762433628,
46.1444043088575));
#173059=CARTESIAN_POINT('Ctrl Pts',(75.6864127941312,-9.05262898091877,
46.0872217634099));
#173060=CARTESIAN_POINT('Ctrl Pts',(75.9392036797019,-8.91181887450907,
46.0477308214453));
#173061=CARTESIAN_POINT('Ctrl Pts',(76.6767679350914,-8.45842479205521,
45.932554552414));
#173062=CARTESIAN_POINT('Ctrl Pts',(77.1415427806757,-8.11484095676641,
45.8599950243703));
#173063=CARTESIAN_POINT('Ctrl Pts',(77.6874925401928,-7.6344926605228,45.7764740508071));
#173064=CARTESIAN_POINT('Ctrl Pts',(77.7975887495404,-7.53324960471619,
45.7597325125078));
#173065=CARTESIAN_POINT('Ctrl Pts',(77.9541122691709,-7.38284642989016,
45.7361247359689));
#173066=CARTESIAN_POINT('Ctrl Pts',(78.0023057619755,-7.3356123599928,45.7288836468148));
#173067=CARTESIAN_POINT('Ctrl Pts',(78.0890267165177,-7.24892221062687,
45.7159099220155));
#173068=CARTESIAN_POINT('Ctrl Pts',(78.1277061043518,-7.20962787585481,
45.7101446249022));
#173069=CARTESIAN_POINT('Ctrl Pts',(78.2212976394699,-7.11300224490283,
45.6962453540441));
#173070=CARTESIAN_POINT('Ctrl Pts',(78.2758699332725,-7.05533670756435,
45.688183904982));
#173071=CARTESIAN_POINT('Ctrl Pts',(78.5019693615782,-6.81079866175594,
45.6549504512769));
#173072=CARTESIAN_POINT('Ctrl Pts',(78.6672957519092,-6.61814177749665,
45.6310570574329));
#173073=CARTESIAN_POINT('Ctrl Pts',(79.0218762056326,-6.17254607224269,
45.5805028126085));
#173074=CARTESIAN_POINT('Ctrl Pts',(79.2070040643538,-5.91656513488964,
45.5546030126715));
#173075=CARTESIAN_POINT('Ctrl Pts',(79.5963033328536,-5.32250060373993,
45.5009455273585));
#173076=CARTESIAN_POINT('Ctrl Pts',(79.7934587919346,-4.98031078968498,
45.4743623312877));
#173077=CARTESIAN_POINT('Ctrl Pts',(80.0300897822527,-4.50900087827087,
45.4431062222859));
#173078=CARTESIAN_POINT('Ctrl Pts',(80.0873002315768,-4.38935747080625,
45.4356120499775));
#173079=CARTESIAN_POINT('Ctrl Pts',(80.1824841991048,-4.18003291620887,
45.4232544199594));
#173080=CARTESIAN_POINT('Ctrl Pts',(80.2215198621933,-4.09086411410551,
45.4182223792946));
#173081=CARTESIAN_POINT('Ctrl Pts',(80.3004557227389,-3.90338492548337,
45.4081250951556));
#173082=CARTESIAN_POINT('Ctrl Pts',(80.3401146218821,-3.80498337922563,
45.4030979567488));
#173083=CARTESIAN_POINT('Ctrl Pts',(80.443696349993,-3.53611623083272,45.3901014555969));
#173084=CARTESIAN_POINT('Ctrl Pts',(80.5046517516113,-3.36452678420184,
45.3826032536093));
#173085=CARTESIAN_POINT('Ctrl Pts',(80.666437599643,-2.86795784159947,45.3632047048561));
#173086=CARTESIAN_POINT('Ctrl Pts',(80.7558440426525,-2.53944392706786,
45.3531400102567));
#173087=CARTESIAN_POINT('Ctrl Pts',(80.9560349573233,-1.62961664659101,
45.3331920979815));
#173088=CARTESIAN_POINT('Ctrl Pts',(81.0335854643708,-1.04224134504529,
45.3289171756853));
#173089=CARTESIAN_POINT('Ctrl Pts',(81.0654036824948,-0.357498360043161,
45.3354955571808));
#173090=CARTESIAN_POINT('Ctrl Pts',(81.0685020617527,-0.263428123826516,
45.3366519086648));
#173091=CARTESIAN_POINT('Ctrl Pts',(81.0713983569315,-0.114381144895917,
45.3388958921633));
#173092=CARTESIAN_POINT('Ctrl Pts',(81.0720330285175,-0.0594234856816828,
45.3398119639789));
#173093=CARTESIAN_POINT('Ctrl Pts',(81.0724330554443,0.0495516206740589,
45.3418072576274));
#173094=CARTESIAN_POINT('Ctrl Pts',(81.0722131288569,0.103567233911748,
45.3428834527681));
#173095=CARTESIAN_POINT('Ctrl Pts',(81.0705168013786,0.247095979922438,
45.3459714278223));
#173096=CARTESIAN_POINT('Ctrl Pts',(81.0683094374653,0.336592762322675,
45.348132978835));
#173097=CARTESIAN_POINT('Ctrl Pts',(81.0487431222813,0.85794588733079,45.3620684487564));
#173098=CARTESIAN_POINT('Ctrl Pts',(81.0057467068751,1.28827508982859,45.3789321079492));
#173099=CARTESIAN_POINT('Ctrl Pts',(80.8451122782092,2.2716567509323,45.4286899802784));
#173100=CARTESIAN_POINT('Ctrl Pts',(80.7088560351132,2.82010142128822,45.4648015379234));
#173101=CARTESIAN_POINT('Ctrl Pts',(80.4801141151906,3.49803540474294,45.5195318653395));
#173102=CARTESIAN_POINT('Ctrl Pts',(80.4284144257382,3.64076963704903,45.531651699219));
#173103=CARTESIAN_POINT('Ctrl Pts',(80.3373501983133,3.87581996887589,45.5526078744458));
#173104=CARTESIAN_POINT('Ctrl Pts',(80.2997477373566,3.9688172657719,45.5611640196031));
#173105=CARTESIAN_POINT('Ctrl Pts',(80.2218120562113,4.15373527800768,45.5787119087024));
#173106=CARTESIAN_POINT('Ctrl Pts',(80.18148057449,4.24564472473005,45.5877030919483));
#173107=CARTESIAN_POINT('Ctrl Pts',(80.0764314682381,4.47581208897823,45.6109071506257));
#173108=CARTESIAN_POINT('Ctrl Pts',(80.0099762993214,4.61322156272542,45.6253952272206));
#173109=CARTESIAN_POINT('Ctrl Pts',(79.8561674963407,4.91395000955456,45.6585449214192));
#173110=CARTESIAN_POINT('Ctrl Pts',(79.7674132832127,5.07646659247095,45.6774298717117));
#173111=CARTESIAN_POINT('Ctrl Pts',(79.4412025781533,5.63712244572356,45.7461175224448));
#173112=CARTESIAN_POINT('Ctrl Pts',(79.1813617184851,6.02110686093215,45.7995737219165));
#173113=CARTESIAN_POINT('Ctrl Pts',(78.7349486830617,6.59295783336683,45.8906457718601));
#173114=CARTESIAN_POINT('Ctrl Pts',(78.5653234364098,6.79372679985372,45.9251128520068));
#173115=CARTESIAN_POINT('Ctrl Pts',(78.3336419229699,7.0473711167071,45.9722242433797));
#173116=CARTESIAN_POINT('Ctrl Pts',(78.278314298823,7.10650961381684,45.9834774628389));
#173117=CARTESIAN_POINT('Ctrl Pts',(78.1841694864696,7.20476075566679,46.0026386278442));
#173118=CARTESIAN_POINT('Ctrl Pts',(78.1457220480855,7.2442375080533,46.0104674737798));
#173119=CARTESIAN_POINT('Ctrl Pts',(78.0605077734062,7.33032133851806,46.0278293798582));
#173120=CARTESIAN_POINT('Ctrl Pts',(78.0136071090963,7.37678551210205,46.0373910596379));
#173121=CARTESIAN_POINT('Ctrl Pts',(77.8645888000426,7.52156273312126,46.0677825675462));
#173122=CARTESIAN_POINT('Ctrl Pts',(77.7608963602562,7.61816022583092,46.0889459516062));
#173123=CARTESIAN_POINT('Ctrl Pts',(77.4935181638413,7.85695106124518,46.1435002377902));
#173124=CARTESIAN_POINT('Ctrl Pts',(77.327278905375,7.99606068848886,46.1774025615863));
#173125=CARTESIAN_POINT('Ctrl Pts',(76.6592271683617,8.51938645610865,46.3133102269626));
#173126=CARTESIAN_POINT('Ctrl Pts',(76.1268313275312,8.86077207538095,46.4208209273963));
#173127=CARTESIAN_POINT('Ctrl Pts',(75.462403552005,9.20284155474791,46.5530073484307));
#173128=CARTESIAN_POINT('Ctrl Pts',(75.3574780453199,9.25454314075059,46.5738307837529));
#173129=CARTESIAN_POINT('Ctrl Pts',(75.1646140895626,9.34538758918787,46.6120120458151));
#173130=CARTESIAN_POINT('Ctrl Pts',(75.0769653843334,9.3851291014514,46.6293291046125));
#173131=CARTESIAN_POINT('Ctrl Pts',(74.8958182444689,9.46411517545122,46.6650486821665));
#173132=CARTESIAN_POINT('Ctrl Pts',(74.8022693298654,9.50321325397977,46.6834573866458));
#173133=CARTESIAN_POINT('Ctrl Pts',(74.55725120225,9.6012396066345,46.731577959967));
#173134=CARTESIAN_POINT('Ctrl Pts',(74.4049243066894,9.6578862018402,46.7614013117085));
#173135=CARTESIAN_POINT('Ctrl Pts',(74.0620045155435,9.77591051812833,46.8283565648095));
#173136=CARTESIAN_POINT('Ctrl Pts',(73.8708186192574,9.83530448577064,46.865561653675));
#173137=CARTESIAN_POINT('Ctrl Pts',(73.1665268381982,10.0309318259124,47.0022829474601));
#173138=CARTESIAN_POINT('Ctrl Pts',(72.6447153605288,10.1316131573217,47.1028989262433));
#173139=CARTESIAN_POINT('Ctrl Pts',(71.8729498075118,10.217053602988,47.2522040395169));
#173140=CARTESIAN_POINT('Ctrl Pts',(71.6274133368779,10.234991285751,47.2997855656282));
#173141=CARTESIAN_POINT('Ctrl Pts',(71.304819022534,10.2464759571301,47.362585122641));
#173142=CARTESIAN_POINT('Ctrl Pts',(71.2280947672074,10.2483126486633,47.3775423261758));
#173143=CARTESIAN_POINT('Ctrl Pts',(71.1009233288507,10.2498746063893,47.4023767836586));
#173144=CARTESIAN_POINT('Ctrl Pts',(71.0504825350468,10.2501077034053,47.4122382398805));
#173145=CARTESIAN_POINT('Ctrl Pts',(70.9428405032955,10.2497804659859,47.4333090402214));
#173146=CARTESIAN_POINT('Ctrl Pts',(70.8856424746946,10.2491095297945,47.4445208632596));
#173147=CARTESIAN_POINT('Ctrl Pts',(70.7198533539539,10.2457237335422,47.4770582848146));
#173148=CARTESIAN_POINT('Ctrl Pts',(70.611302479733,10.2417137813799,47.498411763524));
#173149=CARTESIAN_POINT('Ctrl Pts',(70.3547050221152,10.2279909974161,47.5489798691584));
#173150=CARTESIAN_POINT('Ctrl Pts',(70.206769271889,10.2167300939211,47.5782061388832));
#173151=CARTESIAN_POINT('Ctrl Pts',(69.59759798258,10.1565221055004,47.6987496720323));
#173152=CARTESIAN_POINT('Ctrl Pts',(69.1397770362672,10.0784273250427,47.7897815199368));
#173153=CARTESIAN_POINT('Ctrl Pts',(68.3282021921214,9.88042003111095,47.9509456965582));
#173154=CARTESIAN_POINT('Ctrl Pts',(67.9725823638028,9.77215906398969,48.0214959853037));
#173155=CARTESIAN_POINT('Ctrl Pts',(67.5002261775576,9.59885585308983,48.1149582809414));
#173156=CARTESIAN_POINT('Ctrl Pts',(67.3777217985953,9.55113345464636,48.1391757396126));
#173157=CARTESIAN_POINT('Ctrl Pts',(67.1673956328049,9.46436065962865,48.1807164467912));
#173158=CARTESIAN_POINT('Ctrl Pts',(67.0791430534159,9.42644795762594,48.1981351450922));
#173159=CARTESIAN_POINT('Ctrl Pts',(66.8963717601802,9.34478028907606,48.2341865470601));
#173160=CARTESIAN_POINT('Ctrl Pts',(66.8019588753419,9.30080693839525,48.2527964444137));
#173161=CARTESIAN_POINT('Ctrl Pts',(66.5477857521161,9.17754497026199,48.302867360851));
#173162=CARTESIAN_POINT('Ctrl Pts',(66.3893879552261,9.09541895339749,48.3340382871065));
#173163=CARTESIAN_POINT('Ctrl Pts',(65.8623604432592,8.80400872937472,48.4376981096682));
#173164=CARTESIAN_POINT('Ctrl Pts',(65.5045247173482,8.57538502364424,48.5079726220249));
#173165=CARTESIAN_POINT('Ctrl Pts',(64.8404989780704,8.08925542286462,48.6389697326557));
#173166=CARTESIAN_POINT('Ctrl Pts',(64.5330668281248,7.83484634717865,48.6999045323923));
#173167=CARTESIAN_POINT('Ctrl Pts',(64.1708356628121,7.49692398147681,48.7727180106483));
#173168=CARTESIAN_POINT('Ctrl Pts',(64.1013176395154,7.43018282468968,48.7867430798592));
#173169=CARTESIAN_POINT('Ctrl Pts',(63.9917481908598,7.32192982248355,48.8089445196392));
#173170=CARTESIAN_POINT('Ctrl Pts',(63.951086108794,7.28106182924346,48.8172054779518));
#173171=CARTESIAN_POINT('Ctrl Pts',(63.8686903595205,7.1968168791224,48.8339938244213));
#173172=CARTESIAN_POINT('Ctrl Pts',(63.8269896091492,7.15341031518989,48.8425164414961));
#173173=CARTESIAN_POINT('Ctrl Pts',(63.710660762785,7.03013627658631,48.8663599065718));
#173174=CARTESIAN_POINT('Ctrl Pts',(63.6369246993532,6.94941400674899,48.8815544183621));
#173175=CARTESIAN_POINT('Ctrl Pts',(63.4666498777151,6.75683149706457,48.9168118329063));
#173176=CARTESIAN_POINT('Ctrl Pts',(63.3712066905908,6.64400505344512,48.9367083126948));
#173177=CARTESIAN_POINT('Ctrl Pts',(62.9872207515609,6.16944616795585,49.0172253903589));
#173178=CARTESIAN_POINT('Ctrl Pts',(62.7207879085076,5.78992719006603,49.0742120869994));
#173179=CARTESIAN_POINT('Ctrl Pts',(62.3220330195843,5.1309880476925,49.1606714854087));
#173180=CARTESIAN_POINT('Ctrl Pts',(62.175076564144,4.86160630276654,49.1928830293485));
#173181=CARTESIAN_POINT('Ctrl Pts',(61.9854827624297,4.47379724987402,49.2348784796164));
#173182=CARTESIAN_POINT('Ctrl Pts',(61.9327210855891,4.36071964276109,49.2466222266294));
#173183=CARTESIAN_POINT('Ctrl Pts',(61.8428315735787,4.15858330130247,49.2667331614468));
#173184=CARTESIAN_POINT('Ctrl Pts',(61.8048822860286,4.06992278890669,49.2752597384238));
#173185=CARTESIAN_POINT('Ctrl Pts',(61.726966573758,3.8806073417182,49.2928463471193));
#173186=CARTESIAN_POINT('Ctrl Pts',(61.6873269232175,3.7798248783761,49.3018427562414));
#173187=CARTESIAN_POINT('Ctrl Pts',(61.5807314244082,3.49579852618635,49.3261831395961));
#173188=CARTESIAN_POINT('Ctrl Pts',(61.5173425880186,3.311207621457,49.3408353891317));
#173189=CARTESIAN_POINT('Ctrl Pts',(61.3820222761095,2.87765594773114,49.3726064190893));
#173190=CARTESIAN_POINT('Ctrl Pts',(61.3141143725114,2.62752498594417,49.3889544822805));
#173191=CARTESIAN_POINT('Ctrl Pts',(61.1886093822549,2.08575666178515,49.4203178232803));
#173192=CARTESIAN_POINT('Ctrl Pts',(61.1340113166221,1.79363551635217,49.4347771311325));
#173193=CARTESIAN_POINT('Ctrl Pts',(61.0434859330599,1.15967815393985,49.461271835961));
#173194=CARTESIAN_POINT('Ctrl Pts',(61.0118289147671,0.817566344443593,
49.472565466228));
#173195=CARTESIAN_POINT('Ctrl Pts',(60.9930270032638,0.37617628195623,49.4837164374098));
#173196=CARTESIAN_POINT('Ctrl Pts',(60.9902398662939,0.277849304918228,
49.485983528557));
#173197=CARTESIAN_POINT('Ctrl Pts',(60.988067133047,0.123669582752043,49.4892119583869));
#173198=CARTESIAN_POINT('Ctrl Pts',(60.9877318234734,0.0678392566848939,
49.4903139558446));
#173199=CARTESIAN_POINT('Ctrl Pts',(60.9878565297257,0.00800513799957859,
49.4914248599193));
#173200=CARTESIAN_POINT('Ctrl Pts',(60.9878671932475,0.00400256564559759,
49.4914988370101));
#173201=CARTESIAN_POINT('Ctrl Pts',(60.9878801781973,-3.30742432695422E-11,
49.4915724783198));
#173202=CARTESIAN_POINT('Origin',(69.7358040552328,8.67361737988404E-16,
40.0761166693274));
#173203=CARTESIAN_POINT('',(62.9451177993176,1.47451495458029E-14,41.4621534271586));
#173204=CARTESIAN_POINT('',(66.3565919271274,-6.,40.860618494437));
#173205=CARTESIAN_POINT('Ctrl Pts',(62.9451177993323,1.18985499391726E-10,
41.4621534276372));
#173206=CARTESIAN_POINT('Ctrl Pts',(64.8245030414636,-2.99999999999997,
42.1461937170664));
#173207=CARTESIAN_POINT('Ctrl Pts',(66.3565919272773,-6.00000000011892,
40.8606184948917));
#173208=CARTESIAN_POINT('',(73.179540182747,-6.,39.6575486289937));
#173209=CARTESIAN_POINT('Ctrl Pts',(66.3565919270745,-5.99999999999999,
40.8606184949275));
#173210=CARTESIAN_POINT('Ctrl Pts',(69.9417142331783,-6.00000000000001,
41.2438913179839));
#173211=CARTESIAN_POINT('Ctrl Pts',(73.1795401829645,-6.00000000000002,
39.6575486294364));
#173212=CARTESIAN_POINT('',(76.5910143105568,4.44197482702742E-16,39.056013696272));
#173213=CARTESIAN_POINT('Ctrl Pts',(73.1795401827616,-6.00000000011894,
39.6575486294722));
#173214=CARTESIAN_POINT('Ctrl Pts',(75.058925424893,-2.99999999999999,40.3415889189015));
#173215=CARTESIAN_POINT('Ctrl Pts',(76.5910143107067,1.1897463431604E-10,
39.0560136967267));
#173216=CARTESIAN_POINT('',(76.8756602645714,-2.05071913934279E-17,38.8171673812424));
#173217=CARTESIAN_POINT('',(76.8756602645714,-2.05071913934274E-17,38.8171673812424));
#173218=CARTESIAN_POINT('Origin',(69.7358040552328,8.67361737988404E-16,
40.0761166693274));
#173219=CARTESIAN_POINT('',(73.179540182747,6.,39.6575486289937));
#173220=CARTESIAN_POINT('Ctrl Pts',(76.5910143107067,-1.18906507354984E-10,
39.0560136967267));
#173221=CARTESIAN_POINT('Ctrl Pts',(75.058925424893,3.00000000000003,40.3415889189014));
#173222=CARTESIAN_POINT('Ctrl Pts',(73.1795401827617,6.00000000011895,39.6575486294722));
#173223=CARTESIAN_POINT('',(66.3565919271274,6.,40.860618494437));
#173224=CARTESIAN_POINT('Ctrl Pts',(73.1795401829645,6.,39.6575486294364));
#173225=CARTESIAN_POINT('Ctrl Pts',(69.9417142331783,6.00000000000001,41.2438913179839));
#173226=CARTESIAN_POINT('Ctrl Pts',(66.3565919270744,6.00000000000001,40.8606184949274));
#173227=CARTESIAN_POINT('Ctrl Pts',(66.3565919272774,6.0000000001189,40.8606184948917));
#173228=CARTESIAN_POINT('Ctrl Pts',(64.8245030414637,2.99999999999997,42.1461937170664));
#173229=CARTESIAN_POINT('Ctrl Pts',(62.9451177993323,-1.18964943843131E-10,
41.4621534276372));
#173230=CARTESIAN_POINT('Origin',(69.7358040552328,0.,40.0761166693274));
#173231=CARTESIAN_POINT('',(64.637845022461,-7.86451166255212,49.0198937666656));
#173232=CARTESIAN_POINT('Ctrl Pts',(60.9878801781973,-3.30742432695422E-11,
49.4915724783198));
#173233=CARTESIAN_POINT('Ctrl Pts',(60.9880401713394,-0.0493173303693729,
49.4924798445168));
#173234=CARTESIAN_POINT('Ctrl Pts',(60.9885525976134,-0.0986336473097226,
49.4933362314723));
#173235=CARTESIAN_POINT('Ctrl Pts',(60.9909257253593,-0.233976944592225,
49.4955439724581));
#173236=CARTESIAN_POINT('Ctrl Pts',(60.9935061966073,-0.31998919131596,
49.4967889330294));
#173237=CARTESIAN_POINT('Ctrl Pts',(61.001704578084,-0.513045452919115,
49.4992170694476));
#173238=CARTESIAN_POINT('Ctrl Pts',(61.0079122741947,-0.620055759686851,
49.500309829454));
#173239=CARTESIAN_POINT('Ctrl Pts',(61.0336081579724,-0.969346204667657,
49.5030194112285));
#173240=CARTESIAN_POINT('Ctrl Pts',(61.0599480389006,-1.21104866590326,
49.5035425669253));
#173241=CARTESIAN_POINT('Ctrl Pts',(61.1922679292548,-2.1261924181685,49.5000167941384));
#173242=CARTESIAN_POINT('Ctrl Pts',(61.3558488408635,-2.78950458864437,
49.4859063527375));
#173243=CARTESIAN_POINT('Ctrl Pts',(61.6293995057569,-3.56328691890951,
49.4540514957178));
#173244=CARTESIAN_POINT('Ctrl Pts',(61.6785649297539,-3.69393067546807,
49.4481242973407));
#173245=CARTESIAN_POINT('Ctrl Pts',(61.766486128001,-3.91401106741436,49.4371998973908));
#173246=CARTESIAN_POINT('Ctrl Pts',(61.8039016441018,-4.00397473164329,
49.4324624103401));
#173247=CARTESIAN_POINT('Ctrl Pts',(61.8835893431142,-4.18822590447127,
49.422197881793));
#173248=CARTESIAN_POINT('Ctrl Pts',(61.9260138406176,-4.2824338436548,49.4166409609042));
#173249=CARTESIAN_POINT('Ctrl Pts',(62.0410890950622,-4.52810486397312,
49.4013386018796));
#173250=CARTESIAN_POINT('Ctrl Pts',(62.1160134027525,-4.678440273996,49.3911514393713));
#173251=CARTESIAN_POINT('Ctrl Pts',(62.2634238141401,-4.95703732795004,
49.3707333809413));
#173252=CARTESIAN_POINT('Ctrl Pts',(62.3350625756721,-5.08571015610324,
49.3606639102153));
#173253=CARTESIAN_POINT('Ctrl Pts',(62.4388006637816,-5.26301523477087,
49.345903663078));
#173254=CARTESIAN_POINT('Ctrl Pts',(62.4686149550707,-5.312998716639,49.3416422986169));
#173255=CARTESIAN_POINT('Ctrl Pts',(62.5072139561134,-5.37648344525029,
49.3361022797283));
#173256=CARTESIAN_POINT('Ctrl Pts',(62.51561262016,-5.39022439117882,49.3348954770061));
#173257=CARTESIAN_POINT('Ctrl Pts',(62.691009452068,-5.67568523459674,49.3096649194389));
#173258=CARTESIAN_POINT('Ctrl Pts',(62.8703876086604,-5.93938633574773,
49.2833333046337));
#173259=CARTESIAN_POINT('Ctrl Pts',(63.2498229223662,-6.44493318261301,
49.2270615686531));
#173260=CARTESIAN_POINT('Ctrl Pts',(63.4493038913084,-6.68678916115698,
49.1972166504444));
#173261=CARTESIAN_POINT('Ctrl Pts',(63.7244571744634,-6.99077316725946,
49.1560595277977));
#173262=CARTESIAN_POINT('Ctrl Pts',(63.7904476578538,-7.06162529942621,
49.1461897604786));
#173263=CARTESIAN_POINT('Ctrl Pts',(63.8975013770108,-7.17333252315719,
49.1301934309612));
#173264=CARTESIAN_POINT('Ctrl Pts',(63.9379276847023,-7.21480264918602,
49.1241561256065));
#173265=CARTESIAN_POINT('Ctrl Pts',(64.0142732844073,-7.29179467432231,
49.1127641635071));
#173266=CARTESIAN_POINT('Ctrl Pts',(64.0501081576586,-7.32739909170935,
49.1074207417009));
#173267=CARTESIAN_POINT('Ctrl Pts',(64.1302141795215,-7.4058142832196,49.0954817591005));
#173268=CARTESIAN_POINT('Ctrl Pts',(64.1746105550878,-7.44849170397798,
49.0888687980882));
#173269=CARTESIAN_POINT('Ctrl Pts',(64.3554553547475,-7.61920543577403,
49.0619394356935));
#173270=CARTESIAN_POINT('Ctrl Pts',(64.4949922116416,-7.74383224910817,
49.0411787461335));
#173271=CARTESIAN_POINT('Ctrl Pts',(64.637845022461,-7.86451166255217,49.0198937666656));
#173272=CARTESIAN_POINT('',(61.9506556875214,-4.30478031493663,49.4937177486874));
#173273=CARTESIAN_POINT('Origin',(71.1115577432812,0.,47.8784035486295));
#173274=CARTESIAN_POINT('Ctrl Pts',(61.9506598557337,-4.30478938863868,
49.4937172065276));
#173275=CARTESIAN_POINT('Ctrl Pts',(61.9294009716217,-4.25851127052955,
49.4964823507224));
#173276=CARTESIAN_POINT('Ctrl Pts',(61.9084833788973,-4.21207392643947,
49.4991933391632));
#173277=CARTESIAN_POINT('Ctrl Pts',(61.8674561497903,-4.11916380707771,
49.5044907771788));
#173278=CARTESIAN_POINT('Ctrl Pts',(61.8473429944743,-4.07269417580616,
49.5070778015142));
#173279=CARTESIAN_POINT('Ctrl Pts',(61.7914021009595,-3.94079672650919,
49.5142441877163));
#173280=CARTESIAN_POINT('Ctrl Pts',(61.7563777950916,-3.85502670269385,
49.5186962557556));
#173281=CARTESIAN_POINT('Ctrl Pts',(61.667277166826,-3.62816619246239,49.5299253978876));
#173282=CARTESIAN_POINT('Ctrl Pts',(61.615126883088,-3.48632894604623,49.5363968482329));
#173283=CARTESIAN_POINT('Ctrl Pts',(61.3816664441308,-2.80571450758912,
49.564824352624));
#173284=CARTESIAN_POINT('Ctrl Pts',(61.2417600627997,-2.25353444009203,
49.5802036917875));
#173285=CARTESIAN_POINT('Ctrl Pts',(61.0762492875393,-1.26672398661516,
49.5929998798764));
#173286=CARTESIAN_POINT('Ctrl Pts',(61.0313922556877,-0.836811029042843,
49.5938184905104));
#173287=CARTESIAN_POINT('Ctrl Pts',(61.0096444362259,-0.319519193756273,
49.5883932902413));
#173288=CARTESIAN_POINT('Ctrl Pts',(61.0070935436993,-0.233603440773108,
49.5872805795056));
#173289=CARTESIAN_POINT('Ctrl Pts',(61.004747258745,-0.0984492968550968,
49.5851883899502));
#173290=CARTESIAN_POINT('Ctrl Pts',(61.0042402605943,-0.0492249582819704,
49.5843551161851));
#173291=CARTESIAN_POINT('Ctrl Pts',(61.0040805671216,3.48409058108532E-11,
49.583449449497));
#173292=CARTESIAN_POINT('Origin',(71.2118135654015,4.33680868994202E-16,
48.4469825699312));
#173293=CARTESIAN_POINT('',(62.4496382053723,-6.991174202171E-16,52.0228437193745));
#173294=CARTESIAN_POINT('Origin',(71.5591099207353,4.33680868994202E-16,
50.4165980759556));
#173295=CARTESIAN_POINT('',(62.1023418500385,-6.991174202171E-16,50.0532282133501));
#173296=CARTESIAN_POINT('',(62.1023418500385,-6.991174202171E-16,50.0532282133501));
#173297=CARTESIAN_POINT('',(80.3212852807645,1.19403062916867E-15,46.8407369265124));
#173298=CARTESIAN_POINT('Origin',(71.2118135654015,4.33680868994202E-16,
48.4469825699312));
#173299=CARTESIAN_POINT('Origin',(71.2118135654015,4.33680868994202E-16,
48.4469825699312));
#173300=CARTESIAN_POINT('Origin',(71.5591099207353,0.,50.4165980759556));
#173301=CARTESIAN_POINT('',(61.0735209929348,-1.34711147906209E-15,54.2963435363159));
#173302=CARTESIAN_POINT('Origin',(71.9064062760691,0.,52.38621358198));
#173303=CARTESIAN_POINT('',(60.726224637601,-1.34711147906209E-15,52.3267280302915));
#173304=CARTESIAN_POINT('',(60.726224637601,-1.34711147906209E-15,52.3267280302915));
#173305=CARTESIAN_POINT('Origin',(71.5591099207353,0.,50.4165980759556));
#173306=CARTESIAN_POINT('Origin',(71.9064062760691,0.,52.38621358198));
#173307=CARTESIAN_POINT('',(63.2427116913412,-1.12055182121983E-15,55.9447099136567));
#173308=CARTESIAN_POINT('Origin',(72.2537026314029,0.,54.3558290880045));
#173309=CARTESIAN_POINT('',(62.8954153360073,-1.12055182121983E-15,53.9750944076322));
#173310=CARTESIAN_POINT('',(62.8954153360073,-1.12055182121983E-15,53.9750944076322));
#173311=CARTESIAN_POINT('Origin',(71.9064062760691,0.,52.38621358198));
#173312=CARTESIAN_POINT('Origin',(72.2537026314029,-4.33680868994202E-16,
54.3558290880045));
#173313=CARTESIAN_POINT('',(72.8461248809557,9.99946181761383,58.3130755089793));
#173314=CARTESIAN_POINT('Ctrl Pts',(63.0153743226244,-3.90012641998867E-11,
59.5503705382064));
#173315=CARTESIAN_POINT('Ctrl Pts',(63.0153972406607,-0.0127238816044014,
59.5505005128487));
#173316=CARTESIAN_POINT('Ctrl Pts',(63.015444218918,-0.025447716762289,
59.5506270909235));
#173317=CARTESIAN_POINT('Ctrl Pts',(63.015670373446,-0.0659565906910079,
59.5510192008863));
#173318=CARTESIAN_POINT('Ctrl Pts',(63.0159402079255,-0.0937410855028063,
59.5512718523828));
#173319=CARTESIAN_POINT('Ctrl Pts',(63.017126433562,-0.179454306078677,
59.5520003585878));
#173320=CARTESIAN_POINT('Ctrl Pts',(63.0184266650033,-0.237376994939163,
59.5524209190357));
#173321=CARTESIAN_POINT('Ctrl Pts',(63.0311791315022,-0.648040738871901,
59.554880622942));
#173322=CARTESIAN_POINT('Ctrl Pts',(63.060603601808,-0.999995108331238,
59.5542488690691));
#173323=CARTESIAN_POINT('Ctrl Pts',(63.1914958773353,-1.9594219188347,59.543981049886));
#173324=CARTESIAN_POINT('Ctrl Pts',(63.3299820083306,-2.56022648173973,
59.5279430870644));
#173325=CARTESIAN_POINT('Ctrl Pts',(63.577938413814,-3.31532630551769,59.4937772209545));
#173326=CARTESIAN_POINT('Ctrl Pts',(63.6385814296694,-3.48467194886097,
59.4851690595328));
#173327=CARTESIAN_POINT('Ctrl Pts',(63.7276922896354,-3.71409752939761,
59.4721915985195));
#173328=CARTESIAN_POINT('Ctrl Pts',(63.7523091857069,-3.77567839889446,
59.4685762666482));
#173329=CARTESIAN_POINT('Ctrl Pts',(63.7943152147813,-3.87783776628032,
59.4623578939484));
#173330=CARTESIAN_POINT('Ctrl Pts',(63.8113696545304,-3.91855553505762,
59.4598204580738));
#173331=CARTESIAN_POINT('Ctrl Pts',(63.8455275209278,-3.99863449379825,
59.4547135931825));
#173332=CARTESIAN_POINT('Ctrl Pts',(63.8626161277331,-4.03800115895169,
59.4521470542971));
#173333=CARTESIAN_POINT('Ctrl Pts',(63.9042491226319,-4.13226440080662,
59.445866798204));
#173334=CARTESIAN_POINT('Ctrl Pts',(63.9290322945844,-4.18705052954745,
59.442106218525));
#173335=CARTESIAN_POINT('Ctrl Pts',(64.0178223892747,-4.37876096587211,
59.428558368047));
#173336=CARTESIAN_POINT('Ctrl Pts',(64.0843950554685,-4.51443814573505,
59.4182680211522));
#173337=CARTESIAN_POINT('Ctrl Pts',(64.2577840528361,-4.84862924827669,
59.3911736943488));
#173338=CARTESIAN_POINT('Ctrl Pts',(64.3682301684812,-5.04510610853753,
59.3736634282429));
#173339=CARTESIAN_POINT('Ctrl Pts',(64.7157075033443,-5.61738396006518,
59.3180188526635));
#173340=CARTESIAN_POINT('Ctrl Pts',(64.9709856154607,-5.98109874914044,
59.2764334550044));
#173341=CARTESIAN_POINT('Ctrl Pts',(65.4055645901478,-6.52006368772027,
59.2056383501741));
#173342=CARTESIAN_POINT('Ctrl Pts',(65.5688871659162,-6.70777928239044,
59.1790381863562));
#173343=CARTESIAN_POINT('Ctrl Pts',(65.7724134155743,-6.92469182104557,
59.1460772755362));
#173344=CARTESIAN_POINT('Ctrl Pts',(65.8060762427447,-6.96004241693961,
59.140631466992));
#173345=CARTESIAN_POINT('Ctrl Pts',(65.8590087100124,-7.01481347859254,
59.1320793091153));
#173346=CARTESIAN_POINT('Ctrl Pts',(65.8781019561053,-7.03440701784639,
59.1289966624021));
#173347=CARTESIAN_POINT('Ctrl Pts',(65.9120948662297,-7.06900296197743,
59.1235127045085));
#173348=CARTESIAN_POINT('Ctrl Pts',(65.9269621141047,-7.08403741921878,
59.1211156858566));
#173349=CARTESIAN_POINT('Ctrl Pts',(65.9628921482931,-7.12013975848987,
59.1153261899299));
#173350=CARTESIAN_POINT('Ctrl Pts',(65.9840014881413,-7.14115991619729,
59.1119275771374));
#173351=CARTESIAN_POINT('Ctrl Pts',(66.0494881321774,-7.20578455083538,
59.1013919552325));
#173352=CARTESIAN_POINT('Ctrl Pts',(66.0941781085156,-7.24906319306956,
59.0942130436402));
#173353=CARTESIAN_POINT('Ctrl Pts',(66.3225891886383,-7.4661314114206,59.0575643349633));
#173354=CARTESIAN_POINT('Ctrl Pts',(66.5124360680845,-7.63319524967299,
59.0272396712087));
#173355=CARTESIAN_POINT('Ctrl Pts',(67.1810548013945,-8.17764157613828,
58.9204019059097));
#173356=CARTESIAN_POINT('Ctrl Pts',(67.687749069195,-8.51764354585437,58.839288498054));
#173357=CARTESIAN_POINT('Ctrl Pts',(68.3717923878515,-8.89008177659352,
58.7280371590308));
#173358=CARTESIAN_POINT('Ctrl Pts',(68.523824359906,-8.96779965280919,58.703216448197));
#173359=CARTESIAN_POINT('Ctrl Pts',(68.7358647752087,-9.06931987054389,
58.6684580987205));
#173360=CARTESIAN_POINT('Ctrl Pts',(68.7942463895949,-9.09656908715674,
58.6588737037093));
#173361=CARTESIAN_POINT('Ctrl Pts',(68.8884982994032,-9.13943631771255,
58.6433774281439));
#173362=CARTESIAN_POINT('Ctrl Pts',(68.9242060720533,-9.1554198934331,58.6375013119101));
#173363=CARTESIAN_POINT('Ctrl Pts',(68.9985283346228,-9.18815626502272,
58.6252598037237));
#173364=CARTESIAN_POINT('Ctrl Pts',(69.0371565514239,-9.20487475187628,
58.6188913202396));
#173365=CARTESIAN_POINT('Ctrl Pts',(69.1285119656597,-9.24371779764268,
58.6038156489328));
#173366=CARTESIAN_POINT('Ctrl Pts',(69.1813247014005,-9.26562972817009,
58.5950892397882));
#173367=CARTESIAN_POINT('Ctrl Pts',(69.3586907108283,-9.33740673626942,
58.5657459079227));
#173368=CARTESIAN_POINT('Ctrl Pts',(69.4840492563005,-9.38516584059354,
58.5449464070969));
#173369=CARTESIAN_POINT('Ctrl Pts',(69.7880668066933,-9.49389191081518,
58.4943704100662));
#173370=CARTESIAN_POINT('Ctrl Pts',(69.9675568819216,-9.55228305330136,
58.4644011635447));
#173371=CARTESIAN_POINT('Ctrl Pts',(70.7867530700148,-9.79278136731914,
58.3272347957418));
#173372=CARTESIAN_POINT('Ctrl Pts',(71.4417459459794,-9.91427382230702,
58.2163822146416));
#173373=CARTESIAN_POINT('Ctrl Pts',(72.2909494508674,-9.98325294556837,
58.073953998191));
#173374=CARTESIAN_POINT('Ctrl Pts',(72.4783440086267,-9.99302939405581,
58.0426137861576));
#173375=CARTESIAN_POINT('Ctrl Pts',(72.7092993085787,-9.99838801357882,
58.0041839749464));
#173376=CARTESIAN_POINT('Ctrl Pts',(72.7526810991047,-9.99910430876741,
57.9969739744684));
#173377=CARTESIAN_POINT('Ctrl Pts',(72.8208982492309,-9.99977439078064,
57.985651176986));
#173378=CARTESIAN_POINT('Ctrl Pts',(72.8457301582975,-9.99992326850401,
57.9815326198913));
#173379=CARTESIAN_POINT('Ctrl Pts',(72.8899657043635,-10.0000191893599,
57.974201626971));
#173380=CARTESIAN_POINT('Ctrl Pts',(72.9093687778549,-10.0000032472533,
57.9709880394958));
#173381=CARTESIAN_POINT('Ctrl Pts',(72.9560850226036,-9.99982518655341,
57.9632555469892));
#173382=CARTESIAN_POINT('Ctrl Pts',(72.9833980664459,-9.99960612928655,
57.95873858226));
#173383=CARTESIAN_POINT('Ctrl Pts',(73.0673484280767,-9.99857949922355,
57.9448664145709));
#173384=CARTESIAN_POINT('Ctrl Pts',(73.1239820394017,-9.99739259086614,
57.9355239956593));
#173385=CARTESIAN_POINT('Ctrl Pts',(73.6369106535519,-9.98216442695471,
57.8510368702289));
#173386=CARTESIAN_POINT('Ctrl Pts',(74.0918896743786,-9.93654433063337,
57.776979615097));
#173387=CARTESIAN_POINT('Ctrl Pts',(75.1339980204783,-9.75747861245336,
57.6075192203945));
#173388=CARTESIAN_POINT('Ctrl Pts',(75.7155099326642,-9.60128775932434,
57.5130253832674));
#173389=CARTESIAN_POINT('Ctrl Pts',(76.3817355004841,-9.35460524953656,
57.4038240322294));
#173390=CARTESIAN_POINT('Ctrl Pts',(76.4835659284401,-9.31494784018957,
57.3871091765992));
#173391=CARTESIAN_POINT('Ctrl Pts',(76.6335636359693,-9.25361818247504,
57.3624515261964));
#173392=CARTESIAN_POINT('Ctrl Pts',(76.6822450676087,-9.23325265268029,
57.3544431961951));
#173393=CARTESIAN_POINT('Ctrl Pts',(76.7688873856061,-9.1961802856855,57.3401799165044));
#173394=CARTESIAN_POINT('Ctrl Pts',(76.8069101801534,-9.17962452221205,
57.3339169693134));
#173395=CARTESIAN_POINT('Ctrl Pts',(76.8872849321029,-9.14401880221152,
57.3206705985712));
#173396=CARTESIAN_POINT('Ctrl Pts',(76.9296093820722,-9.12490792130417,
57.3136908201104));
#173397=CARTESIAN_POINT('Ctrl Pts',(77.0429865065423,-9.07274046470455,
57.294982168038));
#173398=CARTESIAN_POINT('Ctrl Pts',(77.1137856280795,-9.03912897268019,
57.2832871923927));
#173399=CARTESIAN_POINT('Ctrl Pts',(77.5054901203791,-8.84737815138417,
57.2185199911168));
#173400=CARTESIAN_POINT('Ctrl Pts',(77.8181007715108,-8.67253810194579,
57.1665794757874));
#173401=CARTESIAN_POINT('Ctrl Pts',(78.4865875535025,-8.24917525748617,
57.0553471649651));
#173402=CARTESIAN_POINT('Ctrl Pts',(78.8370898372806,-7.99335053134205,
56.9969090578562));
#173403=CARTESIAN_POINT('Ctrl Pts',(79.3494357490841,-7.56514391086097,
56.9122457696215));
#173404=CARTESIAN_POINT('Ctrl Pts',(79.523584019982,-7.40881765385398,56.8836243759743));
#173405=CARTESIAN_POINT('Ctrl Pts',(79.7268934068559,-7.21294877118822,
56.8505570511511));
#173406=CARTESIAN_POINT('Ctrl Pts',(79.761381174521,-7.17923736371063,56.8449604366153));
#173407=CARTESIAN_POINT('Ctrl Pts',(79.8149575964137,-7.12610208360609,
56.8362879582245));
#173408=CARTESIAN_POINT('Ctrl Pts',(79.8342105098096,-7.10685082368393,
56.8331759397018));
#173409=CARTESIAN_POINT('Ctrl Pts',(79.8682893117592,-7.0724951025603,56.8276758506217));
#173410=CARTESIAN_POINT('Ctrl Pts',(79.8831457204213,-7.05742247501516,
56.825281011699));
#173411=CARTESIAN_POINT('Ctrl Pts',(79.9189277391044,-7.02088820525327,
56.8195198916435));
#173412=CARTESIAN_POINT('Ctrl Pts',(79.9398056652184,-6.99937859483033,
56.8161641379583));
#173413=CARTESIAN_POINT('Ctrl Pts',(80.0043851385759,-6.93224333926219,
56.8058011541814));
#173414=CARTESIAN_POINT('Ctrl Pts',(80.0477566006229,-6.88629127384611,
56.7988658139896));
#173415=CARTESIAN_POINT('Ctrl Pts',(80.2681868436911,-6.64826358789515,
56.7637317615667));
#173416=CARTESIAN_POINT('Ctrl Pts',(80.4382129438355,-6.44959649984763,
56.7370123858501));
#173417=CARTESIAN_POINT('Ctrl Pts',(81.0118714857229,-5.72354607914022,
56.6477165955925));
#173418=CARTESIAN_POINT('Ctrl Pts',(81.3711484916976,-5.16233930121776,
56.593297712963));
#173419=CARTESIAN_POINT('Ctrl Pts',(81.7301171758017,-4.45584920586747,
56.5392293896068));
#173420=CARTESIAN_POINT('Ctrl Pts',(81.7855469201543,-4.34143560350729,
56.5308967250654));
#173421=CARTESIAN_POINT('Ctrl Pts',(81.8606013483149,-4.17872253269041,
56.5196337823115));
#173422=CARTESIAN_POINT('Ctrl Pts',(81.8820352272707,-4.13129108731475,
56.5164198239708));
#173423=CARTESIAN_POINT('Ctrl Pts',(81.9188526854303,-4.04810309294576,
56.5109034407096));
#173424=CARTESIAN_POINT('Ctrl Pts',(81.9343980121356,-4.01242106548909,
56.5085756772287));
#173425=CARTESIAN_POINT('Ctrl Pts',(81.9666698308304,-3.93715668223187,
56.5037462684997));
#173426=CARTESIAN_POINT('Ctrl Pts',(81.983350805942,-3.89755521620216,56.5012517488476));
#173427=CARTESIAN_POINT('Ctrl Pts',(82.0228732947852,-3.80202205813339,
56.4953457956932));
#173428=CARTESIAN_POINT('Ctrl Pts',(82.0454668398663,-3.74598724189699,
56.4919732041538));
#173429=CARTESIAN_POINT('Ctrl Pts',(82.1232852072188,-3.54786746878617,
56.4803707974395));
#173430=CARTESIAN_POINT('Ctrl Pts',(82.1757966107307,-3.40471499598959,
56.4725665516287));
#173431=CARTESIAN_POINT('Ctrl Pts',(82.2974089349353,-3.04839754066916,
56.4545746395008));
#173432=CARTESIAN_POINT('Ctrl Pts',(82.362702218747,-2.83399194437994,56.4449903211823));
#173433=CARTESIAN_POINT('Ctrl Pts',(82.5133755507188,-2.27292092536084,
56.4231974807356));
#173434=CARTESIAN_POINT('Ctrl Pts',(82.5876402737568,-1.92353356160316,
56.4128057182158));
#173435=CARTESIAN_POINT('Ctrl Pts',(82.6717518192979,-1.39111488943614,
56.4021240616837));
#173436=CARTESIAN_POINT('Ctrl Pts',(82.6953154067304,-1.21059315410368,
56.3993835526276));
#173437=CARTESIAN_POINT('Ctrl Pts',(82.7408522150387,-0.769879807381216,
56.3949493823501));
#173438=CARTESIAN_POINT('Ctrl Pts',(82.7576795567097,-0.50928211026459,
56.3942270198793));
#173439=CARTESIAN_POINT('Ctrl Pts',(82.7656342431276,-0.204847392485989,
56.3957898248367));
#173440=CARTESIAN_POINT('Ctrl Pts',(82.7664924732408,-0.161355025493206,
56.3960703577545));
#173441=CARTESIAN_POINT('Ctrl Pts',(82.7674377811045,-0.0905000121902342,
56.3966220412924));
#173442=CARTESIAN_POINT('Ctrl Pts',(82.767692825144,-0.0631399135396372,
56.3968580573713));
#173443=CARTESIAN_POINT('Ctrl Pts',(82.7679532228835,-0.0140427354381262,
56.3973232171349));
#173444=CARTESIAN_POINT('Ctrl Pts',(82.7679991279918,0.00769383312288637,
56.3975438216474));
#173445=CARTESIAN_POINT('Ctrl Pts',(82.7679472374795,0.0557499153964174,
56.3980640098788));
#173446=CARTESIAN_POINT('Ctrl Pts',(82.7678170962327,0.0820689182735145,
56.3983703916125));
#173447=CARTESIAN_POINT('Ctrl Pts',(82.7671393580162,0.158987447891594,
56.3993280919463));
#173448=CARTESIAN_POINT('Ctrl Pts',(82.7663173891197,0.209583024122863,
56.4000368302565));
#173449=CARTESIAN_POINT('Ctrl Pts',(82.7542402509525,0.719447650404466,
56.4079605514154));
#173450=CARTESIAN_POINT('Ctrl Pts',(82.7123557420851,1.17735529161294,56.4214469228521));
#173451=CARTESIAN_POINT('Ctrl Pts',(82.540832122938,2.24635608924051,56.4661470751882));
#173452=CARTESIAN_POINT('Ctrl Pts',(82.3854851470434,2.85121668799052,56.501820406516));
#173453=CARTESIAN_POINT('Ctrl Pts',(82.1386395300699,3.54000434630717,56.553781145612));
#173454=CARTESIAN_POINT('Ctrl Pts',(82.1001676646831,3.64209240272902,56.5617916307335));
#173455=CARTESIAN_POINT('Ctrl Pts',(82.0405538098305,3.79280040737901,56.5740785028626));
#173456=CARTESIAN_POINT('Ctrl Pts',(82.0206709476821,3.84192555607953,56.5781573750507));
#173457=CARTESIAN_POINT('Ctrl Pts',(81.9844173075688,3.92949900162393,56.5855611586151));
#173458=CARTESIAN_POINT('Ctrl Pts',(81.9681928481918,3.968008425401,56.5888631306304));
#173459=CARTESIAN_POINT('Ctrl Pts',(81.9332342088384,4.04955745250443,56.5959540893212));
#173460=CARTESIAN_POINT('Ctrl Pts',(81.9144378849117,4.09256846232226,56.5997527901644));
#173461=CARTESIAN_POINT('Ctrl Pts',(81.8629634791182,4.20813908897189,56.6101190986596));
#173462=CARTESIAN_POINT('Ctrl Pts',(81.829725698529,4.28043771285296,56.6167743630153));
#173463=CARTESIAN_POINT('Ctrl Pts',(81.635620859875,4.68974778331293,56.6554326229452));
#173464=CARTESIAN_POINT('Ctrl Pts',(81.456987925288,5.01773594004858,56.6902110873017));
#173465=CARTESIAN_POINT('Ctrl Pts',(81.0153001055961,5.73075077929968,56.7750684403635));
#173466=CARTESIAN_POINT('Ctrl Pts',(80.7428502346743,6.10872866637621,56.8266866698138));
#173467=CARTESIAN_POINT('Ctrl Pts',(80.3215825979059,6.61457358668624,56.9066799010964));
#173468=CARTESIAN_POINT('Ctrl Pts',(80.1935151813372,6.75954443633545,56.9310229636541));
#173469=CARTESIAN_POINT('Ctrl Pts',(80.0297244066458,6.93441398475723,56.9622766104188));
#173470=CARTESIAN_POINT('Ctrl Pts',(79.9978327158827,6.967989670514,56.9683674412743));
#173471=CARTESIAN_POINT('Ctrl Pts',(79.9473384010373,7.02041215847785,56.9780212550551));
#173472=CARTESIAN_POINT('Ctrl Pts',(79.9288898550424,7.03941263564539,56.9815504623455));
#173473=CARTESIAN_POINT('Ctrl Pts',(79.8938406783404,7.07522297942018,56.9882597139624));
#173474=CARTESIAN_POINT('Ctrl Pts',(79.8772554062885,7.09204801206173,56.9914363915921));
#173475=CARTESIAN_POINT('Ctrl Pts',(79.8377102518846,7.13187970416904,56.9990149017995));
#173476=CARTESIAN_POINT('Ctrl Pts',(79.8146982451438,7.1548320385734,57.0034282669222));
#173477=CARTESIAN_POINT('Ctrl Pts',(79.7362675129167,7.23229489000526,57.0184800924012));
#173478=CARTESIAN_POINT('Ctrl Pts',(79.6803322742601,7.28625638218252,57.0292314663774));
#173479=CARTESIAN_POINT('Ctrl Pts',(79.5410759231692,7.41747193530605,57.0560274184527));
#173480=CARTESIAN_POINT('Ctrl Pts',(79.4570638547685,7.49394657412402,57.0722183209985));
#173481=CARTESIAN_POINT('Ctrl Pts',(79.0872997516207,7.81906044935153,57.1435280569425));
#173482=CARTESIAN_POINT('Ctrl Pts',(78.7889709618237,8.05235200373957,57.2011712390321));
#173483=CARTESIAN_POINT('Ctrl Pts',(78.1174129528399,8.517604868232,57.3302768838052));
#173484=CARTESIAN_POINT('Ctrl Pts',(77.7405971542483,8.74279654721798,57.4023171101932));
#173485=CARTESIAN_POINT('Ctrl Pts',(77.2559807990117,8.98974113405135,57.4940844809444));
#173486=CARTESIAN_POINT('Ctrl Pts',(77.1610063170831,9.03620483700701,57.512030631217));
#173487=CARTESIAN_POINT('Ctrl Pts',(77.0182703926689,9.10317545515927,57.5389429559715));
#173488=CARTESIAN_POINT('Ctrl Pts',(76.9710594998861,9.1248668231769,57.5478349740397));
#173489=CARTESIAN_POINT('Ctrl Pts',(76.8860420719781,9.16310689984286,57.5638308016666));
#173490=CARTESIAN_POINT('Ctrl Pts',(76.8482983669322,9.17979569101789,57.5709262592174));
#173491=CARTESIAN_POINT('Ctrl Pts',(76.7676386295085,9.2148482130727,57.5860769369247));
#173492=CARTESIAN_POINT('Ctrl Pts',(76.7246948348139,9.23314390965153,57.5941357238436));
#173493=CARTESIAN_POINT('Ctrl Pts',(76.60789671928,9.28191352929628,57.6160337185872));
#173494=CARTESIAN_POINT('Ctrl Pts',(76.5338007459809,9.31178522144678,57.6299038641073));
#173495=CARTESIAN_POINT('Ctrl Pts',(76.1076484158523,9.47750842145583,57.7095554523373));
#173496=CARTESIAN_POINT('Ctrl Pts',(75.7484278885031,9.59361138243197,57.7762128644523));
#173497=CARTESIAN_POINT('Ctrl Pts',(74.8034124781921,9.83925991498714,57.9508388607145));
#173498=CARTESIAN_POINT('Ctrl Pts',(74.2108875082253,9.93585627851298,58.0595775716456));
#173499=CARTESIAN_POINT('Ctrl Pts',(73.5345862939291,9.9825167094355,58.1848171674148));
#173500=CARTESIAN_POINT('Ctrl Pts',(73.4555248144918,9.98699671540131,58.1994767589549));
#173501=CARTESIAN_POINT('Ctrl Pts',(73.288548965615,9.99440248209955,58.2304880626753));
#173502=CARTESIAN_POINT('Ctrl Pts',(73.2006327068963,9.99710044370478,58.2468457342875));
#173503=CARTESIAN_POINT('Ctrl Pts',(73.0799243445904,9.99915650863733,58.2693555841932));
#173504=CARTESIAN_POINT('Ctrl Pts',(73.0471476756212,9.99954803125916,58.2754729715675));
#173505=CARTESIAN_POINT('Ctrl Pts',(72.9923354438664,9.99992389894518,58.2857123252784));
#173506=CARTESIAN_POINT('Ctrl Pts',(72.970300205909,9.99999963373074,58.2898311889631));
#173507=CARTESIAN_POINT('Ctrl Pts',(72.9316375680396,10.0000002740669,58.2970626910476));
#173508=CARTESIAN_POINT('Ctrl Pts',(72.9150100544956,9.99995763056317,58.3001742181077));
#173509=CARTESIAN_POINT('Ctrl Pts',(72.8809597342367,9.99978240993586,58.3065490651667));
#173510=CARTESIAN_POINT('Ctrl Pts',(72.8635468579032,9.99964571039881,58.3098106669871));
#173511=CARTESIAN_POINT('Ctrl Pts',(72.8461248809557,9.99946181761384,58.3130755089793));
#173512=CARTESIAN_POINT('',(75.0041293598347,9.77968000307984,57.9325610948633));
#173513=CARTESIAN_POINT('Origin',(72.9482953420705,-4.33680868994202E-16,
58.2950601000533));
#173514=CARTESIAN_POINT('Ctrl Pts',(75.0041293598347,9.77968000307985,57.9325610948633));
#173515=CARTESIAN_POINT('Ctrl Pts',(75.4467731959013,9.68351044596169,57.8484084812634));
#173516=CARTESIAN_POINT('Ctrl Pts',(75.8823845795871,9.55632191769558,57.7657085087382));
#173517=CARTESIAN_POINT('Ctrl Pts',(76.4137973744841,9.35987501664702,57.6653655792823));
#173518=CARTESIAN_POINT('Ctrl Pts',(76.5190230165497,9.31888043583612,57.6455221604581));
#173519=CARTESIAN_POINT('Ctrl Pts',(76.6728943200235,9.25582894320786,57.6165442198741));
#173520=CARTESIAN_POINT('Ctrl Pts',(76.7220899015498,9.23519660415285,57.6072853543921));
#173521=CARTESIAN_POINT('Ctrl Pts',(76.8091783031061,9.19782827926034,57.5909053484051));
#173522=CARTESIAN_POINT('Ctrl Pts',(76.8471362271565,9.18125383967444,57.5837696068368));
#173523=CARTESIAN_POINT('Ctrl Pts',(76.9268996140984,9.14581800647895,57.5687822374121));
#173524=CARTESIAN_POINT('Ctrl Pts',(76.9686808112055,9.12690222134181,57.5609359660551));
#173525=CARTESIAN_POINT('Ctrl Pts',(77.0794756270088,9.07579704194072,57.5401405485904));
#173526=CARTESIAN_POINT('Ctrl Pts',(77.1482563307976,9.04308963391436,57.5272425661963));
#173527=CARTESIAN_POINT('Ctrl Pts',(77.4705124676917,8.88519716572557,57.4668634272212));
#173528=CARTESIAN_POINT('Ctrl Pts',(77.7190181804325,8.74977280691174,57.4204584101275));
#173529=CARTESIAN_POINT('Ctrl Pts',(78.030189700602,8.56227075632774,57.3624489883775));
#173530=CARTESIAN_POINT('Ctrl Pts',(78.0984063294809,8.52001558487187,57.3497377317351));
#173531=CARTESIAN_POINT('Ctrl Pts',(78.5379996776848,8.24019661230819,57.2678455490562));
#173532=CARTESIAN_POINT('Ctrl Pts',(78.8939109332315,7.97842237061735,57.2016625143765));
#173533=CARTESIAN_POINT('Ctrl Pts',(79.3476775541994,7.5950744599062,57.1165645447774));
#173534=CARTESIAN_POINT('Ctrl Pts',(79.4617500686661,7.49408041115362,57.0951020493699));
#173535=CARTESIAN_POINT('Ctrl Pts',(79.6434067570898,7.32557470952058,57.0607515561276));
#173536=CARTESIAN_POINT('Ctrl Pts',(79.7124128243414,7.25967526053967,57.0476603624098));
#173537=CARTESIAN_POINT('Ctrl Pts',(79.8058152013125,7.1678479967598,57.0298693125774));
#173538=CARTESIAN_POINT('Ctrl Pts',(79.831033463482,7.14278536173196,57.0250584543731));
#173539=CARTESIAN_POINT('Ctrl Pts',(79.8731595354281,7.10046388306709,57.0170088902476));
#173540=CARTESIAN_POINT('Ctrl Pts',(79.8901396147404,7.08327920502248,57.0137606339998));
#173541=CARTESIAN_POINT('Ctrl Pts',(79.9247720949334,7.04797082913142,57.0071276940998));
#173542=CARTESIAN_POINT('Ctrl Pts',(79.9424182806319,7.02984123948933,57.0037438572943));
#173543=CARTESIAN_POINT('Ctrl Pts',(79.9884130416565,6.98222137726603,56.9949133561584));
#173544=CARTESIAN_POINT('Ctrl Pts',(80.0166497030171,6.9526209096185,56.9894816561048));
#173545=CARTESIAN_POINT('Ctrl Pts',(80.1346281038101,6.82739516097374,56.9667451047949));
#173546=CARTESIAN_POINT('Ctrl Pts',(80.2226658552105,6.73013999979803,56.9496759291628));
#173547=CARTESIAN_POINT('Ctrl Pts',(80.6517489159532,6.23676348029673,56.8660676926006));
#173548=CARTESIAN_POINT('Ctrl Pts',(80.9633740470488,5.81539628222818,56.8040398013639));
#173549=CARTESIAN_POINT('Ctrl Pts',(81.4453105520073,5.04364709862668,56.7073943844033));
#173550=CARTESIAN_POINT('Ctrl Pts',(81.6308100979954,4.70447436208174,56.6699331639591));
#173551=CARTESIAN_POINT('Ctrl Pts',(81.8308315451034,4.28277923689722,56.6294054265953));
#173552=CARTESIAN_POINT('Ctrl Pts',(81.8643070574446,4.20997536880926,56.6226166543153));
#173553=CARTESIAN_POINT('Ctrl Pts',(81.9160634039712,4.09378520405455,56.6121113516085));
#173554=CARTESIAN_POINT('Ctrl Pts',(81.9349106545668,4.05066516732619,56.6082837483891));
#173555=CARTESIAN_POINT('Ctrl Pts',(81.9699159626637,3.96902650888971,56.6011707618622));
#173556=CARTESIAN_POINT('Ctrl Pts',(81.9861375089232,3.93053730728745,56.5978729252474));
#173557=CARTESIAN_POINT('Ctrl Pts',(82.0223224139472,3.84317003762379,56.5905126847755));
#173558=CARTESIAN_POINT('Ctrl Pts',(82.0421431112546,3.79423190014176,56.5864782685232));
#173559=CARTESIAN_POINT('Ctrl Pts',(82.1013519343705,3.64468451638565,56.5744176790237));
#173560=CARTESIAN_POINT('Ctrl Pts',(82.1395177407302,3.54358074476346,56.5666310876267));
#173561=CARTESIAN_POINT('Ctrl Pts',(82.4352121519685,2.72058092398231,56.5061836780537));
#173562=CARTESIAN_POINT('Ctrl Pts',(82.6119385957249,1.97126808711763,56.4695337509488));
#173563=CARTESIAN_POINT('Ctrl Pts',(82.7281380081178,0.991098423549219,
56.441227783338));
#173564=CARTESIAN_POINT('Ctrl Pts',(82.7468707753557,0.772672857103674,
56.4361240812196));
#173565=CARTESIAN_POINT('Ctrl Pts',(82.7649817165545,0.43152827789089,56.4298729603844));
#173566=CARTESIAN_POINT('Ctrl Pts',(82.7692517277016,0.309152529424284,
56.4279738879533));
#173567=CARTESIAN_POINT('Ctrl Pts',(82.7719144434371,0.149660739939274,
56.4259216450456));
#173568=CARTESIAN_POINT('Ctrl Pts',(82.772329179715,0.112592879492385,56.4254744054767));
#173569=CARTESIAN_POINT('Ctrl Pts',(82.772672621413,0.0521326317942333,
56.4247925418771));
#173570=CARTESIAN_POINT('Ctrl Pts',(82.7727242018314,0.0287415005287805,
56.4245403622984));
#173571=CARTESIAN_POINT('Ctrl Pts',(82.7726661340173,-0.0169416276703035,
56.4240702888416));
#173572=CARTESIAN_POINT('Ctrl Pts',(82.7725639466525,-0.0392334248043524,
56.4238513272883));
#173573=CARTESIAN_POINT('Ctrl Pts',(82.7721695074228,-0.0891861820863875,
56.4233842456027));
#173574=CARTESIAN_POINT('Ctrl Pts',(82.7718373999325,-0.116846746766408,
56.4231418120011));
#173575=CARTESIAN_POINT('Ctrl Pts',(82.7702682912575,-0.214211127703349,
56.4223462242944));
#173576=CARTESIAN_POINT('Ctrl Pts',(82.7684232141908,-0.283903871205759,
56.4218809962315));
#173577=CARTESIAN_POINT('Ctrl Pts',(82.7514678215683,-0.744270613431884,
56.4195180785911));
#173578=CARTESIAN_POINT('Ctrl Pts',(82.7144252780961,-1.13382056373104,
56.4209119721584));
#173579=CARTESIAN_POINT('Ctrl Pts',(82.6052931881912,-1.8435017078387,56.4305945125638));
#173580=CARTESIAN_POINT('Ctrl Pts',(82.5399806426814,-2.16415622368731,
56.4377128133442));
#173581=CARTESIAN_POINT('Ctrl Pts',(82.3652512676739,-2.850712493114,56.4593591472192));
#173582=CARTESIAN_POINT('Ctrl Pts',(82.2504409526624,-3.21468349051168,
56.4749121566158));
#173583=CARTESIAN_POINT('Ctrl Pts',(82.0868436703953,-3.64682070573528,
56.4985531461655));
#173584=CARTESIAN_POINT('Ctrl Pts',(82.0572953560391,-3.72213598365673,
56.5028691375047));
#173585=CARTESIAN_POINT('Ctrl Pts',(82.0090577248409,-3.84088573544864,
56.5099858420662));
#173586=CARTESIAN_POINT('Ctrl Pts',(81.9909582898006,-3.88456282520516,
56.5126709482585));
#173587=CARTESIAN_POINT('Ctrl Pts',(81.9562808526226,-3.96661619706265,
56.5178428066775));
#173588=CARTESIAN_POINT('Ctrl Pts',(81.9397694297435,-4.00502032509871,
56.5203165159637));
#173589=CARTESIAN_POINT('Ctrl Pts',(81.9019320038613,-4.09154593844688,
56.5260099543371));
#173590=CARTESIAN_POINT('Ctrl Pts',(81.8804682009263,-4.13960401150748,
56.5292567362268));
#173591=CARTESIAN_POINT('Ctrl Pts',(81.8141787371259,-4.28497097243821,
56.5393345924802));
#173592=CARTESIAN_POINT('Ctrl Pts',(81.7681873359722,-4.38172372332873,
56.5463942828094));
#173593=CARTESIAN_POINT('Ctrl Pts',(81.5058189814662,-4.9117697516955,56.5870146276126));
#173594=CARTESIAN_POINT('Ctrl Pts',(81.2602263253606,-5.32942619913495,
56.6263204953934));
#173595=CARTESIAN_POINT('Ctrl Pts',(80.8728807565106,-5.89100418600472,
56.6891085646355));
#173596=CARTESIAN_POINT('Ctrl Pts',(80.7552135735168,-6.0511825699636,56.7082615762688));
#173597=CARTESIAN_POINT('Ctrl Pts',(80.4486136846681,-6.44346996401407,
56.7582033175902));
#173598=CARTESIAN_POINT('Ctrl Pts',(80.2539329007789,-6.67071082421701,
56.789947642877));
#173599=CARTESIAN_POINT('Ctrl Pts',(80.0155401018831,-6.92480966505708,
56.8285554582269));
#173600=CARTESIAN_POINT('Ctrl Pts',(79.981409274778,-6.96064813086315,56.8340769419965));
#173601=CARTESIAN_POINT('Ctrl Pts',(79.9281007141816,-7.01579153353887,
56.8426896371303));
#173602=CARTESIAN_POINT('Ctrl Pts',(79.9091073806543,-7.03527746600376,
56.8457560801649));
#173603=CARTESIAN_POINT('Ctrl Pts',(79.8735424461723,-7.07146550267104,
56.8514935310629));
#173604=CARTESIAN_POINT('Ctrl Pts',(79.8569910549472,-7.08818735527259,
56.854161837644));
#173605=CARTESIAN_POINT('Ctrl Pts',(79.8186029725964,-7.12669558203949,
56.8603464727588));
#173606=CARTESIAN_POINT('Ctrl Pts',(79.7967242794013,-7.14843877457842,
56.8638683496786));
#173607=CARTESIAN_POINT('Ctrl Pts',(79.7250615635052,-7.21899582591115,
56.8753954531214));
#173608=CARTESIAN_POINT('Ctrl Pts',(79.6748683310947,-7.26738210044562,
56.8834556529879));
#173609=CARTESIAN_POINT('Ctrl Pts',(79.3643522650139,-7.56046252068008,
56.9332577743923));
#173610=CARTESIAN_POINT('Ctrl Pts',(79.0916111501441,-7.79132120682228,
56.9767486482454));
#173611=CARTESIAN_POINT('Ctrl Pts',(78.5712273142436,-8.18558759206743,
57.0599872196992));
#173612=CARTESIAN_POINT('Ctrl Pts',(78.3274762239563,-8.35359141757045,
57.0990690184376));
#173613=CARTESIAN_POINT('Ctrl Pts',(77.7870864065363,-8.69130472030276,
57.1862307245456));
#173614=CARTESIAN_POINT('Ctrl Pts',(77.4884667747596,-8.85701839758791,
57.234711640782));
#173615=CARTESIAN_POINT('Ctrl Pts',(77.1124017501038,-9.04083342081322,
57.2962812532537));
#173616=CARTESIAN_POINT('Ctrl Pts',(77.0423483203296,-9.07405335039982,
57.307771059466));
#173617=CARTESIAN_POINT('Ctrl Pts',(76.929888902214,-9.12576107533153,57.3262494043446));
#173618=CARTESIAN_POINT('Ctrl Pts',(76.8877255700245,-9.14478760842171,
57.3331846997422));
#173619=CARTESIAN_POINT('Ctrl Pts',(76.8074789874316,-9.18031904352521,
57.3463981763294));
#173620=CARTESIAN_POINT('Ctrl Pts',(76.7694216413366,-9.19688205912606,
57.3526706594674));
#173621=CARTESIAN_POINT('Ctrl Pts',(76.6824509286958,-9.23407823800715,
57.3670183021908));
#173622=CARTESIAN_POINT('Ctrl Pts',(76.633474839612,-9.25455595583889,57.3751075500505));
#173623=CARTESIAN_POINT('Ctrl Pts',(76.4816189053081,-9.31660574127028,
57.4002184511718));
#173624=CARTESIAN_POINT('Ctrl Pts',(76.378214730224,-9.35682265566409,57.4173587225579));
#173625=CARTESIAN_POINT('Ctrl Pts',(75.739476932803,-9.59283472494313,57.5234747703491));
#173626=CARTESIAN_POINT('Ctrl Pts',(75.1891093755968,-9.74313201815768,
57.616012094509));
#173627=CARTESIAN_POINT('Ctrl Pts',(74.1900029408918,-9.92393171210476,
57.7842862093356));
#173628=CARTESIAN_POINT('Ctrl Pts',(73.7461400514239,-9.97308825592136,
57.8591144494693));
#173629=CARTESIAN_POINT('Ctrl Pts',(73.2170467071406,-9.99507402277027,
57.9474173561294));
#173630=CARTESIAN_POINT('Ctrl Pts',(73.13364670806,-9.99746554065069,57.9613093890031));
#173631=CARTESIAN_POINT('Ctrl Pts',(73.0183569662301,-9.99928798570218,
57.98046728672));
#173632=CARTESIAN_POINT('Ctrl Pts',(72.9864894719869,-9.99963516940403,
57.9857579020262));
#173633=CARTESIAN_POINT('Ctrl Pts',(72.9325316234741,-9.99995797073097,
57.9947070962686));
#173634=CARTESIAN_POINT('Ctrl Pts',(72.9104423816072,-10.0000149225272,
57.9983682015829));
#173635=CARTESIAN_POINT('Ctrl Pts',(72.8650142675287,-9.99997740846153,
58.0058921311289));
#173636=CARTESIAN_POINT('Ctrl Pts',(72.8416755847843,-9.99987420205068,
58.0097546436185));
#173637=CARTESIAN_POINT('Ctrl Pts',(72.7805815077889,-9.99938432564018,
58.0198583561287));
#173638=CARTESIAN_POINT('Ctrl Pts',(72.7428268299027,-9.9988619377727,58.0260949572416));
#173639=CARTESIAN_POINT('Ctrl Pts',(72.5856660738486,-9.99577296064053,
58.0520280822776));
#173640=CARTESIAN_POINT('Ctrl Pts',(72.4662981431576,-9.99122903863457,
58.0716581122195));
#173641=CARTESIAN_POINT('Ctrl Pts',(71.8382485224242,-9.95574377442191,
58.1746775120596));
#173642=CARTESIAN_POINT('Ctrl Pts',(71.332275642921,-9.88711017454876,58.2568035286751));
#173643=CARTESIAN_POINT('Ctrl Pts',(70.4149954224508,-9.68853418958247,
58.4059584866381));
#173644=CARTESIAN_POINT('Ctrl Pts',(70.002446261913,-9.57034611044422,58.473140665632));
#173645=CARTESIAN_POINT('Ctrl Pts',(69.475798030153,-9.38119460952537,58.5593936039634));
#173646=CARTESIAN_POINT('Ctrl Pts',(69.3536395505551,-9.3345336323122,58.5794337231402));
#173647=CARTESIAN_POINT('Ctrl Pts',(69.1799689677899,-9.26417482849022,
58.6079747962927));
#173648=CARTESIAN_POINT('Ctrl Pts',(69.1276840931917,-9.24246267624203,
58.6165739109851));
#173649=CARTESIAN_POINT('Ctrl Pts',(69.0369436745227,-9.20385471888833,
58.6315091405707));
#173650=CARTESIAN_POINT('Ctrl Pts',(68.9984045297915,-9.18716346753873,
58.6378560425308));
#173651=CARTESIAN_POINT('Ctrl Pts',(68.9191198423403,-9.15221778039782,
58.6509206101879));
#173652=CARTESIAN_POINT('Ctrl Pts',(68.8783890760657,-9.13393149665779,
58.6576363084923));
#173653=CARTESIAN_POINT('Ctrl Pts',(68.7740672659082,-9.08623583337875,
58.6748471125024));
#173654=CARTESIAN_POINT('Ctrl Pts',(68.7106608202108,-9.05642001868879,
58.6853175976995));
#173655=CARTESIAN_POINT('Ctrl Pts',(68.4529010933933,-8.93181945359217,
58.7279200086083));
#173656=CARTESIAN_POINT('Ctrl Pts',(68.2613403139167,-8.83127078516811,
58.7596712853618));
#173657=CARTESIAN_POINT('Ctrl Pts',(67.5867832372689,-8.44825033328149,
58.8716923656468));
#173658=CARTESIAN_POINT('Ctrl Pts',(67.1244353361462,-8.13076970883627,
58.9489368434906));
#173659=CARTESIAN_POINT('Ctrl Pts',(66.5515050109661,-7.66113969389995,
59.0437393520847));
#173660=CARTESIAN_POINT('Ctrl Pts',(66.4151940803343,-7.54304802082542,
59.066211621884));
#173661=CARTESIAN_POINT('Ctrl Pts',(66.2024587130554,-7.34836727730175,
59.1010578819761));
#173662=CARTESIAN_POINT('Ctrl Pts',(66.1239772493992,-7.27416411882655,
59.1138613557963));
#173663=CARTESIAN_POINT('Ctrl Pts',(66.020283563421,-7.17288189485434,59.1306897887546));
#173664=CARTESIAN_POINT('Ctrl Pts',(65.9940129064589,-7.14693565865169,
59.1349454501724));
#173665=CARTESIAN_POINT('Ctrl Pts',(65.9505646042505,-7.10354506535806,
59.1419698335437));
#173666=CARTESIAN_POINT('Ctrl Pts',(65.933307466961,-7.08618363545235,59.1447561301731));
#173667=CARTESIAN_POINT('Ctrl Pts',(65.9006600671254,-7.05309656307589,
59.1500199472768));
#173668=CARTESIAN_POINT('Ctrl Pts',(65.8852578349303,-7.03738342126679,
59.1525001552024));
#173669=CARTESIAN_POINT('Ctrl Pts',(65.8443266233363,-6.99534909116079,
59.1590831842411));
#173670=CARTESIAN_POINT('Ctrl Pts',(65.8188888331638,-6.96893643795431,
59.1631659323899));
#173671=CARTESIAN_POINT('Ctrl Pts',(65.7260282901543,-6.8714488235828,59.1780405856725));
#173672=CARTESIAN_POINT('Ctrl Pts',(65.6594915527174,-6.79950845535027,
59.1886411877593));
#173673=CARTESIAN_POINT('Ctrl Pts',(65.2682083459048,-6.36376760191899,
59.2506854862593));
#173674=CARTESIAN_POINT('Ctrl Pts',(64.9690019957253,-5.97718409652332,
59.2969223037193));
#173675=CARTESIAN_POINT('Ctrl Pts',(64.4820929619994,-5.24292591026478,
59.3713729644349));
#173676=CARTESIAN_POINT('Ctrl Pts',(64.2844585657862,-4.90321920214682,
59.40127276137));
#173677=CARTESIAN_POINT('Ctrl Pts',(64.0504444438035,-4.4405409171905,59.4365137785057));
#173678=CARTESIAN_POINT('Ctrl Pts',(63.9958559312707,-4.32739695139035,
59.4447187310132));
#173679=CARTESIAN_POINT('Ctrl Pts',(63.9200046964509,-4.16235183274881,
59.4560996843544));
#173680=CARTESIAN_POINT('Ctrl Pts',(63.8970407421879,-4.11126453786561,
59.4595423884426));
#173681=CARTESIAN_POINT('Ctrl Pts',(63.8575157325095,-4.02133402450607,
59.4654628737801));
#173682=CARTESIAN_POINT('Ctrl Pts',(63.8407710571365,-3.98257497481352,
59.4679694160702));
#173683=CARTESIAN_POINT('Ctrl Pts',(63.806478922087,-3.90180678617291,59.473099166708));
#173684=CARTESIAN_POINT('Ctrl Pts',(63.7889714103401,-3.85978134686698,
59.4757161218222));
#173685=CARTESIAN_POINT('Ctrl Pts',(63.7442102713071,-3.7502492135287,59.4824014704031));
#173686=CARTESIAN_POINT('Ctrl Pts',(63.7174010286647,-3.68255964634962,
59.4864002347442));
#173687=CARTESIAN_POINT('Ctrl Pts',(63.6075193260636,-3.39609343517798,
59.5027648311992));
#173688=CARTESIAN_POINT('Ctrl Pts',(63.5313270261378,-3.17469714629436,
59.5140514019717));
#173689=CARTESIAN_POINT('Ctrl Pts',(63.2973269190406,-2.40921389201419,
59.5483745945473));
#173690=CARTESIAN_POINT('Ctrl Pts',(63.1775481661048,-1.85438684178791,
59.5653567652896));
#173691=CARTESIAN_POINT('Ctrl Pts',(63.0598574046051,-0.946967874140944,
59.5789299855943));
#173692=CARTESIAN_POINT('Ctrl Pts',(63.0328413169354,-0.599497723594773,
59.5808302493471));
#173693=CARTESIAN_POINT('Ctrl Pts',(63.0223514195684,-0.202514087150256,
59.5788164213045));
#173694=CARTESIAN_POINT('Ctrl Pts',(63.0214117882815,-0.153682582570271,
59.5784965442126));
#173695=CARTESIAN_POINT('Ctrl Pts',(63.020509351098,-0.0788965070287953,
59.5778943145523));
#173696=CARTESIAN_POINT('Ctrl Pts',(63.0202951359107,-0.052945302010251,
59.5776646261293));
#173697=CARTESIAN_POINT('Ctrl Pts',(63.0201398336951,-0.0179958244278507,
59.577327158151));
#173698=CARTESIAN_POINT('Ctrl Pts',(63.020111739358,-0.00899790371852897,
59.5772377635995));
#173699=CARTESIAN_POINT('Ctrl Pts',(63.0200955324887,6.3021835685309E-11,
59.5771458498765));
#173700=CARTESIAN_POINT('Origin',(71.1115577432812,0.,47.8784035486295));
#173701=CARTESIAN_POINT('',(64.0306785352666,-5.86505158422741,49.6545847421392));
#173702=CARTESIAN_POINT('Origin',(71.2017879831895,0.,48.390124667801));
#173703=CARTESIAN_POINT('Ctrl Pts',(61.9506556875219,-4.3047803149361,49.4937177486876));
#173704=CARTESIAN_POINT('Ctrl Pts',(62.2558206002957,-4.61623330510467,
49.5206334656356));
#173705=CARTESIAN_POINT('Ctrl Pts',(62.5832897840105,-4.90076464302932,
49.547843602726));
#173706=CARTESIAN_POINT('Ctrl Pts',(63.2824918720409,-5.42189876047775,
49.6025356820337));
#173707=CARTESIAN_POINT('Ctrl Pts',(63.6484713972954,-5.65428821703993,
49.6296108874038));
#173708=CARTESIAN_POINT('Ctrl Pts',(64.0306785258525,-5.86505159962108,
49.6545847362842));
#173709=CARTESIAN_POINT('',(80.8588354304983,2.85105345906058E-13,46.3896787948389));
#173710=CARTESIAN_POINT('Ctrl Pts',(64.6378450224609,-7.86451166255203,
49.0198937666656));
#173711=CARTESIAN_POINT('Ctrl Pts',(65.5842187461411,-8.63596418606187,
48.8664417213224));
#173712=CARTESIAN_POINT('Ctrl Pts',(66.665244343586,-9.22997942887594,48.6898268456387));
#173713=CARTESIAN_POINT('Ctrl Pts',(68.7747317454522,-9.93701681694214,
48.3390049827969));
#173714=CARTESIAN_POINT('Ctrl Pts',(69.7756131305846,-10.1127840631434,
48.1705755632247));
#173715=CARTESIAN_POINT('Ctrl Pts',(72.216831965991,-10.1565930546866,47.7638481135821));
#173716=CARTESIAN_POINT('Ctrl Pts',(73.5290184110035,-9.86044398257961,
47.5496328656722));
#173717=CARTESIAN_POINT('Ctrl Pts',(75.8074028357543,-8.93620081766558,
47.1739853063171));
#173718=CARTESIAN_POINT('Ctrl Pts',(76.875925036593,-8.24881812823009,46.9959483360242));
#173719=CARTESIAN_POINT('Ctrl Pts',(78.8289563773398,-6.37831825034712,
46.6778185170246));
#173720=CARTESIAN_POINT('Ctrl Pts',(79.5456376526136,-5.24822323308914,
46.5682067541693));
#173721=CARTESIAN_POINT('Ctrl Pts',(80.2581416878816,-3.61460952657338,
46.4612355483114));
#173722=CARTESIAN_POINT('Ctrl Pts',(80.4496406732615,-3.04167150164063,
46.4332669072356));
#173723=CARTESIAN_POINT('Ctrl Pts',(80.736121211927,-1.83560492013537,46.3940854916214));
#173724=CARTESIAN_POINT('Ctrl Pts',(80.8744849978637,-0.999929053673554,
46.3765472486026));
#173725=CARTESIAN_POINT('Ctrl Pts',(80.8588354304983,5.39845945723982E-13,
46.3896787948389));
#173726=CARTESIAN_POINT('',(81.2058372116564,-1.25526296912604E-15,46.0985097275438));
#173727=CARTESIAN_POINT('Ctrl Pts',(80.8588354304983,5.47409340079241E-13,
46.3896787948389));
#173728=CARTESIAN_POINT('Ctrl Pts',(80.8552340384864,0.230110930372039,
46.3927007215552));
#173729=CARTESIAN_POINT('Ctrl Pts',(80.8433646224346,0.468917934731292,
46.3974082864174));
#173730=CARTESIAN_POINT('Ctrl Pts',(80.7059853381663,2.01312934365047,46.4391509714778));
#173731=CARTESIAN_POINT('Ctrl Pts',(80.3339343657837,3.27999513199469,46.5206449108692));
#173732=CARTESIAN_POINT('Ctrl Pts',(79.4591112270451,4.96117031922987,46.6937471773202));
#173733=CARTESIAN_POINT('Ctrl Pts',(79.1359999079507,5.46514833664704,46.7562038675566));
#173734=CARTESIAN_POINT('Ctrl Pts',(77.9119991335175,7.03455036712757,46.9907537556784));
#173735=CARTESIAN_POINT('Ctrl Pts',(76.9694568196666,7.75538512274565,47.1711076777577));
#173736=CARTESIAN_POINT('Ctrl Pts',(75.2419357532795,8.79481324655818,47.499283653396));
#173737=CARTESIAN_POINT('Ctrl Pts',(74.2128668963147,9.19433759694196,47.6920275536023));
#173738=CARTESIAN_POINT('Ctrl Pts',(72.605135482623,9.51488062321757,47.9910034564073));
#173739=CARTESIAN_POINT('Ctrl Pts',(72.0575858302653,9.57463114299576,48.0926072795593));
#173740=CARTESIAN_POINT('Ctrl Pts',(70.1521659122945,9.60900492598336,48.4482545044341));
#173741=CARTESIAN_POINT('Ctrl Pts',(68.9147695441831,9.32689482673615,48.6834345344816));
#173742=CARTESIAN_POINT('Ctrl Pts',(66.8402588659947,8.48044663053028,49.0744129611521));
#173743=CARTESIAN_POINT('Ctrl Pts',(65.8928670853075,7.88377482069447,49.2515523539232));
#173744=CARTESIAN_POINT('Ctrl Pts',(64.1751301883544,6.30870724482377,49.5779460890239));
#173745=CARTESIAN_POINT('Ctrl Pts',(63.6087131950866,5.46229732862544,49.6908447836293));
#173746=CARTESIAN_POINT('Ctrl Pts',(62.8054838250294,4.0282503011191,49.8519237176284));
#173747=CARTESIAN_POINT('Ctrl Pts',(62.4739050278201,3.16727015018886,49.9201710396792));
#173748=CARTESIAN_POINT('Ctrl Pts',(62.2702697970345,2.27382383776023,49.9649923034));
#173749=CARTESIAN_POINT('Origin',(72.3389200802052,-4.33680868994202E-16,
54.8391212561108));
#173750=CARTESIAN_POINT('',(80.8412511893021,-3.85114170205159,53.0468024688033));
#173751=CARTESIAN_POINT('',(62.6457011510073,-8.83286634079036E-15,56.4456612375439));
#173752=CARTESIAN_POINT('Ctrl Pts',(62.6457011510073,1.4432899320127E-14,
56.4456612375439));
#173753=CARTESIAN_POINT('Ctrl Pts',(62.6558818028268,1.2588196834612,56.4371186563363));
#173754=CARTESIAN_POINT('Ctrl Pts',(62.9068166598699,2.3426378835086,56.3841671741036));
#173755=CARTESIAN_POINT('Ctrl Pts',(63.3895004888157,3.72170130583507,56.2902490190701));
#173756=CARTESIAN_POINT('Ctrl Pts',(63.6188721136369,4.23445645416726,56.246865015372));
#173757=CARTESIAN_POINT('Ctrl Pts',(64.3236027030591,5.50911067298779,56.1159109714176));
#173758=CARTESIAN_POINT('Ctrl Pts',(65.0460461515127,6.57626816176057,55.9846336701387));
#173759=CARTESIAN_POINT('Ctrl Pts',(67.1241688952235,8.25959511912813,55.600727527555));
#173760=CARTESIAN_POINT('Ctrl Pts',(68.1153344812789,8.80727618002418,55.4182675813396));
#173761=CARTESIAN_POINT('Ctrl Pts',(70.1652119838017,9.51224353360967,55.046367693855));
#173762=CARTESIAN_POINT('Ctrl Pts',(71.3752373091251,9.74662388873713,54.8298371513194));
#173763=CARTESIAN_POINT('Ctrl Pts',(73.9983723123867,9.59906696956911,54.3510038345899));
#173764=CARTESIAN_POINT('Ctrl Pts',(75.2412925532651,9.26681056744937,54.1219257269736));
#173765=CARTESIAN_POINT('Ctrl Pts',(77.4110681835218,8.19401660720014,53.7267754853011));
#173766=CARTESIAN_POINT('Ctrl Pts',(78.3513233293596,7.49763695817288,53.5574829999965));
#173767=CARTESIAN_POINT('Ctrl Pts',(79.9997511629273,5.71009860563118,53.2525982152993));
#173768=CARTESIAN_POINT('Ctrl Pts',(80.6675890443261,4.60317191979347,53.1250053406627));
#173769=CARTESIAN_POINT('Ctrl Pts',(81.4593335541564,2.42846581422788,52.9736249621716));
#173770=CARTESIAN_POINT('Ctrl Pts',(81.6594257029317,1.39833823602532,52.935032235611));
#173771=CARTESIAN_POINT('Ctrl Pts',(81.7086205819825,-0.363183533732222,
52.9176503833502));
#173772=CARTESIAN_POINT('Ctrl Pts',(81.645129190087,-1.08304839861894,52.9237907714508));
#173773=CARTESIAN_POINT('Ctrl Pts',(81.3602107718099,-2.49761284659637,
52.9640327929444));
#173774=CARTESIAN_POINT('Ctrl Pts',(81.1375058307725,-3.19089770223702,
52.9985048418238));
#173775=CARTESIAN_POINT('Ctrl Pts',(80.8412511898528,-3.85114170233543,
53.0468024683008));
#173776=CARTESIAN_POINT('',(77.6076111848316,-7.81540780901842,53.6169804474894));
#173777=CARTESIAN_POINT('Origin',(72.288792169145,-4.33680868994202E-16,
54.55483174546));
#173778=CARTESIAN_POINT('Origin',(1.36168634987441,-56.100840902432,65.8484117826429));
#173779=CARTESIAN_POINT('Ctrl Pts',(76.6496952865774,-8.9910764663851,54.0790152794584));
#173780=CARTESIAN_POINT('Ctrl Pts',(75.4612431654612,-9.5637074614093,54.2810582811977));
#173781=CARTESIAN_POINT('Ctrl Pts',(74.166995732845,-9.89613305269025,54.5052439135236));
#173782=CARTESIAN_POINT('Ctrl Pts',(71.3800140752479,-10.0235187484533,
54.9838678620627));
#173783=CARTESIAN_POINT('Ctrl Pts',(70.0865581450753,-9.73932742333592,
55.2011833834671));
#173784=CARTESIAN_POINT('Ctrl Pts',(67.866731806019,-8.91204338453401,55.5785455713441));
#173785=CARTESIAN_POINT('Ctrl Pts',(66.7699239004441,-8.24310830719802,
55.7676027583461));
#173786=CARTESIAN_POINT('Ctrl Pts',(64.7456933822644,-6.38037642119864,
56.1118241547508));
#173787=CARTESIAN_POINT('Ctrl Pts',(64.0299445336693,-5.2602300440886,56.2276516472125));
#173788=CARTESIAN_POINT('Ctrl Pts',(63.0420874263768,-3.11680606634751,
56.3884754344893));
#173789=CARTESIAN_POINT('Ctrl Pts',(62.7309508857847,-1.88072460747348,
56.4393114111633));
#173790=CARTESIAN_POINT('Ctrl Pts',(62.6487768516383,-0.412225399740427,
56.4472167150806));
#173791=CARTESIAN_POINT('Ctrl Pts',(62.6440527780866,-0.203818411142372,
56.4470443866571));
#173792=CARTESIAN_POINT('Ctrl Pts',(62.6457011510073,1.80064296806393E-14,
56.4456612375439));
#173793=CARTESIAN_POINT('',(62.4908425500831,-1.65832766814155E-15,56.5756030327798));
#173794=CARTESIAN_POINT('Origin',(73.035119430904,-4.33680868994202E-16,
58.7874639765594));
#173795=CARTESIAN_POINT('',(65.3160352562258,5.15420400344998E-16,59.6408334769718));
#173796=CARTESIAN_POINT('',(80.5805554279152,-1.3827821383334E-15,56.9492867231348));
#173797=CARTESIAN_POINT('Origin',(72.9482953420705,-4.33680868994202E-16,
58.2950601000533));
#173798=CARTESIAN_POINT('',(80.3548127969482,-1.3827821383334E-15,55.6690366442189));
#173799=CARTESIAN_POINT('',(80.6673795167487,-1.3827821383334E-15,57.4416905996409));
#173800=CARTESIAN_POINT('Origin',(72.7225527111036,-4.33680868994202E-16,
57.0148100211374));
#173801=CARTESIAN_POINT('Origin',(72.9482953420705,-4.33680868994202E-16,
58.2950601000533));
#173802=CARTESIAN_POINT('Origin',(73.035119430904,-8.67361737988404E-16,
58.7874639765594));
#173803=CARTESIAN_POINT('',(79.0803910612662,-1.66338215743418E-15,55.6398949280495));
#173804=CARTESIAN_POINT('Origin',(72.6791406666868,-8.67361737988404E-16,
56.7686080828844));
#173805=CARTESIAN_POINT('',(78.3423863061819,-1.66338215743418E-15,51.4544619777476));
#173806=CARTESIAN_POINT('',(79.4363698254834,-1.66338215743418E-15,57.6587508217245));
#173807=CARTESIAN_POINT('Origin',(71.9411359116025,-8.67361737988404E-16,
52.5831751325825));
#173808=CARTESIAN_POINT('Origin',(72.6791406666868,-8.67361737988404E-16,
56.7686080828844));
#173809=CARTESIAN_POINT('',(79.370005043936,-1.69399832741288E-15,55.8426848218858));
#173810=CARTESIAN_POINT('Origin',(72.7225527111036,-8.67361737988404E-16,
57.0148100211374));
#173811=CARTESIAN_POINT('Origin',(79.3265929995192,-1.69399832741287E-15,
55.5964828836328));
#173812=CARTESIAN_POINT('Origin',(72.9482953420705,-4.33680868994202E-16,
58.2950601000533));
#173813=CARTESIAN_POINT('',(64.9104554685532,-1.44401447829076E-15,60.2200614423113));
#173814=CARTESIAN_POINT('Origin',(64.8236313797197,-1.44401447829077E-15,
59.7276575658052));
#173815=CARTESIAN_POINT('Origin',(73.035119430904,-4.33680868994202E-16,
58.7874639765594));
#173816=CARTESIAN_POINT('Origin',(74.4590344877726,0.,66.8628875512595));
#173817=CARTESIAN_POINT('',(69.479116529072,-3.1224989991992,53.0172955767497));
#173818=CARTESIAN_POINT('',(69.479116529072,3.1224989991992,53.0172955767497));
#173819=CARTESIAN_POINT('Origin',(71.9411359116025,0.,52.5831751325825));
#173820=CARTESIAN_POINT('',(69.0102664493713,-3.1224989991992,50.3583146436167));
#173821=CARTESIAN_POINT('',(71.997015105242,-3.1224989991992,67.2970079954268));
#173822=CARTESIAN_POINT('',(69.0102664493713,3.1224989991992,50.3583146436167));
#173823=CARTESIAN_POINT('Origin',(71.4722858319019,0.,49.9241941994495));
#173824=CARTESIAN_POINT('',(71.997015105242,3.1224989991992,67.2970079954268));
#173825=CARTESIAN_POINT('Origin',(73.035119430904,-4.33680868994202E-16,
58.7874639765594));
#173826=CARTESIAN_POINT('Origin',(73.035119430904,-4.33680868994202E-16,
58.7874639765594));
#173827=CARTESIAN_POINT('Ctrl Pts',(64.0263520775732,-2.56296981511825,
60.3759527238769));
#173828=CARTESIAN_POINT('Ctrl Pts',(63.7875845097259,-1.77172877889257,
60.4006974385262));
#173829=CARTESIAN_POINT('Ctrl Pts',(63.6565142256614,-0.956392695659807,
60.4105594712462));
#173830=CARTESIAN_POINT('Ctrl Pts',(63.6035905069927,0.30360001951426,60.3883547596279));
#173831=CARTESIAN_POINT('Ctrl Pts',(63.611715312006,0.743305782075929,60.3733985025284));
#173832=CARTESIAN_POINT('Ctrl Pts',(63.7164166135911,1.97589461027358,60.3151289341474));
#173833=CARTESIAN_POINT('Ctrl Pts',(63.879562647937,2.75611408109453,60.2597360604376));
#173834=CARTESIAN_POINT('Ctrl Pts',(64.5648131938851,4.72056632679071,60.0820156254564));
#173835=CARTESIAN_POINT('Ctrl Pts',(65.227248808725,5.8102138204816,59.9468224778353));
#173836=CARTESIAN_POINT('Ctrl Pts',(66.7215046807206,7.47366464069322,59.6286908078873));
#173837=CARTESIAN_POINT('Ctrl Pts',(67.4441302929274,8.0844582883649,59.4676839220779));
#173838=CARTESIAN_POINT('Ctrl Pts',(68.6416845804107,8.81513527266344,59.2149470199522));
#173839=CARTESIAN_POINT('Ctrl Pts',(69.043883161962,9.0215869125654,59.1317880463288));
#173840=CARTESIAN_POINT('Ctrl Pts',(70.9344218775917,9.82102618121542,58.7492604909112));
#173841=CARTESIAN_POINT('Ctrl Pts',(72.2569812764208,9.93197375381987,58.4985556012195));
#173842=CARTESIAN_POINT('Ctrl Pts',(73.7464228758253,9.9476694037475,58.1960089508397));
#173843=CARTESIAN_POINT('Ctrl Pts',(74.3790867245964,9.89542960221607,58.063113491427));
#173844=CARTESIAN_POINT('Ctrl Pts',(75.0041293597107,9.77968000098264,57.9325610961289));
#173845=CARTESIAN_POINT('Ctrl Pts',(72.8461347155083,9.99946198871296,58.3130737055659));
#173846=CARTESIAN_POINT('Ctrl Pts',(71.9149068124353,9.98320644558344,58.4838062328919));
#173847=CARTESIAN_POINT('Ctrl Pts',(70.9897556457315,9.82983607379267,58.6559080466542));
#173848=CARTESIAN_POINT('Ctrl Pts',(69.5021320403036,9.3582570208983,58.930684869102));
#173849=CARTESIAN_POINT('Ctrl Pts',(68.9219285900236,9.11090652668606,59.0373716283145));
#173850=CARTESIAN_POINT('Ctrl Pts',(67.5783941095989,8.37896837345306,59.2833197292783));
#173851=CARTESIAN_POINT('Ctrl Pts',(66.8474154851385,7.84011641204557,59.4160341187888));
#173852=CARTESIAN_POINT('Ctrl Pts',(65.2642516723813,6.28883638723455,59.7091484603951));
#173853=CARTESIAN_POINT('Ctrl Pts',(64.5212429759071,5.18470424453446,59.8532670983327));
#173854=CARTESIAN_POINT('Ctrl Pts',(63.5478969272612,2.87521845013382,60.0418329593114));
#173855=CARTESIAN_POINT('Ctrl Pts',(63.2799418969696,1.6982627346725,60.0936703250998));
#173856=CARTESIAN_POINT('Ctrl Pts',(63.1657385233228,-0.917901988626705,
60.1290073346147));
#173857=CARTESIAN_POINT('Ctrl Pts',(63.4167115584965,-2.22103464168441,
60.0982490330575));
#173858=CARTESIAN_POINT('Ctrl Pts',(64.2574469136842,-4.53354012896003,
59.9683289205253));
#173859=CARTESIAN_POINT('Ctrl Pts',(64.9136511838193,-5.6373681902584,59.8580788638135));
#173860=CARTESIAN_POINT('Ctrl Pts',(66.6986338989128,-7.63000409523024,
59.5591622625367));
#173861=CARTESIAN_POINT('Ctrl Pts',(67.7775303758803,-8.37226083492883,
59.3819682455633));
#173862=CARTESIAN_POINT('Ctrl Pts',(69.9524651194837,-9.39905901463539,
59.0158642552059));
#173863=CARTESIAN_POINT('Ctrl Pts',(71.1596155168285,-9.70968120699252,
58.8080610233883));
#173864=CARTESIAN_POINT('Ctrl Pts',(73.3729201406308,-9.83583275513113,
58.43066506375));
#173865=CARTESIAN_POINT('Ctrl Pts',(74.3575262345018,-9.73497309686251,
58.2662251899724));
#173866=CARTESIAN_POINT('Ctrl Pts',(76.3782480250941,-9.20815341290068,
57.9276702428763));
#173867=CARTESIAN_POINT('Ctrl Pts',(77.3972451749448,-8.74454053614141,
57.7553593824384));
#173868=CARTESIAN_POINT('Ctrl Pts',(78.6753907266003,-7.87164291992839,
57.5382919268542));
#173869=CARTESIAN_POINT('Ctrl Pts',(79.0201448012645,-7.60006937811386,
57.4797430645897));
#173870=CARTESIAN_POINT('Ctrl Pts',(80.3839454547407,-6.36466254602424,
57.2501127656707));
#173871=CARTESIAN_POINT('Ctrl Pts',(81.1129231951604,-5.29014523519362,
57.1344711030446));
#173872=CARTESIAN_POINT('Ctrl Pts',(81.992728202448,-3.42226759385829,56.994493242659));
#173873=CARTESIAN_POINT('Ctrl Pts',(82.2662184197964,-2.54642331504456,
56.9511812568696));
#173874=CARTESIAN_POINT('Ctrl Pts',(82.4839371806097,-1.23056618564693,
56.9195544439548));
#173875=CARTESIAN_POINT('Ctrl Pts',(82.5259926495773,-0.810139400801797,
56.9142786692208));
#173876=CARTESIAN_POINT('Ctrl Pts',(82.5450936724779,-0.258026219139575,
56.9142906530356));
#173877=CARTESIAN_POINT('Ctrl Pts',(82.5469438787143,-0.128531025228586,
56.9147998423219));
#173878=CARTESIAN_POINT('Ctrl Pts',(82.5462364601441,-3.03547362939804E-8,
56.915810141241));
#173879=CARTESIAN_POINT('Origin',(69.9094522328998,0.,41.0609244223396));
#173880=CARTESIAN_POINT('',(60.0036718763913,-9.6034686896093E-16,42.5716136120261));
#173881=CARTESIAN_POINT('Ctrl Pts',(60.0036718763913,-9.71445146547012E-15,
42.5716136120261));
#173882=CARTESIAN_POINT('Ctrl Pts',(60.015100851557,1.12076762514684,42.5552913438929));
#173883=CARTESIAN_POINT('Ctrl Pts',(60.2126873206611,2.13839800656458,42.5043854450878));
#173884=CARTESIAN_POINT('Ctrl Pts',(60.9006318822312,4.25527362975578,42.352347691539));
#173885=CARTESIAN_POINT('Ctrl Pts',(61.5373356061649,5.40491193212032,42.2258291698478));
#173886=CARTESIAN_POINT('Ctrl Pts',(63.2842977147422,7.47099370248614,41.8858881841359));
#173887=CARTESIAN_POINT('Ctrl Pts',(64.3217540848946,8.2258424335728,41.683036578767));
#173888=CARTESIAN_POINT('Ctrl Pts',(66.451028591047,9.32975004786528,41.2743904466553));
#173889=CARTESIAN_POINT('Ctrl Pts',(67.6946653135831,9.68938228252847,41.0411463826451));
#173890=CARTESIAN_POINT('Ctrl Pts',(70.249425026084,9.89392953488958,40.5602284082465));
#173891=CARTESIAN_POINT('Ctrl Pts',(71.3809810751992,9.72068069599538,40.3427593588294));
#173892=CARTESIAN_POINT('Ctrl Pts',(73.2715781015043,9.17865716757742,39.9806019499236));
#173893=CARTESIAN_POINT('Ctrl Pts',(74.1892182222798,8.75151497853075,39.8057754039733));
#173894=CARTESIAN_POINT('Ctrl Pts',(75.4581963738792,7.89714843430856,39.5638811008101));
#173895=CARTESIAN_POINT('Ctrl Pts',(75.868825936961,7.5689631723131,39.4854636028735));
#173896=CARTESIAN_POINT('Ctrl Pts',(77.2483266748846,6.26457595469469,39.2185396485213));
#173897=CARTESIAN_POINT('Ctrl Pts',(77.9577795744693,5.18258137974227,39.0727146413577));
#173898=CARTESIAN_POINT('Ctrl Pts',(78.8596251672318,3.1507044373941,38.8836436555022));
#173899=CARTESIAN_POINT('Ctrl Pts',(79.131437675942,2.12458558215186,38.8239526068959));
#173900=CARTESIAN_POINT('Ctrl Pts',(79.3692586925281,-0.323481828215834,
38.7530699483904));
#173901=CARTESIAN_POINT('Ctrl Pts',(79.1854889076528,-1.5955261956348,38.7654352018601));
#173902=CARTESIAN_POINT('Ctrl Pts',(78.5652621680601,-3.63454258061496,
38.8438640005469));
#173903=CARTESIAN_POINT('Ctrl Pts',(78.1275440032739,-4.54476502256378,
38.9083134454724));
#173904=CARTESIAN_POINT('Ctrl Pts',(77.2671455806108,-5.79308784648288,
39.0418902563234));
#173905=CARTESIAN_POINT('Ctrl Pts',(76.9402683789618,-6.19380668058799,
39.0934590420892));
#173906=CARTESIAN_POINT('Ctrl Pts',(75.7122858853336,-7.467828066414,39.2868961783433));
#173907=CARTESIAN_POINT('Ctrl Pts',(74.6693898303905,-8.18345984132722,
39.4501703743754));
#173908=CARTESIAN_POINT('Ctrl Pts',(72.5648273975363,-9.08634426397409,
39.7900363806716));
#173909=CARTESIAN_POINT('Ctrl Pts',(71.539508412694,-9.3357772537295,39.9591202037972));
#173910=CARTESIAN_POINT('Ctrl Pts',(69.2592631600181,-9.48947083365311,
40.3326286562384));
#173911=CARTESIAN_POINT('Ctrl Pts',(68.1626906187745,-9.30992149226666,
40.5078344866331));
#173912=CARTESIAN_POINT('Ctrl Pts',(66.3499023071681,-8.76459892370793,
40.7990369030172));
#173913=CARTESIAN_POINT('Ctrl Pts',(65.4869193623454,-8.3529885143117,40.9385799356877));
#173914=CARTESIAN_POINT('Ctrl Pts',(64.7021225437138,-7.81768501306327,
41.065233192728));
#173915=CARTESIAN_POINT('Ctrl Pts',(76.8678595013252,-7.42547303891627,
39.8339694781584));
#173916=CARTESIAN_POINT('Ctrl Pts',(76.2996665754096,-7.93011918472383,
39.9050608108253));
#173917=CARTESIAN_POINT('Ctrl Pts',(75.6825187982154,-8.37119663038465,
39.9887641400102));
#173918=CARTESIAN_POINT('Ctrl Pts',(74.4558505579195,-9.04934668012714,
40.1542389939804));
#173919=CARTESIAN_POINT('Ctrl Pts',(73.8654202486675,-9.30370903464973,
40.2335728392658));
#173920=CARTESIAN_POINT('Ctrl Pts',(72.2903388606086,-9.80223571367267,
40.441283110937));
#173921=CARTESIAN_POINT('Ctrl Pts',(71.2931850079593,-9.95167476081707,
40.5682944419678));
#173922=CARTESIAN_POINT('Ctrl Pts',(69.4560555737328,-9.95340529705847,
40.8124145716253));
#173923=CARTESIAN_POINT('Ctrl Pts',(68.0374687632394,-9.86536563346914,
41.0176380044774));
#173924=CARTESIAN_POINT('Ctrl Pts',(65.5125902514186,-8.79704444319692,
41.3538217666584));
#173925=CARTESIAN_POINT('Ctrl Pts',(64.6573596433338,-8.25918115529596,
41.4580511199009));
#173926=CARTESIAN_POINT('Ctrl Pts',(63.4723018145351,-7.22572972472362,
41.5943541895369));
#173927=CARTESIAN_POINT('Ctrl Pts',(63.0784912802987,-6.81814121716002,
41.6388112706362));
#173928=CARTESIAN_POINT('Ctrl Pts',(61.9669303031546,-5.46050870597522,
41.7656919416805));
#173929=CARTESIAN_POINT('Ctrl Pts',(61.3871579820319,-4.41116939664101,
41.8264853738403));
#173930=CARTESIAN_POINT('Ctrl Pts',(60.7520023897809,-2.43621381970203,
41.8462181459636));
#173931=CARTESIAN_POINT('Ctrl Pts',(60.6035823151644,-1.57716493704874,
41.8289274144168));
#173932=CARTESIAN_POINT('Ctrl Pts',(60.5714935134192,-0.70586883869046,
41.7935745403973));
#173933=CARTESIAN_POINT('Ctrl Pts',(72.9974833261206,-9.75859007406184,
40.5164212233382));
#173934=CARTESIAN_POINT('Ctrl Pts',(72.1680866689036,-10.0182427508679,
40.6526096763793));
#173935=CARTESIAN_POINT('Ctrl Pts',(71.3084745515891,-10.1699514565876,
40.7953672456757));
#173936=CARTESIAN_POINT('Ctrl Pts',(69.096234136181,-10.2640179840406,41.1594237519536));
#173937=CARTESIAN_POINT('Ctrl Pts',(67.8768440048148,-10.0398244678189,
41.3550739449956));
#173938=CARTESIAN_POINT('Ctrl Pts',(65.5868797574183,-9.26087437006304,
41.725821401744));
#173939=CARTESIAN_POINT('Ctrl Pts',(64.429406738187,-8.59349167447454,41.9157601187445));
#173940=CARTESIAN_POINT('Ctrl Pts',(62.3355503431521,-6.75255369228092,
42.2527084519859));
#173941=CARTESIAN_POINT('Ctrl Pts',(61.5631077787736,-5.64482332823591,
42.3683202081607));
#173942=CARTESIAN_POINT('Ctrl Pts',(60.4566040978486,-3.37627727188828,
42.5298683525699));
#173943=CARTESIAN_POINT('Ctrl Pts',(60.1092783965342,-2.07466361355572,
42.5774466901993));
#173944=CARTESIAN_POINT('Ctrl Pts',(60.0075858713322,-0.493629709332019,
42.5770362265899));
#173945=CARTESIAN_POINT('Ctrl Pts',(60.0011799984526,-0.244362777846393,
42.575172382544));
#173946=CARTESIAN_POINT('Ctrl Pts',(60.0036718763913,-6.10622663543836E-15,
42.5716136120261));
#173947=CARTESIAN_POINT('',(60.6263323388303,-1.1327982893212E-15,41.6823623120182));
#173948=CARTESIAN_POINT('',(59.8151727645246,-1.25526296912604E-15,42.8408182434253));
#173949=CARTESIAN_POINT('Origin',(69.7358040552328,0.,40.0761166693274));
#173950=CARTESIAN_POINT('Origin',(73.0915550886457,-4.33680868994202E-16,
59.1075264962884));
#173951=CARTESIAN_POINT('Ctrl Pts',(81.6610766756267,4.47259269587928E-12,
52.9993788854899));
#173952=CARTESIAN_POINT('Ctrl Pts',(81.6610722764663,-0.00232025445502517,
52.9993539366116));
#173953=CARTESIAN_POINT('Ctrl Pts',(81.661067045244,-0.00464051070797554,
52.9993291640552));
#173954=CARTESIAN_POINT('Ctrl Pts',(81.6609993686616,-0.0305384148304018,
52.9990546279118));
#173955=CARTESIAN_POINT('Ctrl Pts',(81.6608518350455,-0.054115947562142,
52.9988228830155));
#173956=CARTESIAN_POINT('Ctrl Pts',(81.6602425001029,-0.115647279179397,
52.9982651715894));
#173957=CARTESIAN_POINT('Ctrl Pts',(81.6596439234659,-0.153599559557272,
52.9979679311037));
#173958=CARTESIAN_POINT('Ctrl Pts',(81.6559699978132,-0.323336835080533,
52.9968448740763));
#173959=CARTESIAN_POINT('Ctrl Pts',(81.6504306382807,-0.455057219995967,
52.9965296115069));
#173960=CARTESIAN_POINT('Ctrl Pts',(81.6266559635856,-0.835254836627224,
52.9971545979555));
#173961=CARTESIAN_POINT('Ctrl Pts',(81.6015184647897,-1.08318716183554,
52.9994595362967));
#173962=CARTESIAN_POINT('Ctrl Pts',(81.474195624691,-1.98833237428493,53.0142996630001));
#173963=CARTESIAN_POINT('Ctrl Pts',(81.3137681540632,-2.63524327442574,
53.0373067696788));
#173964=CARTESIAN_POINT('Ctrl Pts',(81.0527830174814,-3.3569861251441,53.0756325690094));
#173965=CARTESIAN_POINT('Ctrl Pts',(81.0161192583185,-3.45347191784948,
53.0810339964031));
#173966=CARTESIAN_POINT('Ctrl Pts',(80.9584501697706,-3.5981461001753,53.089552188204));
#173967=CARTESIAN_POINT('Ctrl Pts',(80.9385925672861,-3.64679406876821,
53.092488995169));
#173968=CARTESIAN_POINT('Ctrl Pts',(80.9022225162372,-3.73383870110997,
53.0978741346783));
#173969=CARTESIAN_POINT('Ctrl Pts',(80.8858567197031,-3.77229655864622,
53.1002995016838));
#173970=CARTESIAN_POINT('Ctrl Pts',(80.8504034898739,-3.85411521597498,
53.1055580685769));
#173971=CARTESIAN_POINT('Ctrl Pts',(80.8312451048555,-3.89744331436159,
53.1084023826643));
#173972=CARTESIAN_POINT('Ctrl Pts',(80.7782437501906,-4.01494090251588,
53.1162783170956));
#173973=CARTESIAN_POINT('Ctrl Pts',(80.7437752410286,-4.08881713239427,
53.1214079609473));
#173974=CARTESIAN_POINT('Ctrl Pts',(80.5644807627053,-4.46060791753182,
53.1481310887594));
#173975=CARTESIAN_POINT('Ctrl Pts',(80.4052406243085,-4.75115004446838,
53.1719827824595));
#173976=CARTESIAN_POINT('Ctrl Pts',(80.0553836328029,-5.31746468070993,
53.224836143526));
#173977=CARTESIAN_POINT('Ctrl Pts',(79.8646680539399,-5.59262914290383,
53.2538583446598));
#173978=CARTESIAN_POINT('Ctrl Pts',(79.487921471852,-6.07933967601403,53.3120132898615));
#173979=CARTESIAN_POINT('Ctrl Pts',(79.3061523332329,-6.29380594126246,
53.3403692069814));
#173980=CARTESIAN_POINT('Ctrl Pts',(79.0749264208731,-6.54332446046129,
53.3770383702038));
#173981=CARTESIAN_POINT('Ctrl Pts',(79.0341547104778,-6.58650217127409,
53.3835253887303));
#173982=CARTESIAN_POINT('Ctrl Pts',(78.97272632313,-6.65034533360716,53.3933336964837));
#173983=CARTESIAN_POINT('Ctrl Pts',(78.9523697631261,-6.67130755192734,
53.3965896191447));
#173984=CARTESIAN_POINT('Ctrl Pts',(78.9155399574673,-6.70888447947886,
53.4024908438246));
#173985=CARTESIAN_POINT('Ctrl Pts',(78.8991009973588,-6.7255333291227,53.4051286087279));
#173986=CARTESIAN_POINT('Ctrl Pts',(78.8621076697072,-6.76272290145134,
53.4110728755343));
#173987=CARTESIAN_POINT('Ctrl Pts',(78.8415209041491,-6.78322958915602,
53.4143865479715));
#173988=CARTESIAN_POINT('Ctrl Pts',(78.7791598347458,-6.84477967856057,
53.4244404681999));
#173989=CARTESIAN_POINT('Ctrl Pts',(78.7371042565384,-6.88552595802291,
53.4312424413944));
#173990=CARTESIAN_POINT('Ctrl Pts',(78.6379734609746,-6.97980400347526,
53.447320443257));
#173991=CARTESIAN_POINT('Ctrl Pts',(78.5806122158642,-7.03301822335197,
53.4566578090453));
#173992=CARTESIAN_POINT('Ctrl Pts',(78.2327508384596,-7.34778625380926,
53.5134520550835));
#173993=CARTESIAN_POINT('Ctrl Pts',(77.9272003779144,-7.59155407372705,
53.564017729834));
#173994=CARTESIAN_POINT('Ctrl Pts',(77.6076111848315,-7.81540780901845,
53.6169804474894));
#173995=CARTESIAN_POINT('Ctrl Pts',(80.841251189302,-3.85114170205161,53.0468024688033));
#173996=CARTESIAN_POINT('Ctrl Pts',(80.8507779136793,-3.82942848242393,
53.0453809010695));
#173997=CARTESIAN_POINT('Ctrl Pts',(80.8602207064578,-3.80768840471765,
53.0439756042331));
#173998=CARTESIAN_POINT('Ctrl Pts',(80.8792048973429,-3.76353516228782,
53.0411580292377));
#173999=CARTESIAN_POINT('Ctrl Pts',(80.8887378829764,-3.74112938354105,
53.0397472097096));
#174000=CARTESIAN_POINT('Ctrl Pts',(80.9163307695015,-3.67558706517093,
53.0356755751662));
#174001=CARTESIAN_POINT('Ctrl Pts',(80.9341623540418,-3.63235242951933,
53.0330595355005));
#174002=CARTESIAN_POINT('Ctrl Pts',(80.982223849608,-3.51336899811502,53.0260511192625));
#174003=CARTESIAN_POINT('Ctrl Pts',(81.0118098928388,-3.43735710624604,
53.0217849107517));
#174004=CARTESIAN_POINT('Ctrl Pts',(81.183168553697,-2.98000080361263,52.9973720652675));
#174005=CARTESIAN_POINT('Ctrl Pts',(81.301710550912,-2.5901662948204,52.9817814278254));
#174006=CARTESIAN_POINT('Ctrl Pts',(81.4650039959974,-1.89866215450415,
52.9626858339964));
#174007=CARTESIAN_POINT('Ctrl Pts',(81.5207698692727,-1.6002609329892,52.9571167954222));
#174008=CARTESIAN_POINT('Ctrl Pts',(81.5807520080895,-1.16684122199171,
52.9525768273773));
#174009=CARTESIAN_POINT('Ctrl Pts',(81.5963630564538,-1.03360813536364,
52.9516575893418));
#174010=CARTESIAN_POINT('Ctrl Pts',(81.6236379970694,-0.749572634412603,
52.9506649274304));
#174011=CARTESIAN_POINT('Ctrl Pts',(81.6345423798266,-0.598733092378248,
52.9507142757853));
#174012=CARTESIAN_POINT('Ctrl Pts',(81.6464653136749,-0.353392227770225,
52.95167538014));
#174013=CARTESIAN_POINT('Ctrl Pts',(81.6496579259418,-0.259021630920684,
52.9522561509393));
#174014=CARTESIAN_POINT('Ctrl Pts',(81.6520988061173,-0.130967865973636,
52.9533185372138));
#174015=CARTESIAN_POINT('Ctrl Pts',(81.6525632048301,-0.0973118027878368,
52.9536234500613));
#174016=CARTESIAN_POINT('Ctrl Pts',(81.6530315026046,-0.0424365229063424,
52.954161815321));
#174017=CARTESIAN_POINT('Ctrl Pts',(81.6531421625657,-0.0212183265239835,
52.9543800258197));
#174018=CARTESIAN_POINT('Ctrl Pts',(81.653182392128,-1.2050098533051E-12,
52.9546081790047));
#174019=CARTESIAN_POINT('Origin',(69.6316151486327,0.,39.48523201752));
#174020=CARTESIAN_POINT('Ctrl Pts',(61.9717635125435,8.13085086909029E-10,
49.8885587101925));
#174021=CARTESIAN_POINT('Ctrl Pts',(61.9719008215855,-0.0386086908632389,
49.8893374284854));
#174022=CARTESIAN_POINT('Ctrl Pts',(61.9722723485771,-0.07721697300564,
49.890067325024));
#174023=CARTESIAN_POINT('Ctrl Pts',(61.9740902680162,-0.193059381531131,
49.8921128159878));
#174024=CARTESIAN_POINT('Ctrl Pts',(61.9762401391437,-0.270281536593981,
49.8932835767828));
#174025=CARTESIAN_POINT('Ctrl Pts',(61.9903399164194,-0.622718691519423,
49.8977695916096));
#174026=CARTESIAN_POINT('Ctrl Pts',(62.0132749459347,-0.897383461623408,
49.8988800511485));
#174027=CARTESIAN_POINT('Ctrl Pts',(62.1314503069768,-1.82461418207681,
49.8952281601475));
#174028=CARTESIAN_POINT('Ctrl Pts',(62.2825927448918,-2.46800064525378,
49.88026429198));
#174029=CARTESIAN_POINT('Ctrl Pts',(62.5446291335746,-3.22012079152954,
49.8496607753499));
#174030=CARTESIAN_POINT('Ctrl Pts',(62.5927555060374,-3.34910781432234,
49.8439163670925));
#174031=CARTESIAN_POINT('Ctrl Pts',(62.6799351968114,-3.56801770024668,
49.8333222087998));
#174032=CARTESIAN_POINT('Ctrl Pts',(62.7176037771392,-3.65847766312796,
49.8286919141738));
#174033=CARTESIAN_POINT('Ctrl Pts',(62.7984789875565,-3.84447399668024,
49.8186477774749));
#174034=CARTESIAN_POINT('Ctrl Pts',(62.8418829557966,-3.93990795901347,
49.813202487331));
#174035=CARTESIAN_POINT('Ctrl Pts',(62.9337938583576,-4.13336329246223,
49.8015641096309));
#174036=CARTESIAN_POINT('Ctrl Pts',(62.9824332342972,-4.23130270792171,
49.7953497651111));
#174037=CARTESIAN_POINT('Ctrl Pts',(63.3148528957183,-4.87238148852751,
49.7525174065633));
#174038=CARTESIAN_POINT('Ctrl Pts',(63.6491750771382,-5.38710153959971,
49.7078918497935));
#174039=CARTESIAN_POINT('Ctrl Pts',(64.0306847538311,-5.86505936749701,
49.6545838761671));
#174040=CARTESIAN_POINT('Ctrl Pts',(78.7320872163416,0.,37.9066414382813));
#174041=CARTESIAN_POINT('Ctrl Pts',(78.740769625225,2.41806680288088,37.9558818259319));
#174042=CARTESIAN_POINT('Ctrl Pts',(76.7871543254317,7.2349491628497,38.4018995743988));
#174043=CARTESIAN_POINT('Ctrl Pts',(69.6881675238581,10.2370276571518,39.8059564749922));
#174044=CARTESIAN_POINT('Ctrl Pts',(62.5891807222845,7.23494916284969,41.2100133755855));
#174045=CARTESIAN_POINT('Ctrl Pts',(59.6587577725946,1.77635683940025E-15,
41.8790399982859));
#174046=CARTESIAN_POINT('Ctrl Pts',(62.6412751755846,-7.2349491628497,41.5054557014892));
#174047=CARTESIAN_POINT('Ctrl Pts',(69.7923564304583,-10.2370276571518,
40.3968411267995));
#174048=CARTESIAN_POINT('Ctrl Pts',(76.9434376853319,-7.2349491628497,39.2882265521098));
#174049=CARTESIAN_POINT('Ctrl Pts',(79.9259550883219,-1.77635683940025E-15,
38.9146422553131));
#174050=CARTESIAN_POINT('Ctrl Pts',(76.995532138632,7.23494916284969,39.5836688780135));
#174051=CARTESIAN_POINT('Ctrl Pts',(69.8965453370584,10.2370276571518,40.9877257786068));
#174052=CARTESIAN_POINT('Ctrl Pts',(62.7975585354848,7.23494916284971,42.3917826792002));
#174053=CARTESIAN_POINT('Ctrl Pts',(59.8671355857949,3.5527136788005E-15,
43.0608093019006));
#174054=CARTESIAN_POINT('Ctrl Pts',(62.8496529887849,-7.23494916284971,
42.6872250051038));
#174055=CARTESIAN_POINT('Ctrl Pts',(70.0007342436585,-10.2370276571518,
41.5786104304142));
#174056=CARTESIAN_POINT('Ctrl Pts',(77.1518154985322,-7.23494916284971,
40.4699958557245));
#174057=CARTESIAN_POINT('Ctrl Pts',(80.1343329015222,-4.44089209850063E-15,
40.0964115589277));
#174058=CARTESIAN_POINT('Ctrl Pts',(77.2039099518322,7.2349491628497,40.7654381816281));
#174059=CARTESIAN_POINT('Ctrl Pts',(70.1049231502587,10.2370276571518,42.1694950822215));
#174060=CARTESIAN_POINT('Ctrl Pts',(63.0059363486851,7.23494916284972,43.5735519828148));
#174061=CARTESIAN_POINT('Ctrl Pts',(60.0755133989952,6.21724893790088E-15,
44.2425786055152));
#174062=CARTESIAN_POINT('Ctrl Pts',(63.0580308019852,-7.23494916284971,
43.8689943087185));
#174063=CARTESIAN_POINT('Ctrl Pts',(70.2091120568588,-10.2370276571518,
42.7603797340288));
#174064=CARTESIAN_POINT('Ctrl Pts',(77.3601933117325,-7.23494916284971,
41.6517651593391));
#174065=CARTESIAN_POINT('Ctrl Pts',(80.3427107147225,-7.99360577730113E-15,
41.2781808625424));
#174066=CARTESIAN_POINT('Ctrl Pts',(77.4122877650325,7.2349491628497,41.9472074852428));
#174067=CARTESIAN_POINT('Ctrl Pts',(70.3133009634589,10.2370276571518,43.3512643858361));
#174068=CARTESIAN_POINT('Ctrl Pts',(63.2143141618854,7.23494916284972,44.7553212864295));
#174069=CARTESIAN_POINT('Ctrl Pts',(60.2838912121955,9.76996261670138E-15,
45.4243479091299));
#174070=CARTESIAN_POINT('Ctrl Pts',(63.2664086151855,-7.23494916284971,
45.0507636123332));
#174071=CARTESIAN_POINT('Ctrl Pts',(70.4174898700591,-10.2370276571518,
43.9421490376435));
#174072=CARTESIAN_POINT('Ctrl Pts',(77.5685711249327,-7.23494916284971,
42.8335344629538));
#174073=CARTESIAN_POINT('Ctrl Pts',(80.5510885279228,-1.15463194561016E-14,
42.459950166157));
#174074=CARTESIAN_POINT('Ctrl Pts',(77.6206655782328,7.2349491628497,43.1289767888574));
#174075=CARTESIAN_POINT('Ctrl Pts',(70.5216787766592,10.2370276571518,44.5330336894508));
#174076=CARTESIAN_POINT('Ctrl Pts',(63.4226919750857,7.23494916284972,45.9370905900442));
#174077=CARTESIAN_POINT('Ctrl Pts',(60.4922690253957,1.15463194561016E-14,
46.6061172127446));
#174078=CARTESIAN_POINT('Ctrl Pts',(63.4747864283858,-7.2349491628497,46.2325329159478));
#174079=CARTESIAN_POINT('Ctrl Pts',(70.6258676832593,-10.2370276571518,
45.1239183412581));
#174080=CARTESIAN_POINT('Ctrl Pts',(77.776948938133,-7.23494916284971,44.0153037665684));
#174081=CARTESIAN_POINT('Ctrl Pts',(80.759466341123,0.,43.6417194697717));
#174082=CARTESIAN_POINT('Ctrl Pts',(77.8290433914331,7.23494916284965,44.3107460924721));
#174083=CARTESIAN_POINT('Ctrl Pts',(70.7300565898595,10.2370276571518,45.7148029930655));
#174084=CARTESIAN_POINT('Ctrl Pts',(63.631069788286,7.23494916284971,47.1188598936588));
#174085=CARTESIAN_POINT('Ctrl Pts',(60.700646838596,7.90478793533111E-14,
47.7878865163592));
#174086=CARTESIAN_POINT('Ctrl Pts',(63.683164241586,-7.23494916284972,47.4143022195625));
#174087=CARTESIAN_POINT('Ctrl Pts',(70.8342454964596,-10.2370276571518,
46.3056876448728));
#174088=CARTESIAN_POINT('Ctrl Pts',(77.9853267513333,-7.23494916284967,
45.1970730701831));
#174089=CARTESIAN_POINT('Ctrl Pts',(80.9678441543233,-1.59872115546023E-14,
44.8234887733864));
#174090=CARTESIAN_POINT('Ctrl Pts',(78.0374212046334,7.23494916284965,45.4925153960867));
#174091=CARTESIAN_POINT('Ctrl Pts',(70.9384344030598,10.2370276571518,46.8965722966801));
#174092=CARTESIAN_POINT('Ctrl Pts',(63.8394476014863,7.23494916284974,48.3006291972735));
#174093=CARTESIAN_POINT('Ctrl Pts',(60.9090246517963,-4.61852778244065E-14,
48.9696558199739));
#174094=CARTESIAN_POINT('Ctrl Pts',(63.8915420547863,-7.23494916284968,
48.5960715231771));
#174095=CARTESIAN_POINT('Ctrl Pts',(71.0426233096599,-10.2370276571518,
47.4874569484874));
#174096=CARTESIAN_POINT('Ctrl Pts',(78.1937045645336,-7.23494916284967,
46.3788423737977));
#174097=CARTESIAN_POINT('Ctrl Pts',(81.1762219675236,-2.04281036531029E-14,
46.005258077001));
#174098=CARTESIAN_POINT('Ctrl Pts',(78.2457990178337,7.23494916284965,46.6742846997014));
#174099=CARTESIAN_POINT('Ctrl Pts',(71.1468122162601,10.2370276571518,48.0783416002948));
#174100=CARTESIAN_POINT('Ctrl Pts',(64.0478254146866,7.23494916284971,49.4823985008881));
#174101=CARTESIAN_POINT('Ctrl Pts',(61.1174024649966,8.34887714518118E-14,
50.1514251235885));
#174102=CARTESIAN_POINT('Ctrl Pts',(64.0999198679866,-7.23494916284971,
49.7778408267918));
#174103=CARTESIAN_POINT('Ctrl Pts',(71.2510011228602,-10.2370276571518,
48.6692262521021));
#174104=CARTESIAN_POINT('Ctrl Pts',(77.6476023720424,-7.55168562811132,
47.6775768608315));
#174105=CARTESIAN_POINT('Ctrl Pts',(79.691478707762,-3.87217647526957,47.4026589808119));
#174106=CARTESIAN_POINT('Ctrl Pts',(80.1038958562351,-2.27117162724,47.3646400428343));
#174107=CARTESIAN_POINT('Ctrl Pts',(79.8990610925212,0.,38.2745868880941));
#174108=CARTESIAN_POINT('Ctrl Pts',(79.9077435014046,2.70221125641844,38.3238272757448));
#174109=CARTESIAN_POINT('Ctrl Pts',(77.7225204280915,8.08512033008161,38.810683723625));
#174110=CARTESIAN_POINT('Ctrl Pts',(69.7862784696405,11.4399698695112,40.3623712981132));
#174111=CARTESIAN_POINT('Ctrl Pts',(61.8500365111895,8.0851203300816,41.9140588726013));
#174112=CARTESIAN_POINT('Ctrl Pts',(58.5722019012198,1.77635683940025E-15,
42.6443435444217));
#174113=CARTESIAN_POINT('Ctrl Pts',(61.9021309644895,-8.08512033008161,
42.209501198505));
#174114=CARTESIAN_POINT('Ctrl Pts',(69.8904673762406,-11.4399698695112,
40.9532559499205));
#174115=CARTESIAN_POINT('Ctrl Pts',(77.8788037879917,-8.08512033008161,
39.697010701336));
#174116=CARTESIAN_POINT('Ctrl Pts',(81.2087328512614,-1.77635683940025E-15,
39.2621683554193));
#174117=CARTESIAN_POINT('Ctrl Pts',(77.9308982412917,8.0851203300816,39.9924530272397));
#174118=CARTESIAN_POINT('Ctrl Pts',(69.9946562828407,11.4399698695112,41.5441406017278));
#174119=CARTESIAN_POINT('Ctrl Pts',(62.0584143243898,8.08512033008162,43.095828176216));
#174120=CARTESIAN_POINT('Ctrl Pts',(58.7805797144201,3.5527136788005E-15,
43.8261128480364));
#174121=CARTESIAN_POINT('Ctrl Pts',(62.1105087776898,-8.08512033008161,
43.3912705021196));
#174122=CARTESIAN_POINT('Ctrl Pts',(70.0988451894409,-11.4399698695112,
42.1350252535352));
#174123=CARTESIAN_POINT('Ctrl Pts',(78.0871816011919,-8.08512033008162,
40.8787800049507));
#174124=CARTESIAN_POINT('Ctrl Pts',(81.4171106644617,-4.44089209850063E-15,
40.4439376590339));
#174125=CARTESIAN_POINT('Ctrl Pts',(78.139276054492,8.08512033008161,41.1742223308544));
#174126=CARTESIAN_POINT('Ctrl Pts',(70.203034096041,11.4399698695112,42.7259099053425));
#174127=CARTESIAN_POINT('Ctrl Pts',(62.2667921375901,8.08512033008162,44.2775974798306));
#174128=CARTESIAN_POINT('Ctrl Pts',(58.9889575276203,6.21724893790088E-15,
45.007882151651));
#174129=CARTESIAN_POINT('Ctrl Pts',(62.3188865908901,-8.08512033008161,
44.5730398057343));
#174130=CARTESIAN_POINT('Ctrl Pts',(70.3072230026411,-11.4399698695112,
43.3167945571498));
#174131=CARTESIAN_POINT('Ctrl Pts',(78.2955594143922,-8.08512033008162,
42.0605493085653));
#174132=CARTESIAN_POINT('Ctrl Pts',(81.625488477662,-7.99360577730113E-15,
41.6257069626486));
#174133=CARTESIAN_POINT('Ctrl Pts',(78.3476538676923,8.08512033008161,42.355991634469));
#174134=CARTESIAN_POINT('Ctrl Pts',(70.4114119092413,11.4399698695112,43.9076792089571));
#174135=CARTESIAN_POINT('Ctrl Pts',(62.4751699507903,8.08512033008163,45.4593667834453));
#174136=CARTESIAN_POINT('Ctrl Pts',(59.1973353408206,9.76996261670138E-15,
46.1896514552657));
#174137=CARTESIAN_POINT('Ctrl Pts',(62.5272644040904,-8.08512033008161,
45.7548091093489));
#174138=CARTESIAN_POINT('Ctrl Pts',(70.5156008158414,-11.4399698695112,
44.4985638607645));
#174139=CARTESIAN_POINT('Ctrl Pts',(78.5039372275925,-8.08512033008162,
43.24231861218));
#174140=CARTESIAN_POINT('Ctrl Pts',(81.8338662908623,-1.15463194561016E-14,
42.8074762662632));
#174141=CARTESIAN_POINT('Ctrl Pts',(78.5560316808926,8.08512033008161,43.5377609380837));
#174142=CARTESIAN_POINT('Ctrl Pts',(70.6197897224416,11.4399698695112,45.0894485125718));
#174143=CARTESIAN_POINT('Ctrl Pts',(62.6835477639906,8.08512033008163,46.6411360870599));
#174144=CARTESIAN_POINT('Ctrl Pts',(59.4057131540209,1.15463194561016E-14,
47.3714207588804));
#174145=CARTESIAN_POINT('Ctrl Pts',(62.7356422172907,-8.08512033008161,
46.9365784129636));
#174146=CARTESIAN_POINT('Ctrl Pts',(70.7239786290417,-11.4399698695112,
45.6803331643791));
#174147=CARTESIAN_POINT('Ctrl Pts',(78.7123150407928,-8.08512033008162,
44.4240879157947));
#174148=CARTESIAN_POINT('Ctrl Pts',(82.0422441040625,0.,43.9892455698779));
#174149=CARTESIAN_POINT('Ctrl Pts',(78.7644094940929,8.08512033008155,44.7195302416983));
#174150=CARTESIAN_POINT('Ctrl Pts',(70.8281675356419,11.4399698695112,46.2712178161865));
#174151=CARTESIAN_POINT('Ctrl Pts',(62.8919255771909,8.08512033008161,47.8229053906746));
#174152=CARTESIAN_POINT('Ctrl Pts',(59.6140909672212,7.90478793533111E-14,
48.553190062495));
#174153=CARTESIAN_POINT('Ctrl Pts',(62.944020030491,-8.08512033008163,48.1183477165782));
#174154=CARTESIAN_POINT('Ctrl Pts',(70.932356442242,-11.4399698695112,46.8621024679938));
#174155=CARTESIAN_POINT('Ctrl Pts',(78.9206928539931,-8.08512033008157,
45.6058572194093));
#174156=CARTESIAN_POINT('Ctrl Pts',(82.2506219172628,-1.59872115546023E-14,
45.1710148734926));
#174157=CARTESIAN_POINT('Ctrl Pts',(78.9727873072932,8.08512033008155,45.901299545313));
#174158=CARTESIAN_POINT('Ctrl Pts',(71.0365453488421,11.4399698695112,47.4529871198011));
#174159=CARTESIAN_POINT('Ctrl Pts',(63.1003033903912,8.08512033008165,49.0046746942892));
#174160=CARTESIAN_POINT('Ctrl Pts',(59.8224687804215,-4.61852778244065E-14,
49.7349593661097));
#174161=CARTESIAN_POINT('Ctrl Pts',(63.1523978436912,-8.08512033008159,
49.3001170201929));
#174162=CARTESIAN_POINT('Ctrl Pts',(71.1407342554422,-11.4399698695112,
48.0438717716084));
#174163=CARTESIAN_POINT('Ctrl Pts',(79.1290706671934,-8.08512033008157,
46.787626523024));
#174164=CARTESIAN_POINT('Ctrl Pts',(82.4589997304631,-2.04281036531029E-14,
46.3527841771072));
#174165=CARTESIAN_POINT('Ctrl Pts',(79.1811651204935,8.08512033008155,47.0830688489276));
#174166=CARTESIAN_POINT('Ctrl Pts',(71.2449231620424,11.4399698695112,48.6347564234158));
#174167=CARTESIAN_POINT('Ctrl Pts',(63.3086812035915,8.08512033008162,50.1864439979039));
#174168=CARTESIAN_POINT('Ctrl Pts',(60.0308465936217,8.34887714518118E-14,
50.9167286697243));
#174169=CARTESIAN_POINT('Ctrl Pts',(63.3607756568915,-8.08512033008162,
50.4818863238076));
#174170=CARTESIAN_POINT('Ctrl Pts',(71.3491120686425,-11.4399698695112,
49.2256410752231));
#174171=CARTESIAN_POINT('Ctrl Pts',(78.4946332631429,-8.43907615989096,
48.1019368912023));
#174172=CARTESIAN_POINT('Ctrl Pts',(80.7769657380788,-4.32719180704438,
47.7849727601233));
#174173=CARTESIAN_POINT('Ctrl Pts',(81.2371482556239,-2.53805458520595,
47.7385314988347));
#174174=CARTESIAN_POINT('Ctrl Pts',(79.6939233571059,0.,37.1111929787152));
#174175=CARTESIAN_POINT('Ctrl Pts',(79.7026057659892,2.70221125641844,37.1604333663658));
#174176=CARTESIAN_POINT('Ctrl Pts',(77.5173826926761,8.08512033008161,37.6472898142461));
#174177=CARTESIAN_POINT('Ctrl Pts',(69.5811407342251,11.4399698695112,39.1989773887342));
#174178=CARTESIAN_POINT('Ctrl Pts',(61.6448987757741,8.0851203300816,40.7506649632223));
#174179=CARTESIAN_POINT('Ctrl Pts',(58.3670641658044,1.77635683940025E-15,
41.4809496350428));
#174180=CARTESIAN_POINT('Ctrl Pts',(61.6969932290742,-8.08512033008161,
41.046107289126));
#174181=CARTESIAN_POINT('Ctrl Pts',(69.6853296408252,-11.4399698695112,
39.7898620405415));
#174182=CARTESIAN_POINT('Ctrl Pts',(77.6736660525763,-8.08512033008161,
38.5336167919571));
#174183=CARTESIAN_POINT('Ctrl Pts',(81.0035951158461,-1.77635683940025E-15,
38.0987744460403));
#174184=CARTESIAN_POINT('Ctrl Pts',(77.7257605058764,8.0851203300816,38.8290591178608));
#174185=CARTESIAN_POINT('Ctrl Pts',(69.7895185474254,11.4399698695112,40.3807466923489));
#174186=CARTESIAN_POINT('Ctrl Pts',(61.8532765889744,8.08512033008162,41.932434266837));
#174187=CARTESIAN_POINT('Ctrl Pts',(58.5754419790047,3.5527136788005E-15,
42.6627189386574));
#174188=CARTESIAN_POINT('Ctrl Pts',(61.9053710422745,-8.08512033008161,
42.2278765927407));
#174189=CARTESIAN_POINT('Ctrl Pts',(69.8937074540255,-11.4399698695112,
40.9716313441562));
#174190=CARTESIAN_POINT('Ctrl Pts',(77.8820438657766,-8.08512033008162,
39.7153860955717));
#174191=CARTESIAN_POINT('Ctrl Pts',(81.2119729290464,-4.44089209850063E-15,
39.280543749655));
#174192=CARTESIAN_POINT('Ctrl Pts',(77.9341383190766,8.08512033008161,40.0108284214754));
#174193=CARTESIAN_POINT('Ctrl Pts',(69.9978963606257,11.4399698695112,41.5625159959635));
#174194=CARTESIAN_POINT('Ctrl Pts',(62.0616544021747,8.08512033008162,43.1142035704517));
#174195=CARTESIAN_POINT('Ctrl Pts',(58.783819792205,6.21724893790088E-15,
43.8444882422721));
#174196=CARTESIAN_POINT('Ctrl Pts',(62.1137488554748,-8.08512033008161,
43.4096458963553));
#174197=CARTESIAN_POINT('Ctrl Pts',(70.1020852672257,-11.4399698695112,
42.1534006477709));
#174198=CARTESIAN_POINT('Ctrl Pts',(78.0904216789768,-8.08512033008162,
40.8971553991864));
#174199=CARTESIAN_POINT('Ctrl Pts',(81.4203507422466,-7.99360577730113E-15,
40.4623130532696));
#174200=CARTESIAN_POINT('Ctrl Pts',(78.1425161322769,8.08512033008161,41.1925977250901));
#174201=CARTESIAN_POINT('Ctrl Pts',(70.2062741738259,11.4399698695112,42.7442852995782));
#174202=CARTESIAN_POINT('Ctrl Pts',(62.270032215375,8.08512033008163,44.2959728740663));
#174203=CARTESIAN_POINT('Ctrl Pts',(58.9921976054052,9.76996261670138E-15,
45.0262575458867));
#174204=CARTESIAN_POINT('Ctrl Pts',(62.322126668675,-8.08512033008161,44.59141519997));
#174205=CARTESIAN_POINT('Ctrl Pts',(70.310463080426,-11.4399698695112,43.3351699513855));
#174206=CARTESIAN_POINT('Ctrl Pts',(78.2987994921771,-8.08512033008162,
42.0789247028011));
#174207=CARTESIAN_POINT('Ctrl Pts',(81.6287285554469,-1.15463194561016E-14,
41.6440823568843));
#174208=CARTESIAN_POINT('Ctrl Pts',(78.3508939454772,8.08512033008161,42.3743670287047));
#174209=CARTESIAN_POINT('Ctrl Pts',(70.4146519870262,11.4399698695112,43.9260546031928));
#174210=CARTESIAN_POINT('Ctrl Pts',(62.4784100285753,8.08512033008163,45.477742177681));
#174211=CARTESIAN_POINT('Ctrl Pts',(59.2005754186055,1.15463194561016E-14,
46.2080268495014));
#174212=CARTESIAN_POINT('Ctrl Pts',(62.5305044818753,-8.08512033008161,
45.7731845035846));
#174213=CARTESIAN_POINT('Ctrl Pts',(70.5188408936263,-11.4399698695112,
44.5169392550002));
#174214=CARTESIAN_POINT('Ctrl Pts',(78.5071773053774,-8.08512033008162,
43.2606940064157));
#174215=CARTESIAN_POINT('Ctrl Pts',(81.8371063686472,0.,42.8258516604989));
#174216=CARTESIAN_POINT('Ctrl Pts',(78.5592717586776,8.08512033008155,43.5561363323194));
#174217=CARTESIAN_POINT('Ctrl Pts',(70.6230298002265,11.4399698695112,45.1078239068075));
#174218=CARTESIAN_POINT('Ctrl Pts',(62.6867878417755,8.08512033008161,46.6595114812956));
#174219=CARTESIAN_POINT('Ctrl Pts',(59.4089532318058,7.90478793533111E-14,
47.3897961531161));
#174220=CARTESIAN_POINT('Ctrl Pts',(62.7388822950756,-8.08512033008163,
46.9549538071993));
#174221=CARTESIAN_POINT('Ctrl Pts',(70.7272187068266,-11.4399698695112,
45.6987085586148));
#174222=CARTESIAN_POINT('Ctrl Pts',(78.7155551185777,-8.08512033008157,
44.4424633100304));
#174223=CARTESIAN_POINT('Ctrl Pts',(82.0454841818474,-1.59872115546023E-14,
44.0076209641136));
#174224=CARTESIAN_POINT('Ctrl Pts',(78.7676495718778,8.08512033008155,44.737905635934));
#174225=CARTESIAN_POINT('Ctrl Pts',(70.8314076134267,11.4399698695112,46.2895932104222));
#174226=CARTESIAN_POINT('Ctrl Pts',(62.8951656549758,8.08512033008165,47.8412807849103));
#174227=CARTESIAN_POINT('Ctrl Pts',(59.6173310450061,-4.61852778244065E-14,
48.5715654567307));
#174228=CARTESIAN_POINT('Ctrl Pts',(62.9472601082759,-8.08512033008159,
48.1367231108139));
#174229=CARTESIAN_POINT('Ctrl Pts',(70.9355965200269,-11.4399698695112,
46.8804778622295));
#174230=CARTESIAN_POINT('Ctrl Pts',(78.923932931778,-8.08512033008157,45.624232613645));
#174231=CARTESIAN_POINT('Ctrl Pts',(82.2538619950477,-2.04281036531029E-14,
45.1893902677283));
#174232=CARTESIAN_POINT('Ctrl Pts',(78.9760273850781,8.08512033008155,45.9196749395487));
#174233=CARTESIAN_POINT('Ctrl Pts',(71.039785426627,11.4399698695112,47.4713625140368));
#174234=CARTESIAN_POINT('Ctrl Pts',(63.1035434681761,8.08512033008162,49.0230500885249));
#174235=CARTESIAN_POINT('Ctrl Pts',(59.8257088582064,8.34887714518118E-14,
49.7533347603454));
#174236=CARTESIAN_POINT('Ctrl Pts',(63.1556379214762,-8.08512033008162,
49.3184924144286));
#174237=CARTESIAN_POINT('Ctrl Pts',(71.1439743332271,-11.4399698695112,
48.0622471658441));
#174238=CARTESIAN_POINT('Ctrl Pts',(78.2894955277276,-8.43907615989096,
46.9385429818233));
#174239=CARTESIAN_POINT('Ctrl Pts',(80.5718280026635,-4.32719180704438,
46.6215788507443));
#174240=CARTESIAN_POINT('Ctrl Pts',(81.0320105202085,-2.53805458520595,
46.5751375894558));
#174241=CARTESIAN_POINT('Ctrl Pts',(78.7231713724909,0.,37.8560771751443));
#174242=CARTESIAN_POINT('Ctrl Pts',(78.7318537813743,2.41806680288088,37.9053175627949));
#174243=CARTESIAN_POINT('Ctrl Pts',(76.778238481581,7.2349491628497,38.3513353112619));
#174244=CARTESIAN_POINT('Ctrl Pts',(69.6792516800074,10.2370276571518,39.7553922118552));
#174245=CARTESIAN_POINT('Ctrl Pts',(62.5802648784339,7.23494916284969,41.1594491124486));
#174246=CARTESIAN_POINT('Ctrl Pts',(59.6498419287439,1.77635683940025E-15,
41.828475735149));
#174247=CARTESIAN_POINT('Ctrl Pts',(62.6323593317339,-7.2349491628497,41.4548914383522));
#174248=CARTESIAN_POINT('Ctrl Pts',(69.7834405866076,-10.2370276571518,
40.3462768636625));
#174249=CARTESIAN_POINT('Ctrl Pts',(76.9345218414812,-7.2349491628497,39.2376622889728));
#174250=CARTESIAN_POINT('Ctrl Pts',(79.9170392444712,-1.77635683940025E-15,
38.8640779921761));
#174251=CARTESIAN_POINT('Ctrl Pts',(76.9866162947813,7.23494916284969,39.5331046148765));
#174252=CARTESIAN_POINT('Ctrl Pts',(69.8876294932077,10.2370276571518,40.9371615154699));
#174253=CARTESIAN_POINT('Ctrl Pts',(62.7886426916342,7.23494916284971,42.3412184160632));
#174254=CARTESIAN_POINT('Ctrl Pts',(59.8582197419442,3.5527136788005E-15,
43.0102450387636));
#174255=CARTESIAN_POINT('Ctrl Pts',(62.8407371449342,-7.23494916284971,
42.6366607419669));
#174256=CARTESIAN_POINT('Ctrl Pts',(69.9918183998079,-10.2370276571518,
41.5280461672772));
#174257=CARTESIAN_POINT('Ctrl Pts',(77.1428996546815,-7.23494916284971,
40.4194315925875));
#174258=CARTESIAN_POINT('Ctrl Pts',(80.1254170576715,-4.44089209850063E-15,
40.0458472957908));
#174259=CARTESIAN_POINT('Ctrl Pts',(77.1949941079816,7.2349491628497,40.7148739184912));
#174260=CARTESIAN_POINT('Ctrl Pts',(70.096007306408,10.2370276571518,42.1189308190845));
#174261=CARTESIAN_POINT('Ctrl Pts',(62.9970205048345,7.23494916284972,43.5229877196779));
#174262=CARTESIAN_POINT('Ctrl Pts',(60.0665975551445,6.21724893790088E-15,
44.1920143423783));
#174263=CARTESIAN_POINT('Ctrl Pts',(63.0491149581345,-7.23494916284971,
43.8184300455816));
#174264=CARTESIAN_POINT('Ctrl Pts',(70.2001962130081,-10.2370276571518,
42.7098154708919));
#174265=CARTESIAN_POINT('Ctrl Pts',(77.3512774678818,-7.23494916284971,
41.6012008962022));
#174266=CARTESIAN_POINT('Ctrl Pts',(80.3337948708718,-7.99360577730113E-15,
41.2276165994054));
#174267=CARTESIAN_POINT('Ctrl Pts',(77.4033719211819,7.2349491628497,41.8966432221058));
#174268=CARTESIAN_POINT('Ctrl Pts',(70.3043851196083,10.2370276571518,43.3007001226992));
#174269=CARTESIAN_POINT('Ctrl Pts',(63.2053983180347,7.23494916284972,44.7047570232925));
#174270=CARTESIAN_POINT('Ctrl Pts',(60.2749753683448,9.76996261670138E-15,
45.3737836459929));
#174271=CARTESIAN_POINT('Ctrl Pts',(63.2574927713348,-7.23494916284971,
45.0001993491962));
#174272=CARTESIAN_POINT('Ctrl Pts',(70.4085740262084,-10.2370276571518,
43.8915847745065));
#174273=CARTESIAN_POINT('Ctrl Pts',(77.5596552810821,-7.23494916284971,
42.7829701998168));
#174274=CARTESIAN_POINT('Ctrl Pts',(80.5421726840721,-1.15463194561016E-14,
42.4093859030201));
#174275=CARTESIAN_POINT('Ctrl Pts',(77.6117497343821,7.2349491628497,43.0784125257205));
#174276=CARTESIAN_POINT('Ctrl Pts',(70.5127629328085,10.2370276571518,44.4824694263138));
#174277=CARTESIAN_POINT('Ctrl Pts',(63.413776131235,7.23494916284972,45.8865263269072));
#174278=CARTESIAN_POINT('Ctrl Pts',(60.483353181545,1.15463194561016E-14,
46.5555529496076));
#174279=CARTESIAN_POINT('Ctrl Pts',(63.4658705845351,-7.2349491628497,46.1819686528109));
#174280=CARTESIAN_POINT('Ctrl Pts',(70.6169518394087,-10.2370276571518,
45.0733540781212));
#174281=CARTESIAN_POINT('Ctrl Pts',(77.7680330942823,-7.23494916284971,
43.9647395034315));
#174282=CARTESIAN_POINT('Ctrl Pts',(80.7505504972723,0.,43.5911552066347));
#174283=CARTESIAN_POINT('Ctrl Pts',(77.8201275475825,7.23494916284965,44.2601818293351));
#174284=CARTESIAN_POINT('Ctrl Pts',(70.7211407460088,10.2370276571518,45.6642387299285));
#174285=CARTESIAN_POINT('Ctrl Pts',(63.6221539444353,7.23494916284971,47.0682956305219));
#174286=CARTESIAN_POINT('Ctrl Pts',(60.6917309947453,7.90478793533111E-14,
47.7373222532223));
#174287=CARTESIAN_POINT('Ctrl Pts',(63.6742483977354,-7.23494916284972,
47.3637379564255));
#174288=CARTESIAN_POINT('Ctrl Pts',(70.8253296526089,-10.2370276571518,
46.2551233817358));
#174289=CARTESIAN_POINT('Ctrl Pts',(77.9764109074827,-7.23494916284967,
45.1465088070461));
#174290=CARTESIAN_POINT('Ctrl Pts',(80.9589283104726,-1.59872115546023E-14,
44.7729245102494));
#174291=CARTESIAN_POINT('Ctrl Pts',(78.0285053607827,7.23494916284965,45.4419511329498));
#174292=CARTESIAN_POINT('Ctrl Pts',(70.9295185592091,10.2370276571518,46.8460080335432));
#174293=CARTESIAN_POINT('Ctrl Pts',(63.8305317576356,7.23494916284974,48.2500649341365));
#174294=CARTESIAN_POINT('Ctrl Pts',(60.9001088079456,-4.61852778244065E-14,
48.9190915568369));
#174295=CARTESIAN_POINT('Ctrl Pts',(63.8826262109356,-7.23494916284968,
48.5455072600402));
#174296=CARTESIAN_POINT('Ctrl Pts',(71.0337074658092,-10.2370276571518,
47.4368926853505));
#174297=CARTESIAN_POINT('Ctrl Pts',(78.1847887206829,-7.23494916284967,
46.3282781106608));
#174298=CARTESIAN_POINT('Ctrl Pts',(81.1673061236729,-2.04281036531029E-14,
45.9546938138641));
#174299=CARTESIAN_POINT('Ctrl Pts',(78.236883173983,7.23494916284965,46.6237204365644));
#174300=CARTESIAN_POINT('Ctrl Pts',(71.1378963724094,10.2370276571518,48.0277773371578));
#174301=CARTESIAN_POINT('Ctrl Pts',(64.0389095708359,7.23494916284971,49.4318342377512));
#174302=CARTESIAN_POINT('Ctrl Pts',(61.1084866211459,8.34887714518118E-14,
50.1008608604516));
#174303=CARTESIAN_POINT('Ctrl Pts',(64.0910040241359,-7.23494916284971,
49.7272765636548));
#174304=CARTESIAN_POINT('Ctrl Pts',(71.2420852790095,-10.2370276571518,
48.6186619889651));
#174305=CARTESIAN_POINT('Ctrl Pts',(77.6386865281917,-7.55168562811132,
47.6270125976946));
#174306=CARTESIAN_POINT('Ctrl Pts',(79.6825628639114,-3.87217647526957,
47.352094717675));
#174307=CARTESIAN_POINT('Ctrl Pts',(80.0949800123844,-2.27117162724,47.3140757796973));
#174308=CARTESIAN_POINT('Ctrl Pts',(82.4182377853508,-4.33680868994202E-16,
57.4564977112756));
#174309=CARTESIAN_POINT('Ctrl Pts',(82.4135348138723,-2.47968200709192,
57.4298258346316));
#174310=CARTESIAN_POINT('Ctrl Pts',(80.3829258470673,-7.41930423095383,
57.7328747079373));
#174311=CARTESIAN_POINT('Ctrl Pts',(73.0622286040322,-10.4978792386127,
58.9412077372665));
#174312=CARTESIAN_POINT('Ctrl Pts',(65.7415313609972,-7.41930423095383,
60.1495407665957));
#174313=CARTESIAN_POINT('Ctrl Pts',(62.6956179107897,-2.21003770839445E-15,
60.6041140765543));
#174314=CARTESIAN_POINT('Ctrl Pts',(65.7133135321263,7.41930423095382,59.9895095067313));
#174315=CARTESIAN_POINT('Ctrl Pts',(73.0057929462905,10.4978792386127,58.6211452175376));
#174316=CARTESIAN_POINT('Ctrl Pts',(80.2982723604547,7.41930423095383,57.2527809283438));
#174317=CARTESIAN_POINT('Ctrl Pts',(83.3159679817913,1.78676518025611E-15,
56.6381763585208));
#174318=CARTESIAN_POINT('Ctrl Pts',(80.2700545315838,-7.41930423095382,
57.0927496684794));
#174319=CARTESIAN_POINT('Ctrl Pts',(72.9493572885488,-10.4978792386127,
58.3010826978086));
#174320=CARTESIAN_POINT('Ctrl Pts',(65.6286600455137,-7.41930423095384,
59.5094157271378));
#174321=CARTESIAN_POINT('Ctrl Pts',(62.5827465953062,-3.54230533794464E-15,
59.9639890370964));
#174322=CARTESIAN_POINT('Ctrl Pts',(65.6004422166428,7.41930423095383,59.3493844672733));
#174323=CARTESIAN_POINT('Ctrl Pts',(72.892921630807,10.4978792386127,57.9810201780796));
#174324=CARTESIAN_POINT('Ctrl Pts',(80.1854010449712,7.41930423095384,56.6126558888859));
#174325=CARTESIAN_POINT('Ctrl Pts',(83.2030966663078,5.33947885905661E-15,
55.9980513190628));
#174326=CARTESIAN_POINT('Ctrl Pts',(80.1571832161003,-7.41930423095383,
56.4526246290214));
#174327=CARTESIAN_POINT('Ctrl Pts',(72.8364859730653,-10.4978792386127,
57.6609576583506));
#174328=CARTESIAN_POINT('Ctrl Pts',(65.5157887300302,-7.41930423095384,
58.8692906876799));
#174329=CARTESIAN_POINT('Ctrl Pts',(62.4698752798227,-7.5391082265952E-15,
59.3238639976385));
#174330=CARTESIAN_POINT('Ctrl Pts',(65.4875709011593,7.41930423095383,58.7092594278154));
#174331=CARTESIAN_POINT('Ctrl Pts',(72.7800503153235,10.4978792386127,57.3408951386217));
#174332=CARTESIAN_POINT('Ctrl Pts',(80.0725297294877,7.41930423095384,55.972530849428));
#174333=CARTESIAN_POINT('Ctrl Pts',(83.0902253508243,7.11583569845686E-15,
55.3579262796049));
#174334=CARTESIAN_POINT('Ctrl Pts',(80.0443119006168,-7.41930423095383,
55.8124995895635));
#174335=CARTESIAN_POINT('Ctrl Pts',(72.7236146575817,-10.4978792386127,
57.0208326188927));
#174336=CARTESIAN_POINT('Ctrl Pts',(65.4029174145467,-7.41930423095385,
58.2291656482219));
#174337=CARTESIAN_POINT('Ctrl Pts',(62.3570039643392,-9.31546506599545E-15,
58.6837389581805));
#174338=CARTESIAN_POINT('Ctrl Pts',(65.3746995856758,7.41930423095384,58.0691343883574));
#174339=CARTESIAN_POINT('Ctrl Pts',(72.66717899984,10.4978792386127,56.7007700991637));
#174340=CARTESIAN_POINT('Ctrl Pts',(79.9596584140042,7.41930423095385,55.33240580997));
#174341=CARTESIAN_POINT('Ctrl Pts',(82.9773540353409,9.33628174770718E-15,
54.717801240147));
#174342=CARTESIAN_POINT('Ctrl Pts',(79.9314405851334,-7.41930423095383,
55.1723745501055));
#174343=CARTESIAN_POINT('Ctrl Pts',(72.6107433420983,-10.4978792386127,
56.3807075794348));
#174344=CARTESIAN_POINT('Ctrl Pts',(65.2900460990632,-7.41930423095385,
57.589040608764));
#174345=CARTESIAN_POINT('Ctrl Pts',(62.2441326488557,-1.24240895349459E-14,
58.0436139187226));
#174346=CARTESIAN_POINT('Ctrl Pts',(65.2618282701924,7.41930423095383,57.4290093488995));
#174347=CARTESIAN_POINT('Ctrl Pts',(72.5543076843565,10.4978792386127,56.0606450597058));
#174348=CARTESIAN_POINT('Ctrl Pts',(79.8467870985207,7.41930423095385,54.6922807705121));
#174349=CARTESIAN_POINT('Ctrl Pts',(82.8644827198574,1.04083408558608E-17,
54.077676200689));
#174350=CARTESIAN_POINT('Ctrl Pts',(79.8185692696499,-7.41930423095378,
54.5322495106476));
#174351=CARTESIAN_POINT('Ctrl Pts',(72.4978720266148,-10.4978792386127,
55.7405825399768));
#174352=CARTESIAN_POINT('Ctrl Pts',(65.1771747835797,-7.41930423095383,
56.9489155693061));
#174353=CARTESIAN_POINT('Ctrl Pts',(62.1312613333722,-7.81492925927552E-14,
57.4034888792646));
#174354=CARTESIAN_POINT('Ctrl Pts',(65.1489569547089,7.41930423095385,56.7888843094416));
#174355=CARTESIAN_POINT('Ctrl Pts',(72.441436368873,10.4978792386127,55.4205200202479));
#174356=CARTESIAN_POINT('Ctrl Pts',(79.7339157830373,7.4193042309538,54.0521557310541));
#174357=CARTESIAN_POINT('Ctrl Pts',(82.7516114043739,1.5109441475758E-14,
53.4375511612311));
#174358=CARTESIAN_POINT('Ctrl Pts',(79.7056979541665,-7.41930423095378,
53.8921244711896));
#174359=CARTESIAN_POINT('Ctrl Pts',(72.3850007111313,-10.4978792386127,
55.1004575005189));
#174360=CARTESIAN_POINT('Ctrl Pts',(65.0643034680963,-7.41930423095387,
56.3087905298481));
#174361=CARTESIAN_POINT('Ctrl Pts',(62.0183900178887,4.44193293258621E-14,
56.7633638398067));
#174362=CARTESIAN_POINT('Ctrl Pts',(65.0360856392254,7.41930423095381,56.1487592699836));
#174363=CARTESIAN_POINT('Ctrl Pts',(72.3285650533895,10.4978792386127,54.7803949807899));
#174364=CARTESIAN_POINT('Ctrl Pts',(79.6210444675538,7.4193042309538,53.4120306915962));
#174365=CARTESIAN_POINT('Ctrl Pts',(82.6387400888904,1.77739767348584E-14,
52.7974261217731));
#174366=CARTESIAN_POINT('Ctrl Pts',(79.592826638683,-7.41930423095377,53.2519994317317));
#174367=CARTESIAN_POINT('Ctrl Pts',(72.2721293956478,-10.4978792386127,
54.460332461061));
#174368=CARTESIAN_POINT('Ctrl Pts',(64.9514321526128,-7.41930423095384,
55.6686654903902));
#174369=CARTESIAN_POINT('Ctrl Pts',(61.9055187024052,-8.21460954814057E-14,
56.1232388003488));
#174370=CARTESIAN_POINT('Ctrl Pts',(64.9232143237419,7.41930423095385,55.5086342305257));
#174371=CARTESIAN_POINT('Ctrl Pts',(72.215693737906,10.4978792386127,54.140269941332));
#174372=CARTESIAN_POINT('Ctrl Pts',(79.5081731520703,7.41930423095381,52.7719056521383));
#174373=CARTESIAN_POINT('Ctrl Pts',(82.5258687734069,2.04385119939587E-14,
52.1573010823152));
#174374=CARTESIAN_POINT('Ctrl Pts',(79.4799553231995,-7.41930423095377,
52.6118743922738));
#174375=CARTESIAN_POINT('Ctrl Pts',(72.1592580801643,-10.4978792386127,
53.820207421603));
#174376=CARTESIAN_POINT('Ctrl Pts',(64.8385608371293,-7.41930423095387,
55.0285404509322));
#174377=CARTESIAN_POINT('Ctrl Pts',(61.7926473869218,3.95343480175114E-14,
55.4831137608908));
#174378=CARTESIAN_POINT('Ctrl Pts',(64.8103430082584,7.41930423095381,54.8685091910678));
#174379=CARTESIAN_POINT('Ctrl Pts',(72.1028224224225,10.4978792386127,53.5001449018741));
#174380=CARTESIAN_POINT('Ctrl Pts',(79.3953018365868,7.4193042309538,52.1317806126803));
#174381=CARTESIAN_POINT('Ctrl Pts',(82.4129974579234,2.39912256727592E-14,
51.5171760428573));
#174382=CARTESIAN_POINT('Ctrl Pts',(79.4795767970927,-7.14529177399519,
51.9549608851035));
#174383=CARTESIAN_POINT('Ctrl Pts',(75.0186143089714,-9.23540832385942,
52.6895937030669));
#174384=CARTESIAN_POINT('Ctrl Pts',(72.8565297133897,-9.43430675859939,
53.0463734606267));
#174385=CARTESIAN_POINT('Ctrl Pts',(82.9022195620938,-4.33680868994202E-16,
57.0503887809141));
#174386=CARTESIAN_POINT('Ctrl Pts',(82.8975165906153,-2.62292530172754,
57.02371690427));
#174387=CARTESIAN_POINT('Ctrl Pts',(80.7501491929166,-7.84789369480698,
57.3473534391675));
#174388=CARTESIAN_POINT('Ctrl Pts',(73.0073737230196,-11.1043081293031,
58.630110247862));
#174389=CARTESIAN_POINT('Ctrl Pts',(65.2645982531226,-7.84789369480698,
59.9128670565566));
#174390=CARTESIAN_POINT('Ctrl Pts',(62.0435471565745,-2.21003770839445E-15,
60.3983218589028));
#174391=CARTESIAN_POINT('Ctrl Pts',(65.2363804242517,7.84789369480698,59.7528357966921));
#174392=CARTESIAN_POINT('Ctrl Pts',(72.9509380652778,11.1043081293031,58.3100477281331));
#174393=CARTESIAN_POINT('Ctrl Pts',(80.665495706304,7.84789369480698,56.867259659574));
#174394=CARTESIAN_POINT('Ctrl Pts',(83.8583289739812,1.78676518025611E-15,
56.2217735973633));
#174395=CARTESIAN_POINT('Ctrl Pts',(80.6372778774331,-7.84789369480698,
56.7072283997095));
#174396=CARTESIAN_POINT('Ctrl Pts',(72.8945024075361,-11.1043081293031,
57.9899852084041));
#174397=CARTESIAN_POINT('Ctrl Pts',(65.1517269376391,-7.847893694807,59.2727420170987));
#174398=CARTESIAN_POINT('Ctrl Pts',(61.930675841091,-3.54230533794464E-15,
59.7581968194449));
#174399=CARTESIAN_POINT('Ctrl Pts',(65.1235091087682,7.84789369480699,59.1127107572342));
#174400=CARTESIAN_POINT('Ctrl Pts',(72.8380667497943,11.1043081293031,57.6699226886751));
#174401=CARTESIAN_POINT('Ctrl Pts',(80.5526243908205,7.847893694807,56.2271346201161));
#174402=CARTESIAN_POINT('Ctrl Pts',(83.7454576584977,5.33947885905661E-15,
55.5816485579054));
#174403=CARTESIAN_POINT('Ctrl Pts',(80.5244065619496,-7.84789369480699,
56.0671033602516));
#174404=CARTESIAN_POINT('Ctrl Pts',(72.7816310920526,-11.1043081293031,
57.3498601689462));
#174405=CARTESIAN_POINT('Ctrl Pts',(65.0388556221556,-7.847893694807,58.6326169776407));
#174406=CARTESIAN_POINT('Ctrl Pts',(61.8178045256075,-7.5391082265952E-15,
59.1180717799869));
#174407=CARTESIAN_POINT('Ctrl Pts',(65.0106377932847,7.84789369480699,58.4725857177762));
#174408=CARTESIAN_POINT('Ctrl Pts',(72.7251954343108,11.1043081293031,57.0297976492172));
#174409=CARTESIAN_POINT('Ctrl Pts',(80.439753075337,7.84789369480699,55.5870095806582));
#174410=CARTESIAN_POINT('Ctrl Pts',(83.6325863430142,7.11583569845686E-15,
54.9415235184475));
#174411=CARTESIAN_POINT('Ctrl Pts',(80.4115352464661,-7.84789369480698,
55.4269783207937));
#174412=CARTESIAN_POINT('Ctrl Pts',(72.6687597765691,-11.1043081293031,
56.7097351294882));
#174413=CARTESIAN_POINT('Ctrl Pts',(64.9259843066721,-7.847893694807,57.9924919381828));
#174414=CARTESIAN_POINT('Ctrl Pts',(61.704933210124,-9.31546506599545E-15,
58.477946740529));
#174415=CARTESIAN_POINT('Ctrl Pts',(64.8977664778012,7.84789369480699,57.8324606783183));
#174416=CARTESIAN_POINT('Ctrl Pts',(72.6123241188273,11.1043081293031,56.3896726097593));
#174417=CARTESIAN_POINT('Ctrl Pts',(80.3268817598535,7.847893694807,54.9468845412002));
#174418=CARTESIAN_POINT('Ctrl Pts',(83.5197150275307,9.33628174770718E-15,
54.3013984789895));
#174419=CARTESIAN_POINT('Ctrl Pts',(80.2986639309826,-7.84789369480698,
54.7868532813357));
#174420=CARTESIAN_POINT('Ctrl Pts',(72.5558884610856,-11.1043081293031,
56.0696100900303));
#174421=CARTESIAN_POINT('Ctrl Pts',(64.8131129911886,-7.847893694807,57.3523668987248));
#174422=CARTESIAN_POINT('Ctrl Pts',(61.5920618946405,-1.24240895349459E-14,
57.8378217010711));
#174423=CARTESIAN_POINT('Ctrl Pts',(64.7848951623178,7.84789369480698,57.1923356388604));
#174424=CARTESIAN_POINT('Ctrl Pts',(72.4994528033438,11.1043081293031,55.7495475703013));
#174425=CARTESIAN_POINT('Ctrl Pts',(80.21401044437,7.847893694807,54.3067595017423));
#174426=CARTESIAN_POINT('Ctrl Pts',(83.4068437120472,1.04083408558608E-17,
53.6612734395316));
#174427=CARTESIAN_POINT('Ctrl Pts',(80.1857926154992,-7.84789369480693,
54.1467282418778));
#174428=CARTESIAN_POINT('Ctrl Pts',(72.4430171456021,-11.1043081293031,
55.4294850505724));
#174429=CARTESIAN_POINT('Ctrl Pts',(64.7002416757051,-7.84789369480699,
56.7122418592669));
#174430=CARTESIAN_POINT('Ctrl Pts',(61.479190579157,-7.81492925927552E-14,
57.1976966616131));
#174431=CARTESIAN_POINT('Ctrl Pts',(64.6720238468343,7.847893694807,56.5522105994024));
#174432=CARTESIAN_POINT('Ctrl Pts',(72.3865814878603,11.1043081293031,55.1094225308434));
#174433=CARTESIAN_POINT('Ctrl Pts',(80.1011391288866,7.84789369480695,53.6666344622843));
#174434=CARTESIAN_POINT('Ctrl Pts',(83.2939723965637,1.5109441475758E-14,
53.0211484000736));
#174435=CARTESIAN_POINT('Ctrl Pts',(80.0729213000157,-7.84789369480693,
53.5066032024198));
#174436=CARTESIAN_POINT('Ctrl Pts',(72.3301458301186,-11.1043081293031,
54.7893600111144));
#174437=CARTESIAN_POINT('Ctrl Pts',(64.5873703602217,-7.84789369480702,
56.072116819809));
#174438=CARTESIAN_POINT('Ctrl Pts',(61.3663192636735,4.44193293258621E-14,
56.5575716221552));
#174439=CARTESIAN_POINT('Ctrl Pts',(64.5591525313508,7.84789369480696,55.9120855599445));
#174440=CARTESIAN_POINT('Ctrl Pts',(72.2737101723769,11.1043081293031,54.4692974913855));
#174441=CARTESIAN_POINT('Ctrl Pts',(79.9882678134031,7.84789369480695,53.0265094228264));
#174442=CARTESIAN_POINT('Ctrl Pts',(83.1811010810802,1.77739767348584E-14,
52.3810233606157));
#174443=CARTESIAN_POINT('Ctrl Pts',(79.9600499845322,-7.84789369480693,
52.8664781629619));
#174444=CARTESIAN_POINT('Ctrl Pts',(72.2172745146351,-11.1043081293031,
54.1492349716565));
#174445=CARTESIAN_POINT('Ctrl Pts',(64.4744990447382,-7.84789369480699,
55.431991780351));
#174446=CARTESIAN_POINT('Ctrl Pts',(61.2534479481901,-8.21460954814057E-14,
55.9174465826972));
#174447=CARTESIAN_POINT('Ctrl Pts',(64.4462812158673,7.847893694807,55.2719605204866));
#174448=CARTESIAN_POINT('Ctrl Pts',(72.1608388568933,11.1043081293031,53.8291724519275));
#174449=CARTESIAN_POINT('Ctrl Pts',(79.8753964979196,7.84789369480696,52.3863843833685));
#174450=CARTESIAN_POINT('Ctrl Pts',(83.0682297655968,2.04385119939587E-14,
51.7408983211578));
#174451=CARTESIAN_POINT('Ctrl Pts',(79.8471786690487,-7.84789369480692,
52.226353123504));
#174452=CARTESIAN_POINT('Ctrl Pts',(72.1044031991516,-11.1043081293031,
53.5091099321985));
#174453=CARTESIAN_POINT('Ctrl Pts',(64.3616277292547,-7.84789369480703,
54.7918667408931));
#174454=CARTESIAN_POINT('Ctrl Pts',(61.1405766327066,3.95343480175114E-14,
55.2773215432393));
#174455=CARTESIAN_POINT('Ctrl Pts',(64.3334099003838,7.84789369480696,54.6318354810286));
#174456=CARTESIAN_POINT('Ctrl Pts',(72.0479675414099,11.1043081293031,53.1890474124696));
#174457=CARTESIAN_POINT('Ctrl Pts',(79.7625251824361,7.84789369480696,51.7462593439105));
#174458=CARTESIAN_POINT('Ctrl Pts',(82.9553584501133,2.39912256727592E-14,
51.1007732816998));
#174459=CARTESIAN_POINT('Ctrl Pts',(79.8532683905412,-7.55805241504216,
51.568299089764));
#174460=CARTESIAN_POINT('Ctrl Pts',(75.1351236247948,-9.76890830967669,
52.3482800822328));
#174461=CARTESIAN_POINT('Ctrl Pts',(72.8483838954811,-9.97929647052207,
52.7270399031534));
#174462=CARTESIAN_POINT('Ctrl Pts',(83.0141466356044,-4.33680868994202E-16,
57.6851587580378));
#174463=CARTESIAN_POINT('Ctrl Pts',(83.0094436641259,-2.62292530172754,
57.6584868813937));
#174464=CARTESIAN_POINT('Ctrl Pts',(80.8620762664272,-7.84789369480698,
57.9821234162912));
#174465=CARTESIAN_POINT('Ctrl Pts',(73.1193007965301,-11.1043081293031,
59.2648802249857));
#174466=CARTESIAN_POINT('Ctrl Pts',(65.3765253266331,-7.84789369480698,
60.5476370336803));
#174467=CARTESIAN_POINT('Ctrl Pts',(62.155474230085,-2.21003770839445E-15,
61.0330918360265));
#174468=CARTESIAN_POINT('Ctrl Pts',(65.3483074977623,7.84789369480698,60.3876057738158));
#174469=CARTESIAN_POINT('Ctrl Pts',(73.0628651387884,11.1043081293031,58.9448177052568));
#174470=CARTESIAN_POINT('Ctrl Pts',(80.7774227798145,7.84789369480698,57.5020296366977));
#174471=CARTESIAN_POINT('Ctrl Pts',(83.9702560474918,1.78676518025611E-15,
56.856543574487));
#174472=CARTESIAN_POINT('Ctrl Pts',(80.7492049509437,-7.84789369480698,
57.3419983768332));
#174473=CARTESIAN_POINT('Ctrl Pts',(73.0064294810467,-11.1043081293031,
58.6247551855278));
#174474=CARTESIAN_POINT('Ctrl Pts',(65.2636540111497,-7.847893694807,59.9075119942224));
#174475=CARTESIAN_POINT('Ctrl Pts',(62.0426029146016,-3.54230533794464E-15,
60.3929667965686));
#174476=CARTESIAN_POINT('Ctrl Pts',(65.2354361822788,7.84789369480699,59.7474807343579));
#174477=CARTESIAN_POINT('Ctrl Pts',(72.9499938233049,11.1043081293031,58.3046926657988));
#174478=CARTESIAN_POINT('Ctrl Pts',(80.664551464331,7.847893694807,56.8619045972398));
#174479=CARTESIAN_POINT('Ctrl Pts',(83.8573847320083,5.33947885905661E-15,
56.2164185350291));
#174480=CARTESIAN_POINT('Ctrl Pts',(80.6363336354602,-7.84789369480699,
56.7018733373753));
#174481=CARTESIAN_POINT('Ctrl Pts',(72.8935581655632,-11.1043081293031,
57.9846301460699));
#174482=CARTESIAN_POINT('Ctrl Pts',(65.1507826956662,-7.847893694807,59.2673869547644));
#174483=CARTESIAN_POINT('Ctrl Pts',(61.9297315991181,-7.5391082265952E-15,
59.7528417571106));
#174484=CARTESIAN_POINT('Ctrl Pts',(65.1225648667953,7.84789369480699,59.1073556948999));
#174485=CARTESIAN_POINT('Ctrl Pts',(72.8371225078214,11.1043081293031,57.6645676263409));
#174486=CARTESIAN_POINT('Ctrl Pts',(80.5516801488476,7.84789369480699,56.2217795577819));
#174487=CARTESIAN_POINT('Ctrl Pts',(83.7445134165248,7.11583569845686E-15,
55.5762934955712));
#174488=CARTESIAN_POINT('Ctrl Pts',(80.5234623199767,-7.84789369480698,
56.0617482979174));
#174489=CARTESIAN_POINT('Ctrl Pts',(72.7806868500797,-11.1043081293031,
57.3445051066119));
#174490=CARTESIAN_POINT('Ctrl Pts',(65.0379113801827,-7.847893694807,58.6272619153065));
#174491=CARTESIAN_POINT('Ctrl Pts',(61.8168602836346,-9.31546506599545E-15,
59.1127167176527));
#174492=CARTESIAN_POINT('Ctrl Pts',(65.0096935513118,7.84789369480699,58.467230655442));
#174493=CARTESIAN_POINT('Ctrl Pts',(72.7242511923379,11.1043081293031,57.024442586883));
#174494=CARTESIAN_POINT('Ctrl Pts',(80.4388088333641,7.847893694807,55.5816545183239));
#174495=CARTESIAN_POINT('Ctrl Pts',(83.6316421010413,9.33628174770718E-15,
54.9361684561132));
#174496=CARTESIAN_POINT('Ctrl Pts',(80.4105910044932,-7.84789369480698,
55.4216232584594));
#174497=CARTESIAN_POINT('Ctrl Pts',(72.6678155345962,-11.1043081293031,
56.704380067154));
#174498=CARTESIAN_POINT('Ctrl Pts',(64.9250400646992,-7.847893694807,57.9871368758485));
#174499=CARTESIAN_POINT('Ctrl Pts',(61.7039889681511,-1.24240895349459E-14,
58.4725916781948));
#174500=CARTESIAN_POINT('Ctrl Pts',(64.8968222358283,7.84789369480698,57.8271056159841));
#174501=CARTESIAN_POINT('Ctrl Pts',(72.6113798768544,11.1043081293031,56.384317547425));
#174502=CARTESIAN_POINT('Ctrl Pts',(80.3259375178806,7.847893694807,54.941529478866));
#174503=CARTESIAN_POINT('Ctrl Pts',(83.5187707855578,1.04083408558608E-17,
54.2960434166553));
#174504=CARTESIAN_POINT('Ctrl Pts',(80.2977196890098,-7.84789369480693,
54.7814982190015));
#174505=CARTESIAN_POINT('Ctrl Pts',(72.5549442191127,-11.1043081293031,
56.0642550276961));
#174506=CARTESIAN_POINT('Ctrl Pts',(64.8121687492157,-7.84789369480699,
57.3470118363906));
#174507=CARTESIAN_POINT('Ctrl Pts',(61.5911176526676,-7.81492925927552E-14,
57.8324666387368));
#174508=CARTESIAN_POINT('Ctrl Pts',(64.7839509203449,7.847893694807,57.1869805765261));
#174509=CARTESIAN_POINT('Ctrl Pts',(72.4985085613709,11.1043081293031,55.7441925079671));
#174510=CARTESIAN_POINT('Ctrl Pts',(80.2130662023972,7.84789369480695,54.301404439408));
#174511=CARTESIAN_POINT('Ctrl Pts',(83.4058994700743,1.5109441475758E-14,
53.6559183771974));
#174512=CARTESIAN_POINT('Ctrl Pts',(80.1848483735263,-7.84789369480693,
54.1413731795435));
#174513=CARTESIAN_POINT('Ctrl Pts',(72.4420729036292,-11.1043081293031,
55.4241299882381));
#174514=CARTESIAN_POINT('Ctrl Pts',(64.6992974337323,-7.84789369480702,
56.7068867969327));
#174515=CARTESIAN_POINT('Ctrl Pts',(61.4782463371841,4.44193293258621E-14,
57.1923415992789));
#174516=CARTESIAN_POINT('Ctrl Pts',(64.6710796048613,7.84789369480696,56.5468555370682));
#174517=CARTESIAN_POINT('Ctrl Pts',(72.3856372458874,11.1043081293031,55.1040674685092));
#174518=CARTESIAN_POINT('Ctrl Pts',(80.1001948869137,7.84789369480695,53.6612793999501));
#174519=CARTESIAN_POINT('Ctrl Pts',(83.2930281545908,1.77739767348584E-14,
53.0157933377394));
#174520=CARTESIAN_POINT('Ctrl Pts',(80.0719770580428,-7.84789369480693,
53.5012481400856));
#174521=CARTESIAN_POINT('Ctrl Pts',(72.3292015881457,-11.1043081293031,
54.7840049487802));
#174522=CARTESIAN_POINT('Ctrl Pts',(64.5864261182488,-7.84789369480699,
56.0667617574747));
#174523=CARTESIAN_POINT('Ctrl Pts',(61.3653750217006,-8.21460954814057E-14,
56.5522165598209));
#174524=CARTESIAN_POINT('Ctrl Pts',(64.5582082893779,7.847893694807,55.9067304976102));
#174525=CARTESIAN_POINT('Ctrl Pts',(72.2727659304039,11.1043081293031,54.4639424290512));
#174526=CARTESIAN_POINT('Ctrl Pts',(79.9873235714302,7.84789369480696,53.0211543604921));
#174527=CARTESIAN_POINT('Ctrl Pts',(83.1801568391073,2.04385119939587E-14,
52.3756682982815));
#174528=CARTESIAN_POINT('Ctrl Pts',(79.9591057425593,-7.84789369480692,
52.8611231006277));
#174529=CARTESIAN_POINT('Ctrl Pts',(72.2163302726622,-11.1043081293031,
54.1438799093222));
#174530=CARTESIAN_POINT('Ctrl Pts',(64.4735548027653,-7.84789369480703,
55.4266367180168));
#174531=CARTESIAN_POINT('Ctrl Pts',(61.2525037062171,3.95343480175114E-14,
55.912091520363));
#174532=CARTESIAN_POINT('Ctrl Pts',(64.4453369738944,7.84789369480696,55.2666054581523));
#174533=CARTESIAN_POINT('Ctrl Pts',(72.1598946149204,11.1043081293031,53.8238173895933));
#174534=CARTESIAN_POINT('Ctrl Pts',(79.8744522559467,7.84789369480696,52.3810293210342));
#174535=CARTESIAN_POINT('Ctrl Pts',(83.0672855236239,2.39912256727592E-14,
51.7355432588235));
#174536=CARTESIAN_POINT('Ctrl Pts',(79.9651954640518,-7.55805241504216,
52.2030690668877));
#174537=CARTESIAN_POINT('Ctrl Pts',(75.2470506983054,-9.76890830967669,
52.9830500593565));
#174538=CARTESIAN_POINT('Ctrl Pts',(72.9603109689917,-9.97929647052207,
53.3618098802771));
#174539=CARTESIAN_POINT('Ctrl Pts',(82.420455096836,-4.33680868994202E-16,
57.4690727095904));
#174540=CARTESIAN_POINT('Ctrl Pts',(82.4157521253576,-2.47968200709192,
57.4424008329463));
#174541=CARTESIAN_POINT('Ctrl Pts',(80.3851431585526,-7.41930423095383,
57.745449706252));
#174542=CARTESIAN_POINT('Ctrl Pts',(73.0644459155175,-10.4978792386127,
58.9537827355813));
#174543=CARTESIAN_POINT('Ctrl Pts',(65.7437486724824,-7.41930423095383,
60.1621157649105));
#174544=CARTESIAN_POINT('Ctrl Pts',(62.6978352222749,-2.21003770839445E-15,
60.6166890748691));
#174545=CARTESIAN_POINT('Ctrl Pts',(65.7155308436115,7.41930423095382,60.002084505046));
#174546=CARTESIAN_POINT('Ctrl Pts',(73.0080102577757,10.4978792386127,58.6337202158523));
#174547=CARTESIAN_POINT('Ctrl Pts',(80.30048967194,7.41930423095383,57.2653559266586));
#174548=CARTESIAN_POINT('Ctrl Pts',(83.3181852932766,1.78676518025611E-15,
56.6507513568355));
#174549=CARTESIAN_POINT('Ctrl Pts',(80.2722718430691,-7.41930423095382,
57.1053246667941));
#174550=CARTESIAN_POINT('Ctrl Pts',(72.951574600034,-10.4978792386127,58.3136576961233));
#174551=CARTESIAN_POINT('Ctrl Pts',(65.6308773569989,-7.41930423095384,
59.5219907254526));
#174552=CARTESIAN_POINT('Ctrl Pts',(62.5849639067914,-3.54230533794464E-15,
59.9765640354111));
#174553=CARTESIAN_POINT('Ctrl Pts',(65.6026595281281,7.41930423095383,59.3619594655881));
#174554=CARTESIAN_POINT('Ctrl Pts',(72.8951389422923,10.4978792386127,57.9935951763944));
#174555=CARTESIAN_POINT('Ctrl Pts',(80.1876183564565,7.41930423095384,56.6252308872007));
#174556=CARTESIAN_POINT('Ctrl Pts',(83.2053139777931,5.33947885905661E-15,
56.0106263173776));
#174557=CARTESIAN_POINT('Ctrl Pts',(80.1594005275856,-7.41930423095383,
56.4651996273362));
#174558=CARTESIAN_POINT('Ctrl Pts',(72.8387032845505,-10.4978792386127,
57.6735326566654));
#174559=CARTESIAN_POINT('Ctrl Pts',(65.5180060415154,-7.41930423095384,
58.8818656859946));
#174560=CARTESIAN_POINT('Ctrl Pts',(62.4720925913079,-7.5391082265952E-15,
59.3364389959532));
#174561=CARTESIAN_POINT('Ctrl Pts',(65.4897882126446,7.41930423095383,58.7218344261301));
#174562=CARTESIAN_POINT('Ctrl Pts',(72.7822676268087,10.4978792386127,57.3534701369364));
#174563=CARTESIAN_POINT('Ctrl Pts',(80.074747040973,7.41930423095384,55.9851058477427));
#174564=CARTESIAN_POINT('Ctrl Pts',(83.0924426623096,7.11583569845686E-15,
55.3705012779196));
#174565=CARTESIAN_POINT('Ctrl Pts',(80.0465292121021,-7.41930423095383,
55.8250745878782));
#174566=CARTESIAN_POINT('Ctrl Pts',(72.725831969067,-10.4978792386127,57.0334076172075));
#174567=CARTESIAN_POINT('Ctrl Pts',(65.405134726032,-7.41930423095385,58.2417406465367));
#174568=CARTESIAN_POINT('Ctrl Pts',(62.3592212758244,-9.31546506599545E-15,
58.6963139564953));
#174569=CARTESIAN_POINT('Ctrl Pts',(65.3769168971611,7.41930423095384,58.0817093866722));
#174570=CARTESIAN_POINT('Ctrl Pts',(72.6693963113252,10.4978792386127,56.7133450974785));
#174571=CARTESIAN_POINT('Ctrl Pts',(79.9618757254895,7.41930423095385,55.3449808082848));
#174572=CARTESIAN_POINT('Ctrl Pts',(82.9795713468261,9.33628174770718E-15,
54.7303762384617));
#174573=CARTESIAN_POINT('Ctrl Pts',(79.9336578966186,-7.41930423095383,
55.1849495484203));
#174574=CARTESIAN_POINT('Ctrl Pts',(72.6129606535835,-10.4978792386127,
56.3932825777495));
#174575=CARTESIAN_POINT('Ctrl Pts',(65.2922634105485,-7.41930423095385,
57.6016156070787));
#174576=CARTESIAN_POINT('Ctrl Pts',(62.246349960341,-1.24240895349459E-14,
58.0561889170373));
#174577=CARTESIAN_POINT('Ctrl Pts',(65.2640455816776,7.41930423095383,57.4415843472143));
#174578=CARTESIAN_POINT('Ctrl Pts',(72.5565249958418,10.4978792386127,56.0732200580206));
#174579=CARTESIAN_POINT('Ctrl Pts',(79.849004410006,7.41930423095385,54.7048557688268));
#174580=CARTESIAN_POINT('Ctrl Pts',(82.8667000313426,1.04083408558608E-17,
54.0902511990038));
#174581=CARTESIAN_POINT('Ctrl Pts',(79.8207865811352,-7.41930423095378,
54.5448245089623));
#174582=CARTESIAN_POINT('Ctrl Pts',(72.5000893381,-10.4978792386127,55.7531575382916));
#174583=CARTESIAN_POINT('Ctrl Pts',(65.179392095065,-7.41930423095383,56.9614905676208));
#174584=CARTESIAN_POINT('Ctrl Pts',(62.1334786448575,-7.81492925927552E-14,
57.4160638775794));
#174585=CARTESIAN_POINT('Ctrl Pts',(65.1511742661941,7.41930423095385,56.8014593077563));
#174586=CARTESIAN_POINT('Ctrl Pts',(72.4436536803583,10.4978792386127,55.4330950185626));
#174587=CARTESIAN_POINT('Ctrl Pts',(79.7361330945226,7.4193042309538,54.0647307293689));
#174588=CARTESIAN_POINT('Ctrl Pts',(82.7538287158591,1.5109441475758E-14,
53.4501261595458));
#174589=CARTESIAN_POINT('Ctrl Pts',(79.7079152656517,-7.41930423095378,
53.9046994695044));
#174590=CARTESIAN_POINT('Ctrl Pts',(72.3872180226165,-10.4978792386127,
55.1130324988336));
#174591=CARTESIAN_POINT('Ctrl Pts',(65.0665207795815,-7.41930423095387,
56.3213655281629));
#174592=CARTESIAN_POINT('Ctrl Pts',(62.020607329374,4.44193293258621E-14,
56.7759388381215));
#174593=CARTESIAN_POINT('Ctrl Pts',(65.0383029507106,7.41930423095381,56.1613342682984));
#174594=CARTESIAN_POINT('Ctrl Pts',(72.3307823648748,10.4978792386127,54.7929699791047));
#174595=CARTESIAN_POINT('Ctrl Pts',(79.6232617790391,7.4193042309538,53.424605689911));
#174596=CARTESIAN_POINT('Ctrl Pts',(82.6409574003756,1.77739767348584E-14,
52.8100011200879));
#174597=CARTESIAN_POINT('Ctrl Pts',(79.5950439501682,-7.41930423095377,
53.2645744300465));
#174598=CARTESIAN_POINT('Ctrl Pts',(72.2743467071331,-10.4978792386127,
54.4729074593757));
#174599=CARTESIAN_POINT('Ctrl Pts',(64.953649464098,-7.41930423095384,55.6812404887049));
#174600=CARTESIAN_POINT('Ctrl Pts',(61.9077360138905,-8.21460954814057E-14,
56.1358137986635));
#174601=CARTESIAN_POINT('Ctrl Pts',(64.9254316352271,7.41930423095385,55.5212092288404));
#174602=CARTESIAN_POINT('Ctrl Pts',(72.2179110493913,10.4978792386127,54.1528449396467));
#174603=CARTESIAN_POINT('Ctrl Pts',(79.5103904635556,7.41930423095381,52.784480650453));
#174604=CARTESIAN_POINT('Ctrl Pts',(82.5280860848922,2.04385119939587E-14,
52.1698760806299));
#174605=CARTESIAN_POINT('Ctrl Pts',(79.4821726346847,-7.41930423095377,
52.6244493905885));
#174606=CARTESIAN_POINT('Ctrl Pts',(72.1614753916496,-10.4978792386127,
53.8327824199178));
#174607=CARTESIAN_POINT('Ctrl Pts',(64.8407781486145,-7.41930423095387,
55.041115449247));
#174608=CARTESIAN_POINT('Ctrl Pts',(61.794864698407,3.95343480175114E-14,
55.4956887592056));
#174609=CARTESIAN_POINT('Ctrl Pts',(64.8125603197436,7.41930423095381,54.8810841893825));
#174610=CARTESIAN_POINT('Ctrl Pts',(72.1050397339078,10.4978792386127,53.5127199001888));
#174611=CARTESIAN_POINT('Ctrl Pts',(79.3975191480721,7.4193042309538,52.1443556109951));
#174612=CARTESIAN_POINT('Ctrl Pts',(82.4152147694087,2.39912256727592E-14,
51.529751041172));
#174613=CARTESIAN_POINT('Ctrl Pts',(79.481794108578,-7.14529177399519,51.9675358834182));
#174614=CARTESIAN_POINT('Ctrl Pts',(75.0208316204567,-9.23540832385942,
52.7021687013817));
#174615=CARTESIAN_POINT('Ctrl Pts',(72.858747024875,-9.43430675859939,53.0589484589415));
#174616=CARTESIAN_POINT('Origin',(71.9970151052421,-5.75,67.2970079954268));
#174617=CARTESIAN_POINT('',(69.479116529072,-5.75,53.0172955767497));
#174618=CARTESIAN_POINT('',(69.479116529072,-1.27999799280051E-15,53.0172955767497));
#174619=CARTESIAN_POINT('',(69.0102664493713,-5.75,50.3583146436167));
#174620=CARTESIAN_POINT('',(71.9970151052421,-5.75,67.2970079954268));
#174621=CARTESIAN_POINT('',(69.0102664493713,4.54725483176297E-16,50.3583146436167));
#174622=CARTESIAN_POINT('Origin',(76.9210538703031,-5.75,66.4287671070923));
#174623=CARTESIAN_POINT('',(74.403155294133,-5.75,52.1490546884152));
#174624=CARTESIAN_POINT('',(71.9411359116025,-5.75,52.5831751325825));
#174625=CARTESIAN_POINT('',(73.9343052144324,-5.75,49.4900737552822));
#174626=CARTESIAN_POINT('',(76.9210538703031,-5.75,66.4287671070923));
#174627=CARTESIAN_POINT('',(71.4722858319019,-5.75,49.9241941994495));
#174628=CARTESIAN_POINT('Origin',(76.9210538703031,-3.1224989991992,66.4287671070923));
#174629=CARTESIAN_POINT('',(74.403155294133,-3.1224989991992,52.1490546884152));
#174630=CARTESIAN_POINT('',(74.403155294133,3.70547026447916E-16,52.1490546884152));
#174631=CARTESIAN_POINT('',(73.9343052144324,-3.1224989991992,49.4900737552822));
#174632=CARTESIAN_POINT('',(76.9210538703031,-3.1224989991992,66.4287671070923));
#174633=CARTESIAN_POINT('',(73.9343052144324,2.10527050242472E-15,49.4900737552822));
#174634=CARTESIAN_POINT('Origin',(74.4590344877726,0.,66.8628875512595));
#174635=CARTESIAN_POINT('',(74.403155294133,3.1224989991992,52.1490546884152));
#174636=CARTESIAN_POINT('Origin',(71.9411359116025,0.,52.5831751325825));
#174637=CARTESIAN_POINT('',(73.9343052144324,3.1224989991992,49.4900737552822));
#174638=CARTESIAN_POINT('',(76.9210538703031,3.1224989991992,66.4287671070923));
#174639=CARTESIAN_POINT('Origin',(71.4722858319019,0.,49.9241941994495));
#174640=CARTESIAN_POINT('Origin',(76.9210538703031,5.75,66.4287671070923));
#174641=CARTESIAN_POINT('',(74.403155294133,5.75,52.1490546884152));
#174642=CARTESIAN_POINT('',(74.403155294133,3.70547026447918E-16,52.1490546884152));
#174643=CARTESIAN_POINT('',(73.9343052144324,5.75,49.4900737552822));
#174644=CARTESIAN_POINT('',(76.9210538703031,5.75,66.4287671070923));
#174645=CARTESIAN_POINT('',(73.9343052144324,2.10527050242472E-15,49.4900737552822));
#174646=CARTESIAN_POINT('Origin',(71.997015105242,5.75,67.2970079954268));
#174647=CARTESIAN_POINT('',(69.479116529072,5.75,53.0172955767497));
#174648=CARTESIAN_POINT('',(71.9411359116025,5.75,52.5831751325825));
#174649=CARTESIAN_POINT('',(69.0102664493713,5.75,50.3583146436167));
#174650=CARTESIAN_POINT('',(71.997015105242,5.75,67.2970079954268));
#174651=CARTESIAN_POINT('',(71.4722858319019,5.75,49.9241941994495));
#174652=CARTESIAN_POINT('Origin',(71.997015105242,3.1224989991992,67.2970079954268));
#174653=CARTESIAN_POINT('',(69.479116529072,-1.27999799280051E-15,53.0172955767497));
#174654=CARTESIAN_POINT('',(69.0102664493713,4.54725483176297E-16,50.3583146436167));
#174655=CARTESIAN_POINT('Origin',(71.9411359116025,-8.67361737988404E-16,
52.5831751325825));
#174656=CARTESIAN_POINT('Origin',(72.7225527111036,-4.33680868994202E-16,
57.0148100211374));
#174657=CARTESIAN_POINT('Origin',(71.4722858319019,8.67361737988404E-16,
49.9241941994495));
#174658=CARTESIAN_POINT('',(68.0608117040921,6.,50.5257291321711));
#174659=CARTESIAN_POINT('',(64.6493375762823,1.47451495458029E-14,51.1272640648928));
#174660=CARTESIAN_POINT('',(68.0608117040921,6.,50.5257291321711));
#174661=CARTESIAN_POINT('',(74.8837599597117,6.,49.3226592667278));
#174662=CARTESIAN_POINT('',(74.8837599597117,6.,49.3226592667278));
#174663=CARTESIAN_POINT('',(78.2952340875215,0.,48.7211243340062));
#174664=CARTESIAN_POINT('',(78.2952340875215,0.,48.7211243340062));
#174665=CARTESIAN_POINT('',(74.8837599597116,-6.,49.3226592667279));
#174666=CARTESIAN_POINT('',(74.8837599597116,-6.,49.3226592667279));
#174667=CARTESIAN_POINT('',(68.0608117040921,-6.,50.5257291321711));
#174668=CARTESIAN_POINT('',(68.0608117040921,-6.,50.5257291321711));
#174669=CARTESIAN_POINT('',(64.6493375762823,1.59872115546023E-14,51.1272640648928));
#174670=CARTESIAN_POINT('Origin',(74.8837599597116,-6.,49.3226592667279));
#174671=CARTESIAN_POINT('',(78.2952340875215,0.,48.7211243340062));
#174672=CARTESIAN_POINT('',(74.8837599597116,-6.,49.3226592667279));
#174673=CARTESIAN_POINT('Origin',(68.0608117040921,-6.,50.5257291321711));
#174674=CARTESIAN_POINT('',(68.0608117040921,-6.,50.5257291321711));
#174675=CARTESIAN_POINT('Origin',(64.6493375762823,1.59872115546023E-14,
51.1272640648928));
#174676=CARTESIAN_POINT('',(64.6493375762823,1.47451495458029E-14,51.1272640648928));
#174677=CARTESIAN_POINT('Origin',(68.0608117040921,6.,50.5257291321711));
#174678=CARTESIAN_POINT('',(68.0608117040921,6.,50.5257291321711));
#174679=CARTESIAN_POINT('Origin',(74.8837599597117,6.,49.3226592667278));
#174680=CARTESIAN_POINT('',(74.8837599597117,6.,49.3226592667278));
#174681=CARTESIAN_POINT('Origin',(78.2952340875215,0.,48.7211243340062));
#174682=CARTESIAN_POINT('Origin',(73.035119430904,-4.33680868994202E-16,
58.7874639765594));
#174683=CARTESIAN_POINT('Origin',(71.5591099207353,0.,50.4165980759556));
#174684=CARTESIAN_POINT('Origin',(71.9064062760691,0.,52.38621358198));
#174685=CARTESIAN_POINT('Origin',(69.7358040552328,0.,40.0761166693274));
#221636=UNCERTAINTY_MEASURE_WITH_UNIT(LENGTH_MEASURE(0.01),#221663,
'DISTANCE_ACCURACY_VALUE',
'Maximum model space distance between geometric entities at asserted c
onnectivities');
#221647=UNCERTAINTY_MEASURE_WITH_UNIT(LENGTH_MEASURE(0.01),#221663,
'DISTANCE_ACCURACY_VALUE',
'Maximum model space distance between geometric entities at asserted c
onnectivities');
#221651=(
GEOMETRIC_REPRESENTATION_CONTEXT(3)
GLOBAL_UNCERTAINTY_ASSIGNED_CONTEXT((#221636))
GLOBAL_UNIT_ASSIGNED_CONTEXT((#221663,#221665,#221666))
REPRESENTATION_CONTEXT('','3D')
);
#221662=(
GEOMETRIC_REPRESENTATION_CONTEXT(3)
GLOBAL_UNCERTAINTY_ASSIGNED_CONTEXT((#221647))
GLOBAL_UNIT_ASSIGNED_CONTEXT((#221663,#221665,#221666))
REPRESENTATION_CONTEXT('','3D')
);
#221663=(
LENGTH_UNIT()
NAMED_UNIT(*)
SI_UNIT(.MILLI.,.METRE.)
);
#221665=(
NAMED_UNIT(*)
PLANE_ANGLE_UNIT()
SI_UNIT($,.RADIAN.)
);
#221666=(
NAMED_UNIT(*)
SI_UNIT($,.STERADIAN.)
SOLID_ANGLE_UNIT()
);
#221670=SHAPE_DEFINITION_REPRESENTATION(#221684,#221711);
#221684=PRODUCT_DEFINITION_SHAPE('',$,#221726);
#221711=SHAPE_REPRESENTATION('',(#80522),#221651);
#221722=PRODUCT_DEFINITION_CONTEXT('part definition',#221766,'design');
#221726=PRODUCT_DEFINITION('2026-10-05-23-02-30-143',
'Shower Hose Connector',#221740,#221722);
#221740=PRODUCT_DEFINITION_FORMATION('',$,#221771);
#221766=APPLICATION_CONTEXT(
'Core Data for Automotive Mechanical Design Process');
#221767=PRODUCT_CONTEXT('part definition',#221766,'mechanical');
#221771=PRODUCT('2026-10-05-23-02-30-143','Shower Hose Connector',$,(#221767));
#221783=PRESENTATION_STYLE_ASSIGNMENT((#221785));
#221785=SURFACE_STYLE_USAGE(.BOTH.,#221787);
#221787=SURFACE_SIDE_STYLE('',(#221789));
#221789=SURFACE_STYLE_FILL_AREA(#221791);
#221791=FILL_AREA_STYLE('Opaque(202,209,238)',(#221793));
#221793=FILL_AREA_STYLE_COLOUR('Opaque(202,209,238)',#221795);
#221795=COLOUR_RGB('Opaque(202,209,238)', 0.09019608, 0.27058824, 0.51372549);
ENDSEC;
END-ISO-10303-21;
